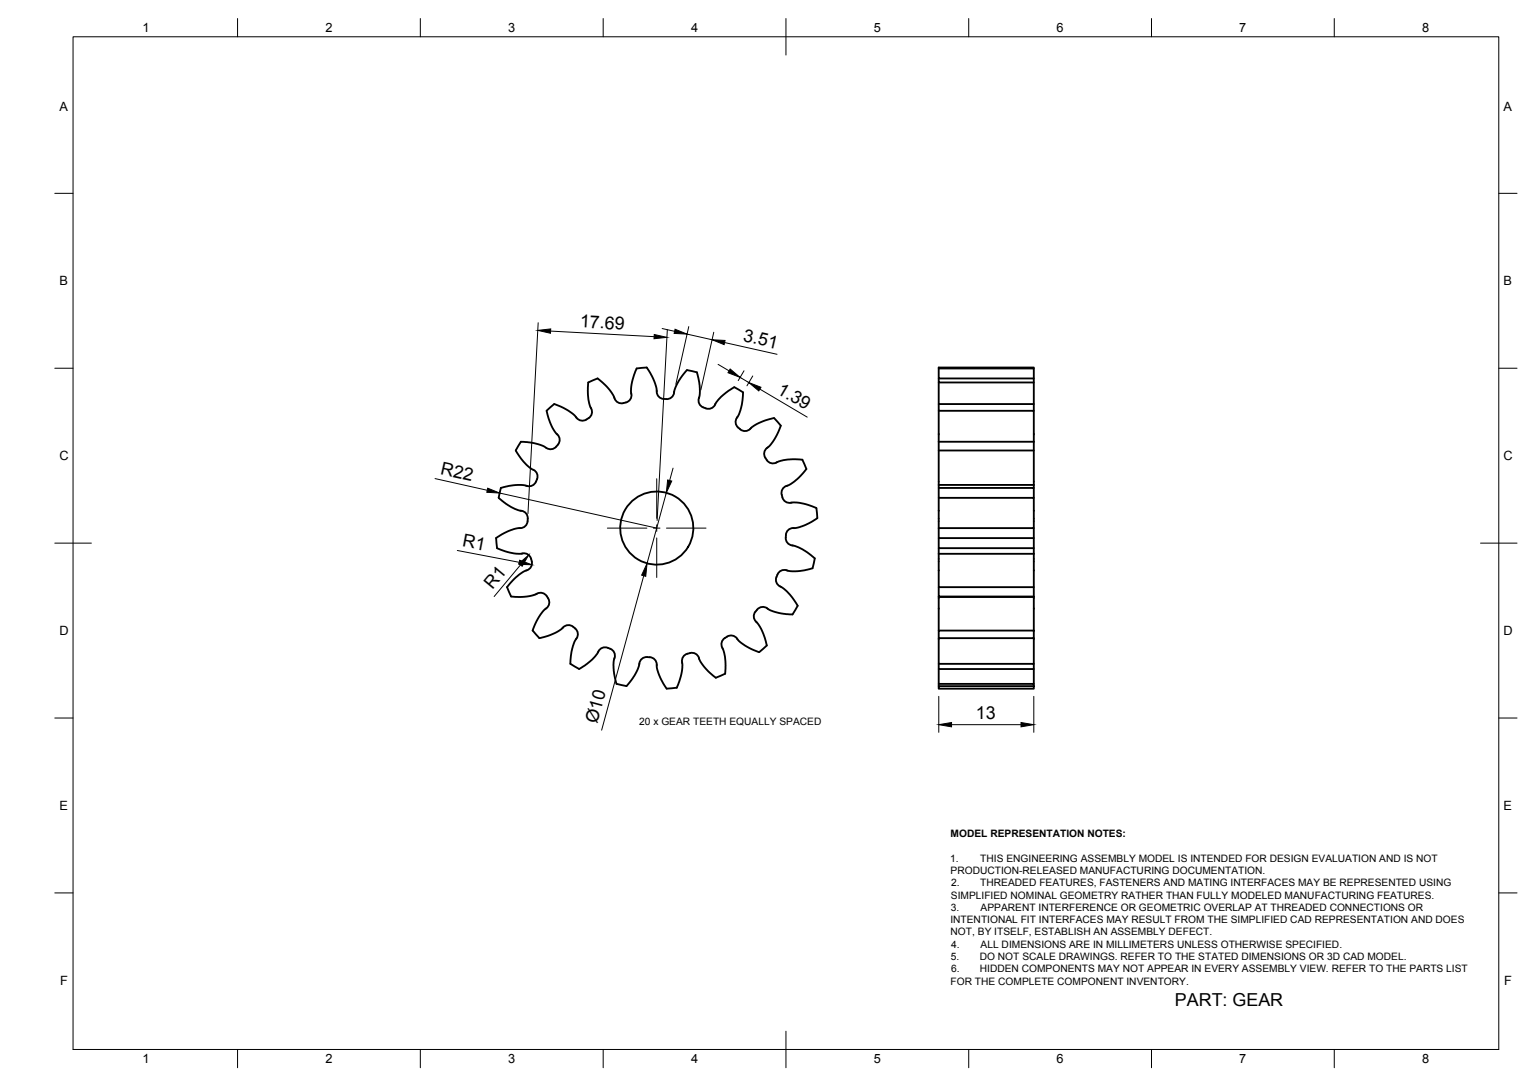
ISO-10303-21;
HEADER;
/* Generated by software containing ST-Developer
 * from STEP Tools, Inc. (www.steptools.com) 
 */

FILE_DESCRIPTION(
/* description */ (''),
/* implementation_level */ '2;1');

FILE_NAME(
/* name */ 'Gear.step',
/* time_stamp */ '2026-10-04T22:47:03-07:00',
/* author */ (''),
/* organization */ (''),
/* preprocessor_version */ 'ST-DEVELOPER v20.2',
/* originating_system */ 'Autodesk Translation Framework v15.15.0.0',
/* authorisation */ '');

FILE_SCHEMA (('AUTOMOTIVE_DESIGN { 1 0 10303 214 3 1 1 }'));
ENDSEC;

DATA;
#10=MECHANICAL_DESIGN_GEOMETRIC_PRESENTATION_REPRESENTATION('',(#77),#19878);
#63=SHAPE_REPRESENTATION_RELATIONSHIP('SRR','None',#19907,#70);
#70=ADVANCED_BREP_SHAPE_REPRESENTATION('',(#84),#19871);
#77=STYLED_ITEM('',(#19951),#84);
#84=MANIFOLD_SOLID_BREP('Body1',#4825);
#91=FACE_BOUND('',#736,.T.);
#92=FACE_BOUND('',#738,.T.);
#111=B_SPLINE_CURVE_WITH_KNOTS('',5,(#7546,#7547,#7548,#7549,#7550,#7551,
#7552,#7553,#7554,#7555,#7556,#7557,#7558,#7559,#7560,#7561,#7562,#7563,
#7564,#7565,#7566,#7567,#7568,#7569,#7570,#7571,#7572,#7573,#7574,#7575,
#7576,#7577,#7578,#7579,#7580,#7581,#7582,#7583,#7584,#7585,#7586,#7587,
#7588,#7589,#7590,#7591,#7592,#7593,#7594,#7595,#7596,#7597,#7598,#7599,
#7600,#7601,#7602,#7603,#7604,#7605,#7606,#7607,#7608,#7609,#7610,#7611,
#7612,#7613,#7614,#7615,#7616,#7617,#7618,#7619),.UNSPECIFIED.,.F.,.F.,
(6,1,1,1,1,1,1,1,1,1,1,1,1,1,1,1,1,1,1,1,1,1,1,1,1,1,1,1,1,1,1,1,1,1,1,
1,1,1,1,1,1,1,1,1,1,1,1,1,1,1,1,1,1,1,1,1,1,1,1,1,1,1,1,1,1,1,1,1,1,6),
(0.,0.0142857142857143,0.0285714285714286,0.0428571428571429,0.0571428571428571,
0.0714285714285714,0.0857142857142857,0.1,0.114285714285714,0.128571428571429,
0.142857142857143,0.157142857142857,0.171428571428571,0.185714285714286,
0.2,0.214285714285714,0.228571428571429,0.242857142857143,0.257142857142857,
0.271428571428571,0.285714285714286,0.3,0.314285714285714,0.328571428571429,
0.342857142857143,0.357142857142857,0.371428571428571,0.385714285714286,
0.4,0.414285714285714,0.428571428571429,0.442857142857143,0.457142857142857,
0.471428571428572,0.485714285714286,0.5,0.514285714285714,0.528571428571429,
0.542857142857143,0.557142857142857,0.571428571428571,0.585714285714286,
0.6,0.614285714285714,0.628571428571428,0.642857142857142,0.657142857142857,
0.671428571428571,0.685714285714285,0.699999999999999,0.714285714285714,
0.728571428571428,0.742857142857142,0.757142857142856,0.771428571428571,
0.785714285714285,0.799999999999999,0.814285714285713,0.828571428571428,
0.842857142857142,0.857142857142856,0.87142857142857,0.885714285714284,
0.899999999999999,0.914285714285713,0.928571428571427,0.942857142857141,
0.957142857142856,0.97142857142857,1.),.UNSPECIFIED.);
#112=B_SPLINE_CURVE_WITH_KNOTS('',3,(#7621,#7622,#7623,#7624,#7625,#7626,
#7627,#7628,#7629,#7630,#7631,#7632,#7633,#7634,#7635,#7636,#7637,#7638,
#7639,#7640,#7641,#7642,#7643,#7644,#7645,#7646,#7647,#7648,#7649,#7650,
#7651,#7652,#7653,#7654,#7655,#7656,#7657,#7658,#7659,#7660,#7661,#7662,
#7663,#7664,#7665,#7666,#7667,#7668,#7669,#7670,#7671,#7672,#7673,#7674,
#7675,#7676,#7677,#7678,#7679,#7680,#7681,#7682,#7683,#7684,#7685,#7686,
#7687),.UNSPECIFIED.,.F.,.F.,(4,3,3,3,3,3,3,3,3,3,3,3,3,3,3,3,3,3,3,3,3,
3,4),(-0.0308474254321917,-0.0282443140955979,-0.0239308458396743,-0.020615261220034,
-0.0170461143578005,-0.0150701375986627,-0.0131660090560162,-0.0115202579240142,
-0.0103391768048034,-0.00917732809651329,-0.00816993701567056,-0.00725747184422916,
-0.00648885937671962,-0.00537659348714137,-0.0047045193012487,-0.00408467783345363,
-0.00323202309358667,-0.00269108370723003,-0.00220561578671065,-0.00169529231611998,
-0.000847646158059989,-0.000380223899959456,0.),.UNSPECIFIED.);
#113=B_SPLINE_CURVE_WITH_KNOTS('',5,(#7845,#7846,#7847,#7848,#7849,#7850,
#7851,#7852,#7853,#7854,#7855,#7856,#7857,#7858,#7859,#7860,#7861,#7862,
#7863,#7864,#7865,#7866,#7867,#7868,#7869,#7870,#7871,#7872,#7873,#7874,
#7875,#7876,#7877,#7878,#7879,#7880,#7881,#7882,#7883,#7884,#7885,#7886,
#7887,#7888,#7889,#7890,#7891,#7892,#7893,#7894,#7895,#7896,#7897,#7898,
#7899,#7900,#7901,#7902,#7903,#7904,#7905,#7906,#7907,#7908,#7909,#7910,
#7911,#7912,#7913,#7914,#7915,#7916,#7917,#7918),.UNSPECIFIED.,.F.,.F.,
(6,1,1,1,1,1,1,1,1,1,1,1,1,1,1,1,1,1,1,1,1,1,1,1,1,1,1,1,1,1,1,1,1,1,1,
1,1,1,1,1,1,1,1,1,1,1,1,1,1,1,1,1,1,1,1,1,1,1,1,1,1,1,1,1,1,1,1,1,1,6),
(0.,0.0142857142857143,0.0285714285714286,0.0428571428571429,0.0571428571428571,
0.0714285714285714,0.0857142857142857,0.1,0.114285714285714,0.128571428571429,
0.142857142857143,0.157142857142857,0.171428571428571,0.185714285714286,
0.2,0.214285714285714,0.228571428571429,0.242857142857143,0.257142857142857,
0.271428571428571,0.285714285714286,0.3,0.314285714285714,0.328571428571429,
0.342857142857143,0.357142857142857,0.371428571428571,0.385714285714286,
0.4,0.414285714285714,0.428571428571429,0.442857142857143,0.457142857142857,
0.471428571428572,0.485714285714286,0.5,0.514285714285714,0.528571428571429,
0.542857142857143,0.557142857142857,0.571428571428571,0.585714285714286,
0.6,0.614285714285714,0.628571428571428,0.642857142857142,0.657142857142857,
0.671428571428571,0.685714285714285,0.699999999999999,0.714285714285714,
0.728571428571428,0.742857142857142,0.757142857142856,0.771428571428571,
0.785714285714285,0.799999999999999,0.814285714285713,0.828571428571428,
0.842857142857142,0.857142857142856,0.87142857142857,0.885714285714284,
0.899999999999999,0.914285714285713,0.928571428571427,0.942857142857141,
0.957142857142856,0.97142857142857,1.),.UNSPECIFIED.);
#114=B_SPLINE_CURVE_WITH_KNOTS('',3,(#7919,#7920,#7921,#7922,#7923,#7924,
#7925,#7926,#7927,#7928,#7929,#7930,#7931,#7932,#7933,#7934,#7935,#7936,
#7937,#7938,#7939,#7940,#7941,#7942,#7943,#7944,#7945,#7946,#7947,#7948,
#7949,#7950,#7951,#7952,#7953,#7954,#7955,#7956,#7957,#7958,#7959,#7960,
#7961,#7962,#7963,#7964,#7965,#7966,#7967,#7968,#7969,#7970,#7971,#7972,
#7973,#7974,#7975,#7976,#7977,#7978,#7979,#7980,#7981,#7982,#7983,#7984,
#7985,#7986,#7987,#7988),.UNSPECIFIED.,.F.,.F.,(4,3,3,3,3,3,3,3,3,3,3,3,
3,3,3,3,3,3,3,3,3,3,3,4),(-0.41144900970185,-0.405504895343942,-0.398537948713814,
-0.388735121356617,-0.382214695160452,-0.375350877738258,-0.367728232762158,
-0.356236725488341,-0.34788839668605,-0.33768327957583,-0.326660059396151,
-0.316483474305328,-0.302658060948649,-0.289316835657715,-0.271192407308052,
-0.255261428784221,-0.231775298718215,-0.202135573387617,-0.16198628027827,
-0.126192134079699,-0.0754619858625935,-0.0360560120089752,-0.00196686783518586,
0.),.UNSPECIFIED.);
#115=B_SPLINE_CURVE_WITH_KNOTS('',5,(#8140,#8141,#8142,#8143,#8144,#8145,
#8146,#8147,#8148,#8149,#8150,#8151,#8152,#8153,#8154,#8155,#8156,#8157,
#8158,#8159,#8160,#8161,#8162,#8163,#8164,#8165,#8166,#8167,#8168,#8169,
#8170,#8171,#8172,#8173,#8174,#8175,#8176,#8177,#8178,#8179,#8180,#8181,
#8182,#8183,#8184,#8185,#8186,#8187,#8188,#8189,#8190,#8191,#8192,#8193,
#8194,#8195,#8196,#8197,#8198,#8199,#8200,#8201,#8202,#8203,#8204,#8205,
#8206,#8207,#8208,#8209,#8210,#8211,#8212,#8213),.UNSPECIFIED.,.F.,.F.,
(6,1,1,1,1,1,1,1,1,1,1,1,1,1,1,1,1,1,1,1,1,1,1,1,1,1,1,1,1,1,1,1,1,1,1,
1,1,1,1,1,1,1,1,1,1,1,1,1,1,1,1,1,1,1,1,1,1,1,1,1,1,1,1,1,1,1,1,1,1,6),
(0.,0.0142857142857143,0.0285714285714286,0.0428571428571429,0.0571428571428571,
0.0714285714285714,0.0857142857142857,0.1,0.114285714285714,0.128571428571429,
0.142857142857143,0.157142857142857,0.171428571428571,0.185714285714286,
0.2,0.214285714285714,0.228571428571429,0.242857142857143,0.257142857142857,
0.271428571428571,0.285714285714286,0.3,0.314285714285714,0.328571428571429,
0.342857142857143,0.357142857142857,0.371428571428571,0.385714285714286,
0.4,0.414285714285714,0.428571428571429,0.442857142857143,0.457142857142857,
0.471428571428572,0.485714285714286,0.5,0.514285714285714,0.528571428571429,
0.542857142857143,0.557142857142857,0.571428571428571,0.585714285714286,
0.6,0.614285714285714,0.628571428571428,0.642857142857142,0.657142857142857,
0.671428571428571,0.685714285714285,0.699999999999999,0.714285714285714,
0.728571428571428,0.742857142857142,0.757142857142856,0.771428571428571,
0.785714285714285,0.799999999999999,0.814285714285713,0.828571428571428,
0.842857142857142,0.857142857142856,0.87142857142857,0.885714285714284,
0.899999999999999,0.914285714285713,0.928571428571427,0.942857142857141,
0.957142857142856,0.97142857142857,1.),.UNSPECIFIED.);
#116=B_SPLINE_CURVE_WITH_KNOTS('',3,(#8215,#8216,#8217,#8218,#8219,#8220,
#8221,#8222,#8223,#8224,#8225,#8226,#8227,#8228,#8229,#8230,#8231,#8232,
#8233,#8234,#8235,#8236,#8237,#8238,#8239,#8240,#8241,#8242,#8243,#8244,
#8245,#8246,#8247,#8248,#8249,#8250,#8251,#8252,#8253,#8254,#8255,#8256,
#8257,#8258,#8259,#8260,#8261,#8262,#8263,#8264,#8265,#8266,#8267,#8268,
#8269,#8270,#8271,#8272,#8273,#8274,#8275,#8276,#8277,#8278,#8279,#8280,
#8281),.UNSPECIFIED.,.F.,.F.,(4,3,3,3,3,3,3,3,3,3,3,3,3,3,3,3,3,3,3,3,3,
3,4),(-0.0308474253927552,-0.0282443143977923,-0.0239308462347147,-0.0206152615976367,
-0.017046114438784,-0.0150701378006816,-0.0131660089382207,-0.0115202578209431,
-0.0103391766998121,-0.00917732804029983,-0.00816993698852514,-0.00725747180050917,
-0.00648885933763945,-0.00537659350788907,-0.00470451931940294,-0.00408467785449232,
-0.00323202307997564,-0.00269108369563703,-0.00220561577615339,-0.00169529230461842,
-0.000847646152309211,-0.000380223895211713,0.),.UNSPECIFIED.);
#117=B_SPLINE_CURVE_WITH_KNOTS('',5,(#8439,#8440,#8441,#8442,#8443,#8444,
#8445,#8446,#8447,#8448,#8449,#8450,#8451,#8452,#8453,#8454,#8455,#8456,
#8457,#8458,#8459,#8460,#8461,#8462,#8463,#8464,#8465,#8466,#8467,#8468,
#8469,#8470,#8471,#8472,#8473,#8474,#8475,#8476,#8477,#8478,#8479,#8480,
#8481,#8482,#8483,#8484,#8485,#8486,#8487,#8488,#8489,#8490,#8491,#8492,
#8493,#8494,#8495,#8496,#8497,#8498,#8499,#8500,#8501,#8502,#8503,#8504,
#8505,#8506,#8507,#8508,#8509,#8510,#8511,#8512),.UNSPECIFIED.,.F.,.F.,
(6,1,1,1,1,1,1,1,1,1,1,1,1,1,1,1,1,1,1,1,1,1,1,1,1,1,1,1,1,1,1,1,1,1,1,
1,1,1,1,1,1,1,1,1,1,1,1,1,1,1,1,1,1,1,1,1,1,1,1,1,1,1,1,1,1,1,1,1,1,6),
(0.,0.0142857142857143,0.0285714285714286,0.0428571428571429,0.0571428571428571,
0.0714285714285714,0.0857142857142857,0.1,0.114285714285714,0.128571428571429,
0.142857142857143,0.157142857142857,0.171428571428571,0.185714285714286,
0.2,0.214285714285714,0.228571428571429,0.242857142857143,0.257142857142857,
0.271428571428571,0.285714285714286,0.3,0.314285714285714,0.328571428571429,
0.342857142857143,0.357142857142857,0.371428571428571,0.385714285714286,
0.4,0.414285714285714,0.428571428571429,0.442857142857143,0.457142857142857,
0.471428571428572,0.485714285714286,0.5,0.514285714285714,0.528571428571429,
0.542857142857143,0.557142857142857,0.571428571428571,0.585714285714286,
0.6,0.614285714285714,0.628571428571428,0.642857142857142,0.657142857142857,
0.671428571428571,0.685714285714285,0.699999999999999,0.714285714285714,
0.728571428571428,0.742857142857142,0.757142857142856,0.771428571428571,
0.785714285714285,0.799999999999999,0.814285714285713,0.828571428571428,
0.842857142857142,0.857142857142856,0.87142857142857,0.885714285714284,
0.899999999999999,0.914285714285713,0.928571428571427,0.942857142857141,
0.957142857142856,0.97142857142857,1.),.UNSPECIFIED.);
#118=B_SPLINE_CURVE_WITH_KNOTS('',3,(#8513,#8514,#8515,#8516,#8517,#8518,
#8519,#8520,#8521,#8522,#8523,#8524,#8525,#8526,#8527,#8528,#8529,#8530,
#8531,#8532,#8533,#8534,#8535,#8536,#8537,#8538,#8539,#8540,#8541,#8542,
#8543,#8544,#8545,#8546,#8547,#8548,#8549,#8550,#8551,#8552,#8553,#8554,
#8555,#8556,#8557,#8558,#8559,#8560,#8561,#8562,#8563,#8564,#8565,#8566,
#8567,#8568,#8569,#8570,#8571,#8572,#8573,#8574,#8575,#8576,#8577,#8578,
#8579,#8580,#8581,#8582,#8583,#8584,#8585,#8586,#8587,#8588),
 .UNSPECIFIED.,.F.,.F.,(4,3,3,3,3,3,3,3,3,3,3,3,3,3,3,3,3,3,3,3,3,3,3,3,
3,4),(-0.411449009835962,-0.403601796399829,-0.395573025581345,-0.386876504715203,
-0.375226575568619,-0.367043560841026,-0.358155681265519,-0.345047445919287,
-0.335636642409539,-0.325415895835815,-0.30690198526545,-0.293588015170367,
-0.286320302426775,-0.284969138437181,-0.283753083910261,-0.264146344834336,
-0.2466687814383,-0.228881898831898,-0.20935255979658,-0.188662818643314,
-0.1773046112729,-0.142988917240362,-0.110440538152722,-0.0644976592576526,
-0.0288887144369996,0.),.UNSPECIFIED.);
#119=B_SPLINE_CURVE_WITH_KNOTS('',5,(#8740,#8741,#8742,#8743,#8744,#8745,
#8746,#8747,#8748,#8749,#8750,#8751,#8752,#8753,#8754,#8755,#8756,#8757,
#8758,#8759,#8760,#8761,#8762,#8763,#8764,#8765,#8766,#8767,#8768,#8769,
#8770,#8771,#8772,#8773,#8774,#8775,#8776,#8777,#8778,#8779,#8780,#8781,
#8782,#8783,#8784,#8785,#8786,#8787,#8788,#8789,#8790,#8791,#8792,#8793,
#8794,#8795,#8796,#8797,#8798,#8799,#8800,#8801,#8802,#8803,#8804,#8805,
#8806,#8807,#8808,#8809,#8810,#8811,#8812,#8813),.UNSPECIFIED.,.F.,.F.,
(6,1,1,1,1,1,1,1,1,1,1,1,1,1,1,1,1,1,1,1,1,1,1,1,1,1,1,1,1,1,1,1,1,1,1,
1,1,1,1,1,1,1,1,1,1,1,1,1,1,1,1,1,1,1,1,1,1,1,1,1,1,1,1,1,1,1,1,1,1,6),
(0.,0.0142857142857143,0.0285714285714286,0.0428571428571429,0.0571428571428571,
0.0714285714285714,0.0857142857142857,0.1,0.114285714285714,0.128571428571429,
0.142857142857143,0.157142857142857,0.171428571428571,0.185714285714286,
0.2,0.214285714285714,0.228571428571429,0.242857142857143,0.257142857142857,
0.271428571428571,0.285714285714286,0.3,0.314285714285714,0.328571428571429,
0.342857142857143,0.357142857142857,0.371428571428571,0.385714285714286,
0.4,0.414285714285714,0.428571428571429,0.442857142857143,0.457142857142857,
0.471428571428572,0.485714285714286,0.5,0.514285714285714,0.528571428571429,
0.542857142857143,0.557142857142857,0.571428571428571,0.585714285714286,
0.6,0.614285714285714,0.628571428571428,0.642857142857142,0.657142857142857,
0.671428571428571,0.685714285714285,0.699999999999999,0.714285714285714,
0.728571428571428,0.742857142857142,0.757142857142856,0.771428571428571,
0.785714285714285,0.799999999999999,0.814285714285713,0.828571428571428,
0.842857142857142,0.857142857142856,0.87142857142857,0.885714285714284,
0.899999999999999,0.914285714285713,0.928571428571427,0.942857142857141,
0.957142857142856,0.97142857142857,1.),.UNSPECIFIED.);
#120=B_SPLINE_CURVE_WITH_KNOTS('',3,(#8815,#8816,#8817,#8818,#8819,#8820,
#8821,#8822,#8823,#8824,#8825,#8826,#8827,#8828,#8829,#8830,#8831,#8832,
#8833,#8834,#8835,#8836,#8837,#8838,#8839,#8840,#8841,#8842,#8843,#8844,
#8845,#8846,#8847,#8848,#8849,#8850,#8851,#8852,#8853,#8854,#8855,#8856,
#8857,#8858,#8859,#8860,#8861,#8862,#8863,#8864,#8865,#8866,#8867,#8868,
#8869,#8870,#8871,#8872,#8873,#8874,#8875,#8876,#8877,#8878,#8879,#8880,
#8881),.UNSPECIFIED.,.F.,.F.,(4,3,3,3,3,3,3,3,3,3,3,3,3,3,3,3,3,3,3,3,3,
3,4),(-0.0308474254458724,-0.0282443139325418,-0.0239308456237518,-0.0206152609798776,
-0.0170461143209945,-0.0150701375196663,-0.0131660090920878,-0.0115202579555768,
-0.0103391768402169,-0.00917732811491881,-0.00816993702510001,-0.00725747186261159,
-0.0064888593923997,-0.00537659347817632,-0.00470451929340428,-0.00408467782457058,
-0.0032320230991173,-0.00269108371201768,-0.00220561579110508,-0.00169529232104257,
-0.000847646160521286,-0.000380223902305551,0.),.UNSPECIFIED.);
#121=B_SPLINE_CURVE_WITH_KNOTS('',5,(#9039,#9040,#9041,#9042,#9043,#9044,
#9045,#9046,#9047,#9048,#9049,#9050,#9051,#9052,#9053,#9054,#9055,#9056,
#9057,#9058,#9059,#9060,#9061,#9062,#9063,#9064,#9065,#9066,#9067,#9068,
#9069,#9070,#9071,#9072,#9073,#9074,#9075,#9076,#9077,#9078,#9079,#9080,
#9081,#9082,#9083,#9084,#9085,#9086,#9087,#9088,#9089,#9090,#9091,#9092,
#9093,#9094,#9095,#9096,#9097,#9098,#9099,#9100,#9101,#9102,#9103,#9104,
#9105,#9106,#9107,#9108,#9109,#9110,#9111,#9112),.UNSPECIFIED.,.F.,.F.,
(6,1,1,1,1,1,1,1,1,1,1,1,1,1,1,1,1,1,1,1,1,1,1,1,1,1,1,1,1,1,1,1,1,1,1,
1,1,1,1,1,1,1,1,1,1,1,1,1,1,1,1,1,1,1,1,1,1,1,1,1,1,1,1,1,1,1,1,1,1,6),
(0.,0.0142857142857143,0.0285714285714286,0.0428571428571429,0.0571428571428571,
0.0714285714285714,0.0857142857142857,0.1,0.114285714285714,0.128571428571429,
0.142857142857143,0.157142857142857,0.171428571428571,0.185714285714286,
0.2,0.214285714285714,0.228571428571429,0.242857142857143,0.257142857142857,
0.271428571428571,0.285714285714286,0.3,0.314285714285714,0.328571428571429,
0.342857142857143,0.357142857142857,0.371428571428571,0.385714285714286,
0.4,0.414285714285714,0.428571428571429,0.442857142857143,0.457142857142857,
0.471428571428572,0.485714285714286,0.5,0.514285714285714,0.528571428571429,
0.542857142857143,0.557142857142857,0.571428571428571,0.585714285714286,
0.6,0.614285714285714,0.628571428571428,0.642857142857142,0.657142857142857,
0.671428571428571,0.685714285714285,0.699999999999999,0.714285714285714,
0.728571428571428,0.742857142857142,0.757142857142856,0.771428571428571,
0.785714285714285,0.799999999999999,0.814285714285713,0.828571428571428,
0.842857142857142,0.857142857142856,0.87142857142857,0.885714285714284,
0.899999999999999,0.914285714285713,0.928571428571427,0.942857142857141,
0.957142857142856,0.97142857142857,1.),.UNSPECIFIED.);
#122=B_SPLINE_CURVE_WITH_KNOTS('',3,(#9113,#9114,#9115,#9116,#9117,#9118,
#9119,#9120,#9121,#9122,#9123,#9124,#9125,#9126,#9127,#9128,#9129,#9130,
#9131,#9132,#9133,#9134,#9135,#9136,#9137,#9138,#9139,#9140,#9141,#9142,
#9143,#9144,#9145,#9146,#9147,#9148,#9149,#9150,#9151,#9152,#9153,#9154,
#9155,#9156,#9157,#9158,#9159,#9160,#9161,#9162,#9163,#9164,#9165,#9166,
#9167,#9168,#9169,#9170,#9171,#9172,#9173,#9174,#9175,#9176,#9177,#9178,
#9179,#9180,#9181,#9182),.UNSPECIFIED.,.F.,.F.,(4,3,3,3,3,3,3,3,3,3,3,3,
3,3,3,3,3,3,3,3,3,3,3,4),(-0.411449010058416,-0.405504895678982,-0.398537949040723,
-0.388735121700349,-0.382214695498563,-0.375350878070222,-0.367728233088589,
-0.356236725804571,-0.347888396993553,-0.337683279874044,-0.326660059681915,
-0.316483474587148,-0.302658061236691,-0.289316835946338,-0.271192407689148,
-0.25526142925369,-0.231775299041798,-0.202135573687089,-0.161986280481546,
-0.126192134078593,-0.075461985765785,-0.0360560137735561,-0.00196687385551187,
0.),.UNSPECIFIED.);
#123=B_SPLINE_CURVE_WITH_KNOTS('',5,(#9334,#9335,#9336,#9337,#9338,#9339,
#9340,#9341,#9342,#9343,#9344,#9345,#9346,#9347,#9348,#9349,#9350,#9351,
#9352,#9353,#9354,#9355,#9356,#9357,#9358,#9359,#9360,#9361,#9362,#9363,
#9364,#9365,#9366,#9367,#9368,#9369,#9370,#9371,#9372,#9373,#9374,#9375,
#9376,#9377,#9378,#9379,#9380,#9381,#9382,#9383,#9384,#9385,#9386,#9387,
#9388,#9389,#9390,#9391,#9392,#9393,#9394,#9395,#9396,#9397,#9398,#9399,
#9400,#9401,#9402,#9403,#9404,#9405,#9406,#9407),.UNSPECIFIED.,.F.,.F.,
(6,1,1,1,1,1,1,1,1,1,1,1,1,1,1,1,1,1,1,1,1,1,1,1,1,1,1,1,1,1,1,1,1,1,1,
1,1,1,1,1,1,1,1,1,1,1,1,1,1,1,1,1,1,1,1,1,1,1,1,1,1,1,1,1,1,1,1,1,1,6),
(0.,0.0142857142857143,0.0285714285714286,0.0428571428571429,0.0571428571428571,
0.0714285714285714,0.0857142857142857,0.1,0.114285714285714,0.128571428571429,
0.142857142857143,0.157142857142857,0.171428571428571,0.185714285714286,
0.2,0.214285714285714,0.228571428571429,0.242857142857143,0.257142857142857,
0.271428571428571,0.285714285714286,0.3,0.314285714285714,0.328571428571429,
0.342857142857143,0.357142857142857,0.371428571428571,0.385714285714286,
0.4,0.414285714285714,0.428571428571429,0.442857142857143,0.457142857142857,
0.471428571428572,0.485714285714286,0.5,0.514285714285714,0.528571428571429,
0.542857142857143,0.557142857142857,0.571428571428571,0.585714285714286,
0.6,0.614285714285714,0.628571428571428,0.642857142857142,0.657142857142857,
0.671428571428571,0.685714285714285,0.699999999999999,0.714285714285714,
0.728571428571428,0.742857142857142,0.757142857142856,0.771428571428571,
0.785714285714285,0.799999999999999,0.814285714285713,0.828571428571428,
0.842857142857142,0.857142857142856,0.87142857142857,0.885714285714284,
0.899999999999999,0.914285714285713,0.928571428571427,0.942857142857141,
0.957142857142856,0.97142857142857,1.),.UNSPECIFIED.);
#124=B_SPLINE_CURVE_WITH_KNOTS('',3,(#9409,#9410,#9411,#9412,#9413,#9414,
#9415,#9416,#9417,#9418,#9419,#9420,#9421,#9422,#9423,#9424,#9425,#9426,
#9427,#9428,#9429,#9430,#9431,#9432,#9433,#9434,#9435,#9436,#9437,#9438,
#9439,#9440,#9441,#9442,#9443,#9444,#9445,#9446,#9447,#9448,#9449,#9450,
#9451,#9452,#9453,#9454,#9455,#9456,#9457,#9458,#9459,#9460,#9461,#9462,
#9463,#9464,#9465,#9466,#9467,#9468,#9469,#9470,#9471,#9472,#9473,#9474,
#9475),.UNSPECIFIED.,.F.,.F.,(4,3,3,3,3,3,3,3,3,3,3,3,3,3,3,3,3,3,3,3,3,
3,4),(-0.0308474254450083,-0.0282443143076938,-0.0239308461003898,-0.0206152614713912,
-0.0170461144298779,-0.0150701377273182,-0.0131660090093565,-0.0115202578831869,
-0.0103391767614099,-0.00917732807782989,-0.00816993701064961,-0.00725747183277268,
-0.00648885936633748,-0.00537659350089532,-0.00470451931328341,-0.00408467784616126,
-0.00323202309082144,-0.00269108370483176,-0.00220561578430491,-0.0016952923129278,
-0.000847646156463901,-0.000380223898998028,0.),.UNSPECIFIED.);
#125=B_SPLINE_CURVE_WITH_KNOTS('',5,(#9633,#9634,#9635,#9636,#9637,#9638,
#9639,#9640,#9641,#9642,#9643,#9644,#9645,#9646,#9647,#9648,#9649,#9650,
#9651,#9652,#9653,#9654,#9655,#9656,#9657,#9658,#9659,#9660,#9661,#9662,
#9663,#9664,#9665,#9666,#9667,#9668,#9669,#9670,#9671,#9672,#9673,#9674,
#9675,#9676,#9677,#9678,#9679,#9680,#9681,#9682,#9683,#9684,#9685,#9686,
#9687,#9688,#9689,#9690,#9691,#9692,#9693,#9694,#9695,#9696,#9697,#9698,
#9699,#9700,#9701,#9702,#9703,#9704,#9705,#9706),.UNSPECIFIED.,.F.,.F.,
(6,1,1,1,1,1,1,1,1,1,1,1,1,1,1,1,1,1,1,1,1,1,1,1,1,1,1,1,1,1,1,1,1,1,1,
1,1,1,1,1,1,1,1,1,1,1,1,1,1,1,1,1,1,1,1,1,1,1,1,1,1,1,1,1,1,1,1,1,1,6),
(0.,0.0142857142857143,0.0285714285714286,0.0428571428571429,0.0571428571428571,
0.0714285714285714,0.0857142857142857,0.1,0.114285714285714,0.128571428571429,
0.142857142857143,0.157142857142857,0.171428571428571,0.185714285714286,
0.2,0.214285714285714,0.228571428571429,0.242857142857143,0.257142857142857,
0.271428571428571,0.285714285714286,0.3,0.314285714285714,0.328571428571429,
0.342857142857143,0.357142857142857,0.371428571428571,0.385714285714286,
0.4,0.414285714285714,0.428571428571429,0.442857142857143,0.457142857142857,
0.471428571428572,0.485714285714286,0.5,0.514285714285714,0.528571428571429,
0.542857142857143,0.557142857142857,0.571428571428571,0.585714285714286,
0.6,0.614285714285714,0.628571428571428,0.642857142857142,0.657142857142857,
0.671428571428571,0.685714285714285,0.699999999999999,0.714285714285714,
0.728571428571428,0.742857142857142,0.757142857142856,0.771428571428571,
0.785714285714285,0.799999999999999,0.814285714285713,0.828571428571428,
0.842857142857142,0.857142857142856,0.87142857142857,0.885714285714284,
0.899999999999999,0.914285714285713,0.928571428571427,0.942857142857141,
0.957142857142856,0.97142857142857,1.),.UNSPECIFIED.);
#126=B_SPLINE_CURVE_WITH_KNOTS('',3,(#9707,#9708,#9709,#9710,#9711,#9712,
#9713,#9714,#9715,#9716,#9717,#9718,#9719,#9720,#9721,#9722,#9723,#9724,
#9725,#9726,#9727,#9728,#9729,#9730,#9731,#9732,#9733,#9734,#9735,#9736,
#9737,#9738,#9739,#9740,#9741,#9742,#9743,#9744,#9745,#9746,#9747,#9748,
#9749,#9750,#9751,#9752,#9753,#9754,#9755,#9756,#9757,#9758,#9759,#9760,
#9761,#9762,#9763,#9764,#9765,#9766,#9767,#9768,#9769,#9770,#9771,#9772,
#9773,#9774,#9775,#9776),.UNSPECIFIED.,.F.,.F.,(4,3,3,3,3,3,3,3,3,3,3,3,
3,3,3,3,3,3,3,3,3,3,3,4),(-0.411449009990747,-0.405504895608626,-0.398537948969837,
-0.388735121635006,-0.38221469543425,-0.375350878008265,-0.367728233026823,
-0.356236725744735,-0.347888396935362,-0.337683279819759,-0.326660059629232,
-0.31648347453161,-0.302658061144547,-0.289316835829758,-0.271192407431711,
-0.255261428895363,-0.2317752988163,-0.202135573454307,-0.16198628027259,
-0.126192133914446,-0.0754619856962401,-0.0360560096209726,-0.00196686147092064,
0.),.UNSPECIFIED.);
#127=B_SPLINE_CURVE_WITH_KNOTS('',5,(#9928,#9929,#9930,#9931,#9932,#9933,
#9934,#9935,#9936,#9937,#9938,#9939,#9940,#9941,#9942,#9943,#9944,#9945,
#9946,#9947,#9948,#9949,#9950,#9951,#9952,#9953,#9954,#9955,#9956,#9957,
#9958,#9959,#9960,#9961,#9962,#9963,#9964,#9965,#9966,#9967,#9968,#9969,
#9970,#9971,#9972,#9973,#9974,#9975,#9976,#9977,#9978,#9979,#9980,#9981,
#9982,#9983,#9984,#9985,#9986,#9987,#9988,#9989,#9990,#9991,#9992,#9993,
#9994,#9995,#9996,#9997,#9998,#9999,#10000,#10001),.UNSPECIFIED.,.F.,.F.,
(6,1,1,1,1,1,1,1,1,1,1,1,1,1,1,1,1,1,1,1,1,1,1,1,1,1,1,1,1,1,1,1,1,1,1,
1,1,1,1,1,1,1,1,1,1,1,1,1,1,1,1,1,1,1,1,1,1,1,1,1,1,1,1,1,1,1,1,1,1,6),
(0.,0.0142857142857143,0.0285714285714286,0.0428571428571429,0.0571428571428571,
0.0714285714285714,0.0857142857142857,0.1,0.114285714285714,0.128571428571429,
0.142857142857143,0.157142857142857,0.171428571428571,0.185714285714286,
0.2,0.214285714285714,0.228571428571429,0.242857142857143,0.257142857142857,
0.271428571428571,0.285714285714286,0.3,0.314285714285714,0.328571428571429,
0.342857142857143,0.357142857142857,0.371428571428571,0.385714285714286,
0.4,0.414285714285714,0.428571428571429,0.442857142857143,0.457142857142857,
0.471428571428572,0.485714285714286,0.5,0.514285714285714,0.528571428571429,
0.542857142857143,0.557142857142857,0.571428571428571,0.585714285714286,
0.6,0.614285714285714,0.628571428571428,0.642857142857142,0.657142857142857,
0.671428571428571,0.685714285714285,0.699999999999999,0.714285714285714,
0.728571428571428,0.742857142857142,0.757142857142856,0.771428571428571,
0.785714285714285,0.799999999999999,0.814285714285713,0.828571428571428,
0.842857142857142,0.857142857142856,0.87142857142857,0.885714285714284,
0.899999999999999,0.914285714285713,0.928571428571427,0.942857142857141,
0.957142857142856,0.97142857142857,1.),.UNSPECIFIED.);
#128=B_SPLINE_CURVE_WITH_KNOTS('',3,(#10003,#10004,#10005,#10006,#10007,
#10008,#10009,#10010,#10011,#10012,#10013,#10014,#10015,#10016,#10017,#10018,
#10019,#10020,#10021,#10022,#10023,#10024,#10025,#10026,#10027,#10028,#10029,
#10030,#10031,#10032,#10033,#10034,#10035,#10036,#10037,#10038,#10039,#10040,
#10041,#10042,#10043,#10044,#10045,#10046,#10047,#10048,#10049,#10050,#10051,
#10052,#10053,#10054,#10055,#10056,#10057,#10058,#10059,#10060,#10061,#10062,
#10063,#10064,#10065,#10066,#10067,#10068,#10069),.UNSPECIFIED.,.F.,.F.,
(4,3,3,3,3,3,3,3,3,3,3,3,3,3,3,3,3,3,3,3,3,3,4),(-0.0308474254187031,-0.028244314224116,
-0.0239308459820195,-0.020615261356278,-0.0170461143857998,-0.0150701376654228,
-0.0131660090191134,-0.0115202578917242,-0.0103391767722299,-0.00917732807803008,
-0.00816993700645051,-0.00725747183186186,-0.00648885936554755,-0.00537659349257577,
-0.0047045193060038,-0.00408467783901597,-0.00323202308941783,-0.00269108370365142,
-0.00220561578349396,-0.00169529231275093,-0.000847646156375465,-0.000380223898800284,
0.),.UNSPECIFIED.);
#129=B_SPLINE_CURVE_WITH_KNOTS('',5,(#10227,#10228,#10229,#10230,#10231,
#10232,#10233,#10234,#10235,#10236,#10237,#10238,#10239,#10240,#10241,#10242,
#10243,#10244,#10245,#10246,#10247,#10248,#10249,#10250,#10251,#10252,#10253,
#10254,#10255,#10256,#10257,#10258,#10259,#10260,#10261,#10262,#10263,#10264,
#10265,#10266,#10267,#10268,#10269,#10270,#10271,#10272,#10273,#10274,#10275,
#10276,#10277,#10278,#10279,#10280,#10281,#10282,#10283,#10284,#10285,#10286,
#10287,#10288,#10289,#10290,#10291,#10292,#10293,#10294,#10295,#10296,#10297,
#10298,#10299,#10300),.UNSPECIFIED.,.F.,.F.,(6,1,1,1,1,1,1,1,1,1,1,1,1,
1,1,1,1,1,1,1,1,1,1,1,1,1,1,1,1,1,1,1,1,1,1,1,1,1,1,1,1,1,1,1,1,1,1,1,1,
1,1,1,1,1,1,1,1,1,1,1,1,1,1,1,1,1,1,1,1,6),(0.,0.0142857142857143,0.0285714285714286,
0.0428571428571429,0.0571428571428571,0.0714285714285714,0.0857142857142857,
0.1,0.114285714285714,0.128571428571429,0.142857142857143,0.157142857142857,
0.171428571428571,0.185714285714286,0.2,0.214285714285714,0.228571428571429,
0.242857142857143,0.257142857142857,0.271428571428571,0.285714285714286,
0.3,0.314285714285714,0.328571428571429,0.342857142857143,0.357142857142857,
0.371428571428571,0.385714285714286,0.4,0.414285714285714,0.428571428571429,
0.442857142857143,0.457142857142857,0.471428571428572,0.485714285714286,
0.5,0.514285714285714,0.528571428571429,0.542857142857143,0.557142857142857,
0.571428571428571,0.585714285714286,0.6,0.614285714285714,0.628571428571428,
0.642857142857142,0.657142857142857,0.671428571428571,0.685714285714285,
0.699999999999999,0.714285714285714,0.728571428571428,0.742857142857142,
0.757142857142856,0.771428571428571,0.785714285714285,0.799999999999999,
0.814285714285713,0.828571428571428,0.842857142857142,0.857142857142856,
0.87142857142857,0.885714285714284,0.899999999999999,0.914285714285713,
0.928571428571427,0.942857142857141,0.957142857142856,0.97142857142857,
1.),.UNSPECIFIED.);
#130=B_SPLINE_CURVE_WITH_KNOTS('',3,(#10301,#10302,#10303,#10304,#10305,
#10306,#10307,#10308,#10309,#10310,#10311,#10312,#10313,#10314,#10315,#10316,
#10317,#10318,#10319,#10320,#10321,#10322,#10323,#10324,#10325,#10326,#10327,
#10328,#10329,#10330,#10331,#10332,#10333,#10334,#10335,#10336,#10337,#10338,
#10339,#10340,#10341,#10342,#10343,#10344,#10345,#10346,#10347,#10348,#10349,
#10350,#10351,#10352,#10353,#10354,#10355,#10356,#10357,#10358,#10359,#10360,
#10361,#10362,#10363,#10364,#10365,#10366,#10367,#10368,#10369,#10370),
 .UNSPECIFIED.,.F.,.F.,(4,3,3,3,3,3,3,3,3,3,3,3,3,3,3,3,3,3,3,3,3,3,3,4),
(-0.411449009784292,-0.405504895410621,-0.398537948775868,-0.388735121437593,
-0.382214695240303,-0.375350877816651,-0.367728232839072,-0.356236725562851,
-0.347888396756906,-0.33768327964519,-0.326660059462181,-0.31648347436891,
-0.302658061000279,-0.289316835703338,-0.271192407317085,-0.255261428783421,
-0.231775298711656,-0.20213557335682,-0.161986280248108,-0.126192134001441,
-0.0754619855590316,-0.036056011065119,-0.00196686534552455,0.),
 .UNSPECIFIED.);
#131=B_SPLINE_CURVE_WITH_KNOTS('',5,(#10522,#10523,#10524,#10525,#10526,
#10527,#10528,#10529,#10530,#10531,#10532,#10533,#10534,#10535,#10536,#10537,
#10538,#10539,#10540,#10541,#10542,#10543,#10544,#10545,#10546,#10547,#10548,
#10549,#10550,#10551,#10552,#10553,#10554,#10555,#10556,#10557,#10558,#10559,
#10560,#10561,#10562,#10563,#10564,#10565,#10566,#10567,#10568,#10569,#10570,
#10571,#10572,#10573,#10574,#10575,#10576,#10577,#10578,#10579,#10580,#10581,
#10582,#10583,#10584,#10585,#10586,#10587,#10588,#10589,#10590,#10591,#10592,
#10593,#10594,#10595),.UNSPECIFIED.,.F.,.F.,(6,1,1,1,1,1,1,1,1,1,1,1,1,
1,1,1,1,1,1,1,1,1,1,1,1,1,1,1,1,1,1,1,1,1,1,1,1,1,1,1,1,1,1,1,1,1,1,1,1,
1,1,1,1,1,1,1,1,1,1,1,1,1,1,1,1,1,1,1,1,6),(0.,0.0142857142857143,0.0285714285714286,
0.0428571428571429,0.0571428571428571,0.0714285714285714,0.0857142857142857,
0.1,0.114285714285714,0.128571428571429,0.142857142857143,0.157142857142857,
0.171428571428571,0.185714285714286,0.2,0.214285714285714,0.228571428571429,
0.242857142857143,0.257142857142857,0.271428571428571,0.285714285714286,
0.3,0.314285714285714,0.328571428571429,0.342857142857143,0.357142857142857,
0.371428571428571,0.385714285714286,0.4,0.414285714285714,0.428571428571429,
0.442857142857143,0.457142857142857,0.471428571428572,0.485714285714286,
0.5,0.514285714285714,0.528571428571429,0.542857142857143,0.557142857142857,
0.571428571428571,0.585714285714286,0.6,0.614285714285714,0.628571428571428,
0.642857142857142,0.657142857142857,0.671428571428571,0.685714285714285,
0.699999999999999,0.714285714285714,0.728571428571428,0.742857142857142,
0.757142857142856,0.771428571428571,0.785714285714285,0.799999999999999,
0.814285714285713,0.828571428571428,0.842857142857142,0.857142857142856,
0.87142857142857,0.885714285714284,0.899999999999999,0.914285714285713,
0.928571428571427,0.942857142857141,0.957142857142856,0.97142857142857,
1.),.UNSPECIFIED.);
#132=B_SPLINE_CURVE_WITH_KNOTS('',3,(#10597,#10598,#10599,#10600,#10601,
#10602,#10603,#10604,#10605,#10606,#10607,#10608,#10609,#10610,#10611,#10612,
#10613,#10614,#10615,#10616,#10617,#10618,#10619,#10620,#10621,#10622,#10623,
#10624,#10625,#10626,#10627,#10628,#10629,#10630,#10631,#10632,#10633,#10634,
#10635,#10636,#10637,#10638,#10639,#10640,#10641,#10642,#10643,#10644,#10645,
#10646,#10647,#10648,#10649,#10650,#10651,#10652,#10653,#10654,#10655,#10656,
#10657,#10658,#10659,#10660,#10661,#10662,#10663),.UNSPECIFIED.,.F.,.F.,
(4,3,3,3,3,3,3,3,3,3,3,3,3,3,3,3,3,3,3,3,3,3,4),(-0.0308474254321917,-0.0282443140955979,
-0.0239308458396743,-0.020615261220034,-0.0170461143578005,-0.0150701375986627,
-0.0131660090560162,-0.0115202579240142,-0.0103391768048034,-0.00917732809651329,
-0.00816993701567056,-0.00725747184422916,-0.00648885937671962,-0.00537659348714137,
-0.0047045193012487,-0.00408467783345363,-0.00323202309358667,-0.00269108370723003,
-0.00220561578671065,-0.00169529231611998,-0.000847646158059989,-0.000380223899959456,
0.),.UNSPECIFIED.);
#133=B_SPLINE_CURVE_WITH_KNOTS('',5,(#10821,#10822,#10823,#10824,#10825,
#10826,#10827,#10828,#10829,#10830,#10831,#10832,#10833,#10834,#10835,#10836,
#10837,#10838,#10839,#10840,#10841,#10842,#10843,#10844,#10845,#10846,#10847,
#10848,#10849,#10850,#10851,#10852,#10853,#10854,#10855,#10856,#10857,#10858,
#10859,#10860,#10861,#10862,#10863,#10864,#10865,#10866,#10867,#10868,#10869,
#10870,#10871,#10872,#10873,#10874,#10875,#10876,#10877,#10878,#10879,#10880,
#10881,#10882,#10883,#10884,#10885,#10886,#10887,#10888,#10889,#10890,#10891,
#10892,#10893,#10894),.UNSPECIFIED.,.F.,.F.,(6,1,1,1,1,1,1,1,1,1,1,1,1,
1,1,1,1,1,1,1,1,1,1,1,1,1,1,1,1,1,1,1,1,1,1,1,1,1,1,1,1,1,1,1,1,1,1,1,1,
1,1,1,1,1,1,1,1,1,1,1,1,1,1,1,1,1,1,1,1,6),(0.,0.0142857142857143,0.0285714285714286,
0.0428571428571429,0.0571428571428571,0.0714285714285714,0.0857142857142857,
0.1,0.114285714285714,0.128571428571429,0.142857142857143,0.157142857142857,
0.171428571428571,0.185714285714286,0.2,0.214285714285714,0.228571428571429,
0.242857142857143,0.257142857142857,0.271428571428571,0.285714285714286,
0.3,0.314285714285714,0.328571428571429,0.342857142857143,0.357142857142857,
0.371428571428571,0.385714285714286,0.4,0.414285714285714,0.428571428571429,
0.442857142857143,0.457142857142857,0.471428571428572,0.485714285714286,
0.5,0.514285714285714,0.528571428571429,0.542857142857143,0.557142857142857,
0.571428571428571,0.585714285714286,0.6,0.614285714285714,0.628571428571428,
0.642857142857142,0.657142857142857,0.671428571428571,0.685714285714285,
0.699999999999999,0.714285714285714,0.728571428571428,0.742857142857142,
0.757142857142856,0.771428571428571,0.785714285714285,0.799999999999999,
0.814285714285713,0.828571428571428,0.842857142857142,0.857142857142856,
0.87142857142857,0.885714285714284,0.899999999999999,0.914285714285713,
0.928571428571427,0.942857142857141,0.957142857142856,0.97142857142857,
1.),.UNSPECIFIED.);
#134=B_SPLINE_CURVE_WITH_KNOTS('',3,(#10895,#10896,#10897,#10898,#10899,
#10900,#10901,#10902,#10903,#10904,#10905,#10906,#10907,#10908,#10909,#10910,
#10911,#10912,#10913,#10914,#10915,#10916,#10917,#10918,#10919,#10920,#10921,
#10922,#10923,#10924,#10925,#10926,#10927,#10928,#10929,#10930,#10931,#10932,
#10933,#10934,#10935,#10936,#10937,#10938,#10939,#10940,#10941,#10942,#10943,
#10944,#10945,#10946,#10947,#10948,#10949,#10950,#10951,#10952,#10953,#10954,
#10955,#10956,#10957,#10958,#10959,#10960,#10961,#10962,#10963,#10964),
 .UNSPECIFIED.,.F.,.F.,(4,3,3,3,3,3,3,3,3,3,3,3,3,3,3,3,3,3,3,3,3,3,3,4),
(-0.41144900970185,-0.405504895343942,-0.398537948713814,-0.388735121356617,
-0.382214695160452,-0.375350877738258,-0.367728232762158,-0.356236725488341,
-0.34788839668605,-0.33768327957583,-0.326660059396151,-0.316483474305328,
-0.302658060948649,-0.289316835657715,-0.271192407308052,-0.255261428784221,
-0.231775298718215,-0.202135573387617,-0.16198628027827,-0.126192134079699,
-0.0754619858625935,-0.0360560120089752,-0.00196686783518586,0.),
 .UNSPECIFIED.);
#135=B_SPLINE_CURVE_WITH_KNOTS('',5,(#11116,#11117,#11118,#11119,#11120,
#11121,#11122,#11123,#11124,#11125,#11126,#11127,#11128,#11129,#11130,#11131,
#11132,#11133,#11134,#11135,#11136,#11137,#11138,#11139,#11140,#11141,#11142,
#11143,#11144,#11145,#11146,#11147,#11148,#11149,#11150,#11151,#11152,#11153,
#11154,#11155,#11156,#11157,#11158,#11159,#11160,#11161,#11162,#11163,#11164,
#11165,#11166,#11167,#11168,#11169,#11170,#11171,#11172,#11173,#11174,#11175,
#11176,#11177,#11178,#11179,#11180,#11181,#11182,#11183,#11184,#11185,#11186,
#11187,#11188,#11189),.UNSPECIFIED.,.F.,.F.,(6,1,1,1,1,1,1,1,1,1,1,1,1,
1,1,1,1,1,1,1,1,1,1,1,1,1,1,1,1,1,1,1,1,1,1,1,1,1,1,1,1,1,1,1,1,1,1,1,1,
1,1,1,1,1,1,1,1,1,1,1,1,1,1,1,1,1,1,1,1,6),(0.,0.0142857142857143,0.0285714285714286,
0.0428571428571429,0.0571428571428571,0.0714285714285714,0.0857142857142857,
0.1,0.114285714285714,0.128571428571429,0.142857142857143,0.157142857142857,
0.171428571428571,0.185714285714286,0.2,0.214285714285714,0.228571428571429,
0.242857142857143,0.257142857142857,0.271428571428571,0.285714285714286,
0.3,0.314285714285714,0.328571428571429,0.342857142857143,0.357142857142857,
0.371428571428571,0.385714285714286,0.4,0.414285714285714,0.428571428571429,
0.442857142857143,0.457142857142857,0.471428571428572,0.485714285714286,
0.5,0.514285714285714,0.528571428571429,0.542857142857143,0.557142857142857,
0.571428571428571,0.585714285714286,0.6,0.614285714285714,0.628571428571428,
0.642857142857142,0.657142857142857,0.671428571428571,0.685714285714285,
0.699999999999999,0.714285714285714,0.728571428571428,0.742857142857142,
0.757142857142856,0.771428571428571,0.785714285714285,0.799999999999999,
0.814285714285713,0.828571428571428,0.842857142857142,0.857142857142856,
0.87142857142857,0.885714285714284,0.899999999999999,0.914285714285713,
0.928571428571427,0.942857142857141,0.957142857142856,0.97142857142857,
1.),.UNSPECIFIED.);
#136=B_SPLINE_CURVE_WITH_KNOTS('',3,(#11191,#11192,#11193,#11194,#11195,
#11196,#11197,#11198,#11199,#11200,#11201,#11202,#11203,#11204,#11205,#11206,
#11207,#11208,#11209,#11210,#11211,#11212,#11213,#11214,#11215,#11216,#11217,
#11218,#11219,#11220,#11221,#11222,#11223,#11224,#11225,#11226,#11227,#11228,
#11229,#11230,#11231,#11232,#11233,#11234,#11235,#11236,#11237,#11238,#11239,
#11240,#11241,#11242,#11243,#11244,#11245,#11246,#11247,#11248,#11249,#11250,
#11251,#11252,#11253,#11254,#11255,#11256,#11257),.UNSPECIFIED.,.F.,.F.,
(4,3,3,3,3,3,3,3,3,3,3,3,3,3,3,3,3,3,3,3,3,3,4),(-0.0308474254313729,-0.0282443144331512,
-0.0239308462436385,-0.0206152616062002,-0.017046114491142,-0.0150701378789916,
-0.0131660089309141,-0.0115202578145499,-0.0103391766904584,-0.0091773280428693,
-0.00816993699591886,-0.00725747180427489,-0.00648885934148822,-0.00537659351838039,
-0.00470451932858284,-0.00408467786302119,-0.00323202308259216,-0.00269108369773592,
-0.00220561577775678,-0.00169529230541892,-0.00084764615270946,-0.000380223895080282,
0.),.UNSPECIFIED.);
#137=B_SPLINE_CURVE_WITH_KNOTS('',5,(#11415,#11416,#11417,#11418,#11419,
#11420,#11421,#11422,#11423,#11424,#11425,#11426,#11427,#11428,#11429,#11430,
#11431,#11432,#11433,#11434,#11435,#11436,#11437,#11438,#11439,#11440,#11441,
#11442,#11443,#11444,#11445,#11446,#11447,#11448,#11449,#11450,#11451,#11452,
#11453,#11454,#11455,#11456,#11457,#11458,#11459,#11460,#11461,#11462,#11463,
#11464,#11465,#11466,#11467,#11468,#11469,#11470,#11471,#11472,#11473,#11474,
#11475,#11476,#11477,#11478,#11479,#11480,#11481,#11482,#11483,#11484,#11485,
#11486,#11487,#11488),.UNSPECIFIED.,.F.,.F.,(6,1,1,1,1,1,1,1,1,1,1,1,1,
1,1,1,1,1,1,1,1,1,1,1,1,1,1,1,1,1,1,1,1,1,1,1,1,1,1,1,1,1,1,1,1,1,1,1,1,
1,1,1,1,1,1,1,1,1,1,1,1,1,1,1,1,1,1,1,1,6),(0.,0.0142857142857143,0.0285714285714286,
0.0428571428571429,0.0571428571428571,0.0714285714285714,0.0857142857142857,
0.1,0.114285714285714,0.128571428571429,0.142857142857143,0.157142857142857,
0.171428571428571,0.185714285714286,0.2,0.214285714285714,0.228571428571429,
0.242857142857143,0.257142857142857,0.271428571428571,0.285714285714286,
0.3,0.314285714285714,0.328571428571429,0.342857142857143,0.357142857142857,
0.371428571428571,0.385714285714286,0.4,0.414285714285714,0.428571428571429,
0.442857142857143,0.457142857142857,0.471428571428572,0.485714285714286,
0.5,0.514285714285714,0.528571428571429,0.542857142857143,0.557142857142857,
0.571428571428571,0.585714285714286,0.6,0.614285714285714,0.628571428571428,
0.642857142857142,0.657142857142857,0.671428571428571,0.685714285714285,
0.699999999999999,0.714285714285714,0.728571428571428,0.742857142857142,
0.757142857142856,0.771428571428571,0.785714285714285,0.799999999999999,
0.814285714285713,0.828571428571428,0.842857142857142,0.857142857142856,
0.87142857142857,0.885714285714284,0.899999999999999,0.914285714285713,
0.928571428571427,0.942857142857141,0.957142857142856,0.97142857142857,
1.),.UNSPECIFIED.);
#138=B_SPLINE_CURVE_WITH_KNOTS('',3,(#11489,#11490,#11491,#11492,#11493,
#11494,#11495,#11496,#11497,#11498,#11499,#11500,#11501,#11502,#11503,#11504,
#11505,#11506,#11507,#11508,#11509,#11510,#11511,#11512,#11513,#11514,#11515,
#11516,#11517,#11518,#11519,#11520,#11521,#11522,#11523,#11524,#11525,#11526,
#11527,#11528,#11529,#11530,#11531,#11532,#11533,#11534,#11535,#11536,#11537,
#11538,#11539,#11540,#11541,#11542,#11543,#11544,#11545,#11546,#11547,#11548,
#11549,#11550,#11551,#11552,#11553,#11554,#11555,#11556,#11557,#11558),
 .UNSPECIFIED.,.F.,.F.,(4,3,3,3,3,3,3,3,3,3,3,3,3,3,3,3,3,3,3,3,3,3,3,4),
(-0.411449009745582,-0.405504895379435,-0.398537948745384,-0.388735121403136,
-0.382214695205601,-0.375350877782795,-0.367728232806823,-0.35623672553161,
-0.347888396726707,-0.337683279620391,-0.326660059439279,-0.316483474349347,
-0.302658060997721,-0.289316835702375,-0.271192407460765,-0.255261428951979,
-0.231775298732412,-0.202135573328733,-0.161986280135987,-0.12619213402364,
-0.0754619855322879,-0.0360560073833462,-0.00196685495466459,0.),
 .UNSPECIFIED.);
#139=B_SPLINE_CURVE_WITH_KNOTS('',5,(#11710,#11711,#11712,#11713,#11714,
#11715,#11716,#11717,#11718,#11719,#11720,#11721,#11722,#11723,#11724,#11725,
#11726,#11727,#11728,#11729,#11730,#11731,#11732,#11733,#11734,#11735,#11736,
#11737,#11738,#11739,#11740,#11741,#11742,#11743,#11744,#11745,#11746,#11747,
#11748,#11749,#11750,#11751,#11752,#11753,#11754,#11755,#11756,#11757,#11758,
#11759,#11760,#11761,#11762,#11763,#11764,#11765,#11766,#11767,#11768,#11769,
#11770,#11771,#11772,#11773,#11774,#11775,#11776,#11777,#11778,#11779,#11780,
#11781,#11782,#11783),.UNSPECIFIED.,.F.,.F.,(6,1,1,1,1,1,1,1,1,1,1,1,1,
1,1,1,1,1,1,1,1,1,1,1,1,1,1,1,1,1,1,1,1,1,1,1,1,1,1,1,1,1,1,1,1,1,1,1,1,
1,1,1,1,1,1,1,1,1,1,1,1,1,1,1,1,1,1,1,1,6),(0.,0.0142857142857143,0.0285714285714286,
0.0428571428571429,0.0571428571428571,0.0714285714285714,0.0857142857142857,
0.1,0.114285714285714,0.128571428571429,0.142857142857143,0.157142857142857,
0.171428571428571,0.185714285714286,0.2,0.214285714285714,0.228571428571429,
0.242857142857143,0.257142857142857,0.271428571428571,0.285714285714286,
0.3,0.314285714285714,0.328571428571429,0.342857142857143,0.357142857142857,
0.371428571428571,0.385714285714286,0.4,0.414285714285714,0.428571428571429,
0.442857142857143,0.457142857142857,0.471428571428572,0.485714285714286,
0.5,0.514285714285714,0.528571428571429,0.542857142857143,0.557142857142857,
0.571428571428571,0.585714285714286,0.6,0.614285714285714,0.628571428571428,
0.642857142857142,0.657142857142857,0.671428571428571,0.685714285714285,
0.699999999999999,0.714285714285714,0.728571428571428,0.742857142857142,
0.757142857142856,0.771428571428571,0.785714285714285,0.799999999999999,
0.814285714285713,0.828571428571428,0.842857142857142,0.857142857142856,
0.87142857142857,0.885714285714284,0.899999999999999,0.914285714285713,
0.928571428571427,0.942857142857141,0.957142857142856,0.97142857142857,
1.),.UNSPECIFIED.);
#140=B_SPLINE_CURVE_WITH_KNOTS('',3,(#11785,#11786,#11787,#11788,#11789,
#11790,#11791,#11792,#11793,#11794,#11795,#11796,#11797,#11798,#11799,#11800,
#11801,#11802,#11803,#11804,#11805,#11806,#11807,#11808,#11809,#11810,#11811,
#11812,#11813,#11814,#11815,#11816,#11817,#11818,#11819,#11820,#11821,#11822,
#11823,#11824,#11825,#11826,#11827,#11828,#11829,#11830,#11831,#11832,#11833,
#11834,#11835,#11836,#11837,#11838,#11839,#11840,#11841,#11842,#11843,#11844,
#11845,#11846,#11847,#11848,#11849,#11850,#11851),.UNSPECIFIED.,.F.,.F.,
(4,3,3,3,3,3,3,3,3,3,3,3,3,3,3,3,3,3,3,3,3,3,4),(-0.0308474254096501,-0.028244313899376,
-0.0239308455956517,-0.020615260955671,-0.0170461143005811,-0.0150701375011353,
-0.0131660090769615,-0.0115202579423413,-0.0103391768283886,-0.00917732810453088,
-0.0081699370150875,-0.00725747185097503,-0.0064888593825484,-0.00537659347407927,
-0.00470451928981936,-0.00408467782188743,-0.00323202309462087,-0.00269108370824936,
-0.00220561578794048,-0.00169529231835461,-0.000847646159177307,-0.000380223901533956,
0.),.UNSPECIFIED.);
#141=B_SPLINE_CURVE_WITH_KNOTS('',5,(#12009,#12010,#12011,#12012,#12013,
#12014,#12015,#12016,#12017,#12018,#12019,#12020,#12021,#12022,#12023,#12024,
#12025,#12026,#12027,#12028,#12029,#12030,#12031,#12032,#12033,#12034,#12035,
#12036,#12037,#12038,#12039,#12040,#12041,#12042,#12043,#12044,#12045,#12046,
#12047,#12048,#12049,#12050,#12051,#12052,#12053,#12054,#12055,#12056,#12057,
#12058,#12059,#12060,#12061,#12062,#12063,#12064,#12065,#12066,#12067,#12068,
#12069,#12070,#12071,#12072,#12073,#12074,#12075,#12076,#12077,#12078,#12079,
#12080,#12081,#12082),.UNSPECIFIED.,.F.,.F.,(6,1,1,1,1,1,1,1,1,1,1,1,1,
1,1,1,1,1,1,1,1,1,1,1,1,1,1,1,1,1,1,1,1,1,1,1,1,1,1,1,1,1,1,1,1,1,1,1,1,
1,1,1,1,1,1,1,1,1,1,1,1,1,1,1,1,1,1,1,1,6),(0.,0.0142857142857143,0.0285714285714286,
0.0428571428571429,0.0571428571428571,0.0714285714285714,0.0857142857142857,
0.1,0.114285714285714,0.128571428571429,0.142857142857143,0.157142857142857,
0.171428571428571,0.185714285714286,0.2,0.214285714285714,0.228571428571429,
0.242857142857143,0.257142857142857,0.271428571428571,0.285714285714286,
0.3,0.314285714285714,0.328571428571429,0.342857142857143,0.357142857142857,
0.371428571428571,0.385714285714286,0.4,0.414285714285714,0.428571428571429,
0.442857142857143,0.457142857142857,0.471428571428572,0.485714285714286,
0.5,0.514285714285714,0.528571428571429,0.542857142857143,0.557142857142857,
0.571428571428571,0.585714285714286,0.6,0.614285714285714,0.628571428571428,
0.642857142857142,0.657142857142857,0.671428571428571,0.685714285714285,
0.699999999999999,0.714285714285714,0.728571428571428,0.742857142857142,
0.757142857142856,0.771428571428571,0.785714285714285,0.799999999999999,
0.814285714285713,0.828571428571428,0.842857142857142,0.857142857142856,
0.87142857142857,0.885714285714284,0.899999999999999,0.914285714285713,
0.928571428571427,0.942857142857141,0.957142857142856,0.97142857142857,
1.),.UNSPECIFIED.);
#142=B_SPLINE_CURVE_WITH_KNOTS('',3,(#12083,#12084,#12085,#12086,#12087,
#12088,#12089,#12090,#12091,#12092,#12093,#12094,#12095,#12096,#12097,#12098,
#12099,#12100,#12101,#12102,#12103,#12104,#12105,#12106,#12107,#12108,#12109,
#12110,#12111,#12112,#12113,#12114,#12115,#12116,#12117,#12118,#12119,#12120,
#12121,#12122,#12123,#12124,#12125,#12126,#12127,#12128,#12129,#12130,#12131,
#12132,#12133,#12134,#12135,#12136,#12137,#12138,#12139,#12140,#12141,#12142,
#12143,#12144,#12145,#12146,#12147,#12148,#12149,#12150,#12151,#12152),
 .UNSPECIFIED.,.F.,.F.,(4,3,3,3,3,3,3,3,3,3,3,3,3,3,3,3,3,3,3,3,3,3,3,4),
(-0.411449009865562,-0.4055048954869,-0.398537948850747,-0.388735121518256,
-0.382214695319647,-0.375350877895016,-0.3677282329171,-0.35623672563844,
-0.347888396831227,-0.337683279715536,-0.326660059528631,-0.316483474438613,
-0.302658061094389,-0.28931683580642,-0.271192407552387,-0.255261429122638,
-0.231775298922887,-0.202135573548005,-0.161986280573123,-0.126192134261937,
-0.0754619859222758,-0.0360560139042322,-0.00196687400591684,0.),
 .UNSPECIFIED.);
#143=B_SPLINE_CURVE_WITH_KNOTS('',5,(#12304,#12305,#12306,#12307,#12308,
#12309,#12310,#12311,#12312,#12313,#12314,#12315,#12316,#12317,#12318,#12319,
#12320,#12321,#12322,#12323,#12324,#12325,#12326,#12327,#12328,#12329,#12330,
#12331,#12332,#12333,#12334,#12335,#12336,#12337,#12338,#12339,#12340,#12341,
#12342,#12343,#12344,#12345,#12346,#12347,#12348,#12349,#12350,#12351,#12352,
#12353,#12354,#12355,#12356,#12357,#12358,#12359,#12360,#12361,#12362,#12363,
#12364,#12365,#12366,#12367,#12368,#12369,#12370,#12371,#12372,#12373,#12374,
#12375,#12376,#12377),.UNSPECIFIED.,.F.,.F.,(6,1,1,1,1,1,1,1,1,1,1,1,1,
1,1,1,1,1,1,1,1,1,1,1,1,1,1,1,1,1,1,1,1,1,1,1,1,1,1,1,1,1,1,1,1,1,1,1,1,
1,1,1,1,1,1,1,1,1,1,1,1,1,1,1,1,1,1,1,1,6),(0.,0.0142857142857143,0.0285714285714286,
0.0428571428571429,0.0571428571428571,0.0714285714285714,0.0857142857142857,
0.1,0.114285714285714,0.128571428571429,0.142857142857143,0.157142857142857,
0.171428571428571,0.185714285714286,0.2,0.214285714285714,0.228571428571429,
0.242857142857143,0.257142857142857,0.271428571428571,0.285714285714286,
0.3,0.314285714285714,0.328571428571429,0.342857142857143,0.357142857142857,
0.371428571428571,0.385714285714286,0.4,0.414285714285714,0.428571428571429,
0.442857142857143,0.457142857142857,0.471428571428572,0.485714285714286,
0.5,0.514285714285714,0.528571428571429,0.542857142857143,0.557142857142857,
0.571428571428571,0.585714285714286,0.6,0.614285714285714,0.628571428571428,
0.642857142857142,0.657142857142857,0.671428571428571,0.685714285714285,
0.699999999999999,0.714285714285714,0.728571428571428,0.742857142857142,
0.757142857142856,0.771428571428571,0.785714285714285,0.799999999999999,
0.814285714285713,0.828571428571428,0.842857142857142,0.857142857142856,
0.87142857142857,0.885714285714284,0.899999999999999,0.914285714285713,
0.928571428571427,0.942857142857141,0.957142857142856,0.97142857142857,
1.),.UNSPECIFIED.);
#144=B_SPLINE_CURVE_WITH_KNOTS('',3,(#12379,#12380,#12381,#12382,#12383,
#12384,#12385,#12386,#12387,#12388,#12389,#12390,#12391,#12392,#12393,#12394,
#12395,#12396,#12397,#12398,#12399,#12400,#12401,#12402,#12403,#12404,#12405,
#12406,#12407,#12408,#12409,#12410,#12411,#12412,#12413,#12414,#12415,#12416,
#12417,#12418,#12419,#12420,#12421,#12422,#12423,#12424,#12425,#12426,#12427,
#12428,#12429,#12430,#12431,#12432,#12433,#12434,#12435,#12436,#12437,#12438,
#12439,#12440,#12441,#12442,#12443,#12444,#12445),.UNSPECIFIED.,.F.,.F.,
(4,3,3,3,3,3,3,3,3,3,3,3,3,3,3,3,3,3,3,3,3,3,4),(-0.0308474254198399,-0.0282443142846492,
-0.0239308460906392,-0.0206152614646765,-0.0170461144159942,-0.0150701377147652,
-0.0131660089970923,-0.0115202578724558,-0.0103391767515509,-0.00917732806988761,
-0.00816993700370822,-0.00725747182636578,-0.00648885936066672,-0.00537659349685568,
-0.00470451930974872,-0.00408467784315956,-0.00323202308807464,-0.00269108370254087,
-0.00220561578241539,-0.00169529231143548,-0.000847646155717738,-0.000380223898423687,
0.),.UNSPECIFIED.);
#145=B_SPLINE_CURVE_WITH_KNOTS('',5,(#12603,#12604,#12605,#12606,#12607,
#12608,#12609,#12610,#12611,#12612,#12613,#12614,#12615,#12616,#12617,#12618,
#12619,#12620,#12621,#12622,#12623,#12624,#12625,#12626,#12627,#12628,#12629,
#12630,#12631,#12632,#12633,#12634,#12635,#12636,#12637,#12638,#12639,#12640,
#12641,#12642,#12643,#12644,#12645,#12646,#12647,#12648,#12649,#12650,#12651,
#12652,#12653,#12654,#12655,#12656,#12657,#12658,#12659,#12660,#12661,#12662,
#12663,#12664,#12665,#12666,#12667,#12668,#12669,#12670,#12671,#12672,#12673,
#12674,#12675,#12676),.UNSPECIFIED.,.F.,.F.,(6,1,1,1,1,1,1,1,1,1,1,1,1,
1,1,1,1,1,1,1,1,1,1,1,1,1,1,1,1,1,1,1,1,1,1,1,1,1,1,1,1,1,1,1,1,1,1,1,1,
1,1,1,1,1,1,1,1,1,1,1,1,1,1,1,1,1,1,1,1,6),(0.,0.0142857142857143,0.0285714285714286,
0.0428571428571429,0.0571428571428571,0.0714285714285714,0.0857142857142857,
0.1,0.114285714285714,0.128571428571429,0.142857142857143,0.157142857142857,
0.171428571428571,0.185714285714286,0.2,0.214285714285714,0.228571428571429,
0.242857142857143,0.257142857142857,0.271428571428571,0.285714285714286,
0.3,0.314285714285714,0.328571428571429,0.342857142857143,0.357142857142857,
0.371428571428571,0.385714285714286,0.4,0.414285714285714,0.428571428571429,
0.442857142857143,0.457142857142857,0.471428571428572,0.485714285714286,
0.5,0.514285714285714,0.528571428571429,0.542857142857143,0.557142857142857,
0.571428571428571,0.585714285714286,0.6,0.614285714285714,0.628571428571428,
0.642857142857142,0.657142857142857,0.671428571428571,0.685714285714285,
0.699999999999999,0.714285714285714,0.728571428571428,0.742857142857142,
0.757142857142856,0.771428571428571,0.785714285714285,0.799999999999999,
0.814285714285713,0.828571428571428,0.842857142857142,0.857142857142856,
0.87142857142857,0.885714285714284,0.899999999999999,0.914285714285713,
0.928571428571427,0.942857142857141,0.957142857142856,0.97142857142857,
1.),.UNSPECIFIED.);
#146=B_SPLINE_CURVE_WITH_KNOTS('',3,(#12677,#12678,#12679,#12680,#12681,
#12682,#12683,#12684,#12685,#12686,#12687,#12688,#12689,#12690,#12691,#12692,
#12693,#12694,#12695,#12696,#12697,#12698,#12699,#12700,#12701,#12702,#12703,
#12704,#12705,#12706,#12707,#12708,#12709,#12710,#12711,#12712,#12713,#12714,
#12715,#12716,#12717,#12718,#12719,#12720,#12721,#12722,#12723,#12724,#12725,
#12726,#12727,#12728,#12729,#12730,#12731,#12732,#12733,#12734,#12735,#12736,
#12737,#12738,#12739,#12740,#12741,#12742,#12743,#12744,#12745,#12746),
 .UNSPECIFIED.,.F.,.F.,(4,3,3,3,3,3,3,3,3,3,3,3,3,3,3,3,3,3,3,3,3,3,3,4),
(-0.411449010137647,-0.405504895753404,-0.398537949112127,-0.388735121773796,
-0.382214695570712,-0.375350878142277,-0.367728233158118,-0.356236725871927,
-0.347888397059155,-0.337683279939957,-0.326660059745585,-0.316483474644296,
-0.302658061251899,-0.289316835931869,-0.271192407516363,-0.255261428973649,
-0.231775298903159,-0.202135573529554,-0.161986280339301,-0.126192134013684,
-0.0754619855442812,-0.0360560094852106,-0.00196686131918792,0.),
 .UNSPECIFIED.);
#147=B_SPLINE_CURVE_WITH_KNOTS('',5,(#12898,#12899,#12900,#12901,#12902,
#12903,#12904,#12905,#12906,#12907,#12908,#12909,#12910,#12911,#12912,#12913,
#12914,#12915,#12916,#12917,#12918,#12919,#12920,#12921,#12922,#12923,#12924,
#12925,#12926,#12927,#12928,#12929,#12930,#12931,#12932,#12933,#12934,#12935,
#12936,#12937,#12938,#12939,#12940,#12941,#12942,#12943,#12944,#12945,#12946,
#12947,#12948,#12949,#12950,#12951,#12952,#12953,#12954,#12955,#12956,#12957,
#12958,#12959,#12960,#12961,#12962,#12963,#12964,#12965,#12966,#12967,#12968,
#12969,#12970,#12971),.UNSPECIFIED.,.F.,.F.,(6,1,1,1,1,1,1,1,1,1,1,1,1,
1,1,1,1,1,1,1,1,1,1,1,1,1,1,1,1,1,1,1,1,1,1,1,1,1,1,1,1,1,1,1,1,1,1,1,1,
1,1,1,1,1,1,1,1,1,1,1,1,1,1,1,1,1,1,1,1,6),(0.,0.0142857142857143,0.0285714285714286,
0.0428571428571429,0.0571428571428571,0.0714285714285714,0.0857142857142857,
0.1,0.114285714285714,0.128571428571429,0.142857142857143,0.157142857142857,
0.171428571428571,0.185714285714286,0.2,0.214285714285714,0.228571428571429,
0.242857142857143,0.257142857142857,0.271428571428571,0.285714285714286,
0.3,0.314285714285714,0.328571428571429,0.342857142857143,0.357142857142857,
0.371428571428571,0.385714285714286,0.4,0.414285714285714,0.428571428571429,
0.442857142857143,0.457142857142857,0.471428571428572,0.485714285714286,
0.5,0.514285714285714,0.528571428571429,0.542857142857143,0.557142857142857,
0.571428571428571,0.585714285714286,0.6,0.614285714285714,0.628571428571428,
0.642857142857142,0.657142857142857,0.671428571428571,0.685714285714285,
0.699999999999999,0.714285714285714,0.728571428571428,0.742857142857142,
0.757142857142856,0.771428571428571,0.785714285714285,0.799999999999999,
0.814285714285713,0.828571428571428,0.842857142857142,0.857142857142856,
0.87142857142857,0.885714285714284,0.899999999999999,0.914285714285713,
0.928571428571427,0.942857142857141,0.957142857142856,0.97142857142857,
1.),.UNSPECIFIED.);
#148=B_SPLINE_CURVE_WITH_KNOTS('',3,(#12973,#12974,#12975,#12976,#12977,
#12978,#12979,#12980,#12981,#12982,#12983,#12984,#12985,#12986,#12987,#12988,
#12989,#12990,#12991,#12992,#12993,#12994,#12995,#12996,#12997,#12998,#12999,
#13000,#13001,#13002,#13003,#13004,#13005,#13006,#13007,#13008,#13009,#13010,
#13011,#13012,#13013,#13014,#13015,#13016,#13017,#13018,#13019,#13020,#13021,
#13022,#13023,#13024,#13025,#13026,#13027,#13028,#13029,#13030,#13031,#13032,
#13033,#13034,#13035,#13036,#13037,#13038,#13039),.UNSPECIFIED.,.F.,.F.,
(4,3,3,3,3,3,3,3,3,3,3,3,3,3,3,3,3,3,3,3,3,3,4),(-0.0308474254388288,-0.0282443142460501,
-0.0239308460091484,-0.0206152613794386,-0.0170461144143175,-0.0150701377107825,
-0.0131660090144569,-0.0115202578876498,-0.0103391767664952,-0.00917732807839727,
-0.00816993700961439,-0.0072574718319948,-0.00648885936575202,-0.00537659349968903,
-0.00470451931222791,-0.00408467784513401,-0.00323202309051337,-0.00269108370452265,
-0.00220561578410232,-0.00169529231285346,-0.00084764615642673,-0.000380223898580438,
0.),.UNSPECIFIED.);
#149=B_SPLINE_CURVE_WITH_KNOTS('',5,(#13197,#13198,#13199,#13200,#13201,
#13202,#13203,#13204,#13205,#13206,#13207,#13208,#13209,#13210,#13211,#13212,
#13213,#13214,#13215,#13216,#13217,#13218,#13219,#13220,#13221,#13222,#13223,
#13224,#13225,#13226,#13227,#13228,#13229,#13230,#13231,#13232,#13233,#13234,
#13235,#13236,#13237,#13238,#13239,#13240,#13241,#13242,#13243,#13244,#13245,
#13246,#13247,#13248,#13249,#13250,#13251,#13252,#13253,#13254,#13255,#13256,
#13257,#13258,#13259,#13260,#13261,#13262,#13263,#13264,#13265,#13266,#13267,
#13268,#13269,#13270),.UNSPECIFIED.,.F.,.F.,(6,1,1,1,1,1,1,1,1,1,1,1,1,
1,1,1,1,1,1,1,1,1,1,1,1,1,1,1,1,1,1,1,1,1,1,1,1,1,1,1,1,1,1,1,1,1,1,1,1,
1,1,1,1,1,1,1,1,1,1,1,1,1,1,1,1,1,1,1,1,6),(0.,0.0142857142857143,0.0285714285714286,
0.0428571428571429,0.0571428571428571,0.0714285714285714,0.0857142857142857,
0.1,0.114285714285714,0.128571428571429,0.142857142857143,0.157142857142857,
0.171428571428571,0.185714285714286,0.2,0.214285714285714,0.228571428571429,
0.242857142857143,0.257142857142857,0.271428571428571,0.285714285714286,
0.3,0.314285714285714,0.328571428571429,0.342857142857143,0.357142857142857,
0.371428571428571,0.385714285714286,0.4,0.414285714285714,0.428571428571429,
0.442857142857143,0.457142857142857,0.471428571428572,0.485714285714286,
0.5,0.514285714285714,0.528571428571429,0.542857142857143,0.557142857142857,
0.571428571428571,0.585714285714286,0.6,0.614285714285714,0.628571428571428,
0.642857142857142,0.657142857142857,0.671428571428571,0.685714285714285,
0.699999999999999,0.714285714285714,0.728571428571428,0.742857142857142,
0.757142857142856,0.771428571428571,0.785714285714285,0.799999999999999,
0.814285714285713,0.828571428571428,0.842857142857142,0.857142857142856,
0.87142857142857,0.885714285714284,0.899999999999999,0.914285714285713,
0.928571428571427,0.942857142857141,0.957142857142856,0.97142857142857,
1.),.UNSPECIFIED.);
#150=B_SPLINE_CURVE_WITH_KNOTS('',3,(#13271,#13272,#13273,#13274,#13275,
#13276,#13277,#13278,#13279,#13280,#13281,#13282,#13283,#13284,#13285,#13286,
#13287,#13288,#13289,#13290,#13291,#13292,#13293,#13294,#13295,#13296,#13297,
#13298,#13299,#13300,#13301,#13302,#13303,#13304,#13305,#13306,#13307,#13308,
#13309,#13310,#13311,#13312,#13313,#13314,#13315,#13316,#13317,#13318,#13319,
#13320,#13321,#13322,#13323,#13324,#13325,#13326,#13327,#13328,#13329,#13330,
#13331,#13332,#13333,#13334,#13335,#13336,#13337,#13338,#13339,#13340),
 .UNSPECIFIED.,.F.,.F.,(4,3,3,3,3,3,3,3,3,3,3,3,3,3,3,3,3,3,3,3,3,3,3,4),
(-0.41144900992668,-0.405504895550952,-0.398537948913654,-0.388735121571637,
-0.382214695372107,-0.37535087794608,-0.367728232965685,-0.356236725685507,
-0.347888396876633,-0.33768327976105,-0.326660059574477,-0.316483474477592,
-0.302658061103083,-0.289316835800213,-0.271192407406943,-0.255261428869757,
-0.231775298804757,-0.202135573441996,-0.161986280303818,-0.126192134093902,
-0.0754619856550688,-0.0360560111222661,-0.00196686536757399,0.),
 .UNSPECIFIED.);
#151=B_SPLINE_CURVE_WITH_KNOTS('',5,(#13492,#13493,#13494,#13495,#13496,
#13497,#13498,#13499,#13500,#13501,#13502,#13503,#13504,#13505,#13506,#13507,
#13508,#13509,#13510,#13511,#13512,#13513,#13514,#13515,#13516,#13517,#13518,
#13519,#13520,#13521,#13522,#13523,#13524,#13525,#13526,#13527,#13528,#13529,
#13530,#13531,#13532,#13533,#13534,#13535,#13536,#13537,#13538,#13539,#13540,
#13541,#13542,#13543,#13544,#13545,#13546,#13547,#13548,#13549,#13550,#13551,
#13552,#13553,#13554,#13555,#13556,#13557,#13558,#13559,#13560,#13561,#13562,
#13563,#13564,#13565),.UNSPECIFIED.,.F.,.F.,(6,1,1,1,1,1,1,1,1,1,1,1,1,
1,1,1,1,1,1,1,1,1,1,1,1,1,1,1,1,1,1,1,1,1,1,1,1,1,1,1,1,1,1,1,1,1,1,1,1,
1,1,1,1,1,1,1,1,1,1,1,1,1,1,1,1,1,1,1,1,6),(0.,0.0142857142857143,0.0285714285714286,
0.0428571428571429,0.0571428571428571,0.0714285714285714,0.0857142857142857,
0.1,0.114285714285714,0.128571428571429,0.142857142857143,0.157142857142857,
0.171428571428571,0.185714285714286,0.2,0.214285714285714,0.228571428571429,
0.242857142857143,0.257142857142857,0.271428571428571,0.285714285714286,
0.3,0.314285714285714,0.328571428571429,0.342857142857143,0.357142857142857,
0.371428571428571,0.385714285714286,0.4,0.414285714285714,0.428571428571429,
0.442857142857143,0.457142857142857,0.471428571428572,0.485714285714286,
0.5,0.514285714285714,0.528571428571429,0.542857142857143,0.557142857142857,
0.571428571428571,0.585714285714286,0.6,0.614285714285714,0.628571428571428,
0.642857142857142,0.657142857142857,0.671428571428571,0.685714285714285,
0.699999999999999,0.714285714285714,0.728571428571428,0.742857142857142,
0.757142857142856,0.771428571428571,0.785714285714285,0.799999999999999,
0.814285714285713,0.828571428571428,0.842857142857142,0.857142857142856,
0.87142857142857,0.885714285714284,0.899999999999999,0.914285714285713,
0.928571428571427,0.942857142857141,0.957142857142856,0.97142857142857,
1.),.UNSPECIFIED.);
#152=B_SPLINE_CURVE_WITH_KNOTS('',3,(#13567,#13568,#13569,#13570,#13571,
#13572,#13573,#13574,#13575,#13576,#13577,#13578,#13579,#13580,#13581,#13582,
#13583,#13584,#13585,#13586,#13587,#13588,#13589,#13590,#13591,#13592,#13593,
#13594,#13595,#13596,#13597,#13598,#13599,#13600,#13601,#13602,#13603,#13604,
#13605,#13606,#13607,#13608,#13609,#13610,#13611,#13612,#13613,#13614,#13615,
#13616,#13617,#13618,#13619,#13620,#13621,#13622,#13623,#13624,#13625,#13626,
#13627,#13628,#13629,#13630,#13631,#13632,#13633),.UNSPECIFIED.,.F.,.F.,
(4,3,3,3,3,3,3,3,3,3,3,3,3,3,3,3,3,3,3,3,3,3,4),(-0.0308474254052201,-0.0282443140946725,
-0.0239308458458541,-0.0206152612254046,-0.0170461143478486,-0.015070137591752,
-0.0131660090404763,-0.0115202579104168,-0.0103391767922971,-0.00917732808736861,
-0.0081699370073885,-0.00725747183607438,-0.00648885936953476,-0.00537659348374253,
-0.00470451929827472,-0.00408467783114113,-0.00323202309011053,-0.00269108370432218,
-0.00220561578425795,-0.00169529231400166,-0.000847646157000828,-0.000380223899135919,
0.),.UNSPECIFIED.);
#153=B_SPLINE_CURVE_WITH_KNOTS('',5,(#13791,#13792,#13793,#13794,#13795,
#13796,#13797,#13798,#13799,#13800,#13801,#13802,#13803,#13804,#13805,#13806,
#13807,#13808,#13809,#13810,#13811,#13812,#13813,#13814,#13815,#13816,#13817,
#13818,#13819,#13820,#13821,#13822,#13823,#13824,#13825,#13826,#13827,#13828,
#13829,#13830,#13831,#13832,#13833,#13834,#13835,#13836,#13837,#13838,#13839,
#13840,#13841,#13842,#13843,#13844,#13845,#13846,#13847,#13848,#13849,#13850,
#13851,#13852,#13853,#13854,#13855,#13856,#13857,#13858,#13859,#13860,#13861,
#13862,#13863,#13864),.UNSPECIFIED.,.F.,.F.,(6,1,1,1,1,1,1,1,1,1,1,1,1,
1,1,1,1,1,1,1,1,1,1,1,1,1,1,1,1,1,1,1,1,1,1,1,1,1,1,1,1,1,1,1,1,1,1,1,1,
1,1,1,1,1,1,1,1,1,1,1,1,1,1,1,1,1,1,1,1,6),(0.,0.0142857142857143,0.0285714285714286,
0.0428571428571429,0.0571428571428571,0.0714285714285714,0.0857142857142857,
0.1,0.114285714285714,0.128571428571429,0.142857142857143,0.157142857142857,
0.171428571428571,0.185714285714286,0.2,0.214285714285714,0.228571428571429,
0.242857142857143,0.257142857142857,0.271428571428571,0.285714285714286,
0.3,0.314285714285714,0.328571428571429,0.342857142857143,0.357142857142857,
0.371428571428571,0.385714285714286,0.4,0.414285714285714,0.428571428571429,
0.442857142857143,0.457142857142857,0.471428571428572,0.485714285714286,
0.5,0.514285714285714,0.528571428571429,0.542857142857143,0.557142857142857,
0.571428571428571,0.585714285714286,0.6,0.614285714285714,0.628571428571428,
0.642857142857142,0.657142857142857,0.671428571428571,0.685714285714285,
0.699999999999999,0.714285714285714,0.728571428571428,0.742857142857142,
0.757142857142856,0.771428571428571,0.785714285714285,0.799999999999999,
0.814285714285713,0.828571428571428,0.842857142857142,0.857142857142856,
0.87142857142857,0.885714285714284,0.899999999999999,0.914285714285713,
0.928571428571427,0.942857142857141,0.957142857142856,0.97142857142857,
1.),.UNSPECIFIED.);
#154=B_SPLINE_CURVE_WITH_KNOTS('',3,(#13865,#13866,#13867,#13868,#13869,
#13870,#13871,#13872,#13873,#13874,#13875,#13876,#13877,#13878,#13879,#13880,
#13881,#13882,#13883,#13884,#13885,#13886,#13887,#13888,#13889,#13890,#13891,
#13892,#13893,#13894,#13895,#13896,#13897,#13898,#13899,#13900,#13901,#13902,
#13903,#13904,#13905,#13906,#13907,#13908,#13909,#13910,#13911,#13912,#13913,
#13914,#13915,#13916,#13917,#13918,#13919,#13920,#13921,#13922,#13923,#13924,
#13925,#13926,#13927,#13928,#13929,#13930,#13931,#13932,#13933,#13934),
 .UNSPECIFIED.,.F.,.F.,(4,3,3,3,3,3,3,3,3,3,3,3,3,3,3,3,3,3,3,3,3,3,3,4),
(-0.411449009805915,-0.405504895443787,-0.398537948811133,-0.388735121455847,
-0.382214695257969,-0.375350877833497,-0.367728232855643,-0.356236725578904,
-0.347888396774101,-0.337683279662952,-0.326660059480431,-0.316483474386569,
-0.302658061019101,-0.289316835720957,-0.271192407372165,-0.25526142885209,
-0.231775298779651,-0.202135573443613,-0.161986280308302,-0.126192134070803,
-0.0754619857048084,-0.0360560114441301,-0.00196686623016366,0.),
 .UNSPECIFIED.);
#155=B_SPLINE_CURVE_WITH_KNOTS('',5,(#14086,#14087,#14088,#14089,#14090,
#14091,#14092,#14093,#14094,#14095,#14096,#14097,#14098,#14099,#14100,#14101,
#14102,#14103,#14104,#14105,#14106,#14107,#14108,#14109,#14110,#14111,#14112,
#14113,#14114,#14115,#14116,#14117,#14118,#14119,#14120,#14121,#14122,#14123,
#14124,#14125,#14126,#14127,#14128,#14129,#14130,#14131,#14132,#14133,#14134,
#14135,#14136,#14137,#14138,#14139,#14140,#14141,#14142,#14143,#14144,#14145,
#14146,#14147,#14148,#14149,#14150,#14151,#14152,#14153,#14154,#14155,#14156,
#14157,#14158,#14159),.UNSPECIFIED.,.F.,.F.,(6,1,1,1,1,1,1,1,1,1,1,1,1,
1,1,1,1,1,1,1,1,1,1,1,1,1,1,1,1,1,1,1,1,1,1,1,1,1,1,1,1,1,1,1,1,1,1,1,1,
1,1,1,1,1,1,1,1,1,1,1,1,1,1,1,1,1,1,1,1,6),(0.,0.0142857142857143,0.0285714285714286,
0.0428571428571429,0.0571428571428571,0.0714285714285714,0.0857142857142857,
0.1,0.114285714285714,0.128571428571429,0.142857142857143,0.157142857142857,
0.171428571428571,0.185714285714286,0.2,0.214285714285714,0.228571428571429,
0.242857142857143,0.257142857142857,0.271428571428571,0.285714285714286,
0.3,0.314285714285714,0.328571428571429,0.342857142857143,0.357142857142857,
0.371428571428571,0.385714285714286,0.4,0.414285714285714,0.428571428571429,
0.442857142857143,0.457142857142857,0.471428571428572,0.485714285714286,
0.5,0.514285714285714,0.528571428571429,0.542857142857143,0.557142857142857,
0.571428571428571,0.585714285714286,0.6,0.614285714285714,0.628571428571428,
0.642857142857142,0.657142857142857,0.671428571428571,0.685714285714285,
0.699999999999999,0.714285714285714,0.728571428571428,0.742857142857142,
0.757142857142856,0.771428571428571,0.785714285714285,0.799999999999999,
0.814285714285713,0.828571428571428,0.842857142857142,0.857142857142856,
0.87142857142857,0.885714285714284,0.899999999999999,0.914285714285713,
0.928571428571427,0.942857142857141,0.957142857142856,0.97142857142857,
1.),.UNSPECIFIED.);
#156=B_SPLINE_CURVE_WITH_KNOTS('',3,(#14161,#14162,#14163,#14164,#14165,
#14166,#14167,#14168,#14169,#14170,#14171,#14172,#14173,#14174,#14175,#14176,
#14177,#14178,#14179,#14180,#14181,#14182,#14183,#14184,#14185,#14186,#14187,
#14188,#14189,#14190,#14191,#14192,#14193,#14194,#14195,#14196,#14197,#14198,
#14199,#14200,#14201,#14202,#14203,#14204,#14205,#14206,#14207,#14208,#14209,
#14210,#14211,#14212,#14213,#14214,#14215,#14216,#14217,#14218,#14219,#14220,
#14221,#14222,#14223,#14224,#14225,#14226,#14227),.UNSPECIFIED.,.F.,.F.,
(4,3,3,3,3,3,3,3,3,3,3,3,3,3,3,3,3,3,3,3,3,3,4),(-0.0308474254313729,-0.0282443144331512,
-0.0239308462436385,-0.0206152616062002,-0.017046114491142,-0.0150701378789916,
-0.0131660089309141,-0.0115202578145499,-0.0103391766904584,-0.0091773280428693,
-0.00816993699591886,-0.00725747180427489,-0.00648885934148822,-0.00537659351838039,
-0.00470451932858284,-0.00408467786302119,-0.00323202308259216,-0.00269108369773592,
-0.00220561577775678,-0.00169529230541892,-0.00084764615270946,-0.000380223895080282,
0.),.UNSPECIFIED.);
#157=B_SPLINE_CURVE_WITH_KNOTS('',5,(#14385,#14386,#14387,#14388,#14389,
#14390,#14391,#14392,#14393,#14394,#14395,#14396,#14397,#14398,#14399,#14400,
#14401,#14402,#14403,#14404,#14405,#14406,#14407,#14408,#14409,#14410,#14411,
#14412,#14413,#14414,#14415,#14416,#14417,#14418,#14419,#14420,#14421,#14422,
#14423,#14424,#14425,#14426,#14427,#14428,#14429,#14430,#14431,#14432,#14433,
#14434,#14435,#14436,#14437,#14438,#14439,#14440,#14441,#14442,#14443,#14444,
#14445,#14446,#14447,#14448,#14449,#14450,#14451,#14452,#14453,#14454,#14455,
#14456,#14457,#14458),.UNSPECIFIED.,.F.,.F.,(6,1,1,1,1,1,1,1,1,1,1,1,1,
1,1,1,1,1,1,1,1,1,1,1,1,1,1,1,1,1,1,1,1,1,1,1,1,1,1,1,1,1,1,1,1,1,1,1,1,
1,1,1,1,1,1,1,1,1,1,1,1,1,1,1,1,1,1,1,1,6),(0.,0.0142857142857143,0.0285714285714286,
0.0428571428571429,0.0571428571428571,0.0714285714285714,0.0857142857142857,
0.1,0.114285714285714,0.128571428571429,0.142857142857143,0.157142857142857,
0.171428571428571,0.185714285714286,0.2,0.214285714285714,0.228571428571429,
0.242857142857143,0.257142857142857,0.271428571428571,0.285714285714286,
0.3,0.314285714285714,0.328571428571429,0.342857142857143,0.357142857142857,
0.371428571428571,0.385714285714286,0.4,0.414285714285714,0.428571428571429,
0.442857142857143,0.457142857142857,0.471428571428572,0.485714285714286,
0.5,0.514285714285714,0.528571428571429,0.542857142857143,0.557142857142857,
0.571428571428571,0.585714285714286,0.6,0.614285714285714,0.628571428571428,
0.642857142857142,0.657142857142857,0.671428571428571,0.685714285714285,
0.699999999999999,0.714285714285714,0.728571428571428,0.742857142857142,
0.757142857142856,0.771428571428571,0.785714285714285,0.799999999999999,
0.814285714285713,0.828571428571428,0.842857142857142,0.857142857142856,
0.87142857142857,0.885714285714284,0.899999999999999,0.914285714285713,
0.928571428571427,0.942857142857141,0.957142857142856,0.97142857142857,
1.),.UNSPECIFIED.);
#158=B_SPLINE_CURVE_WITH_KNOTS('',3,(#14459,#14460,#14461,#14462,#14463,
#14464,#14465,#14466,#14467,#14468,#14469,#14470,#14471,#14472,#14473,#14474,
#14475,#14476,#14477,#14478,#14479,#14480,#14481,#14482,#14483,#14484,#14485,
#14486,#14487,#14488,#14489,#14490,#14491,#14492,#14493,#14494,#14495,#14496,
#14497,#14498,#14499,#14500,#14501,#14502,#14503,#14504,#14505,#14506,#14507,
#14508,#14509,#14510,#14511,#14512,#14513,#14514,#14515,#14516,#14517,#14518,
#14519,#14520,#14521,#14522,#14523,#14524,#14525,#14526,#14527,#14528),
 .UNSPECIFIED.,.F.,.F.,(4,3,3,3,3,3,3,3,3,3,3,3,3,3,3,3,3,3,3,3,3,3,3,4),
(-0.411449009745582,-0.405504895379435,-0.398537948745384,-0.388735121403136,
-0.382214695205601,-0.375350877782795,-0.367728232806823,-0.35623672553161,
-0.347888396726707,-0.337683279620391,-0.326660059439279,-0.316483474349347,
-0.302658060997721,-0.289316835702375,-0.271192407460765,-0.255261428951979,
-0.231775298732412,-0.202135573328733,-0.161986280135987,-0.12619213402364,
-0.0754619855322879,-0.0360560073833462,-0.00196685495466459,0.),
 .UNSPECIFIED.);
#159=B_SPLINE_CURVE_WITH_KNOTS('',5,(#14680,#14681,#14682,#14683,#14684,
#14685,#14686,#14687,#14688,#14689,#14690,#14691,#14692,#14693,#14694,#14695,
#14696,#14697,#14698,#14699,#14700,#14701,#14702,#14703,#14704,#14705,#14706,
#14707,#14708,#14709,#14710,#14711,#14712,#14713,#14714,#14715,#14716,#14717,
#14718,#14719,#14720,#14721,#14722,#14723,#14724,#14725,#14726,#14727,#14728,
#14729,#14730,#14731,#14732,#14733,#14734,#14735,#14736,#14737,#14738,#14739,
#14740,#14741,#14742,#14743,#14744,#14745,#14746,#14747,#14748,#14749,#14750,
#14751,#14752,#14753),.UNSPECIFIED.,.F.,.F.,(6,1,1,1,1,1,1,1,1,1,1,1,1,
1,1,1,1,1,1,1,1,1,1,1,1,1,1,1,1,1,1,1,1,1,1,1,1,1,1,1,1,1,1,1,1,1,1,1,1,
1,1,1,1,1,1,1,1,1,1,1,1,1,1,1,1,1,1,1,1,6),(0.,0.0142857142857143,0.0285714285714286,
0.0428571428571429,0.0571428571428571,0.0714285714285714,0.0857142857142857,
0.1,0.114285714285714,0.128571428571429,0.142857142857143,0.157142857142857,
0.171428571428571,0.185714285714286,0.2,0.214285714285714,0.228571428571429,
0.242857142857143,0.257142857142857,0.271428571428571,0.285714285714286,
0.3,0.314285714285714,0.328571428571429,0.342857142857143,0.357142857142857,
0.371428571428571,0.385714285714286,0.4,0.414285714285714,0.428571428571429,
0.442857142857143,0.457142857142857,0.471428571428572,0.485714285714286,
0.5,0.514285714285714,0.528571428571429,0.542857142857143,0.557142857142857,
0.571428571428571,0.585714285714286,0.6,0.614285714285714,0.628571428571428,
0.642857142857142,0.657142857142857,0.671428571428571,0.685714285714285,
0.699999999999999,0.714285714285714,0.728571428571428,0.742857142857142,
0.757142857142856,0.771428571428571,0.785714285714285,0.799999999999999,
0.814285714285713,0.828571428571428,0.842857142857142,0.857142857142856,
0.87142857142857,0.885714285714284,0.899999999999999,0.914285714285713,
0.928571428571427,0.942857142857141,0.957142857142856,0.97142857142857,
1.),.UNSPECIFIED.);
#160=B_SPLINE_CURVE_WITH_KNOTS('',3,(#14755,#14756,#14757,#14758,#14759,
#14760,#14761,#14762,#14763,#14764,#14765,#14766,#14767,#14768,#14769,#14770,
#14771,#14772,#14773,#14774,#14775,#14776,#14777,#14778,#14779,#14780,#14781,
#14782,#14783,#14784,#14785,#14786,#14787,#14788,#14789,#14790,#14791,#14792,
#14793,#14794,#14795,#14796,#14797,#14798,#14799,#14800,#14801,#14802,#14803,
#14804,#14805,#14806,#14807,#14808,#14809,#14810,#14811,#14812,#14813,#14814,
#14815,#14816,#14817,#14818,#14819,#14820,#14821),.UNSPECIFIED.,.F.,.F.,
(4,3,3,3,3,3,3,3,3,3,3,3,3,3,3,3,3,3,3,3,3,3,4),(-0.0308474254096501,-0.028244313899376,
-0.0239308455956517,-0.020615260955671,-0.0170461143005811,-0.0150701375011353,
-0.0131660090769615,-0.0115202579423413,-0.0103391768283886,-0.00917732810453088,
-0.0081699370150875,-0.00725747185097503,-0.0064888593825484,-0.00537659347407927,
-0.00470451928981936,-0.00408467782188743,-0.00323202309462087,-0.00269108370824936,
-0.00220561578794048,-0.00169529231835461,-0.000847646159177307,-0.000380223901533956,
0.),.UNSPECIFIED.);
#161=B_SPLINE_CURVE_WITH_KNOTS('',5,(#14979,#14980,#14981,#14982,#14983,
#14984,#14985,#14986,#14987,#14988,#14989,#14990,#14991,#14992,#14993,#14994,
#14995,#14996,#14997,#14998,#14999,#15000,#15001,#15002,#15003,#15004,#15005,
#15006,#15007,#15008,#15009,#15010,#15011,#15012,#15013,#15014,#15015,#15016,
#15017,#15018,#15019,#15020,#15021,#15022,#15023,#15024,#15025,#15026,#15027,
#15028,#15029,#15030,#15031,#15032,#15033,#15034,#15035,#15036,#15037,#15038,
#15039,#15040,#15041,#15042,#15043,#15044,#15045,#15046,#15047,#15048,#15049,
#15050,#15051,#15052),.UNSPECIFIED.,.F.,.F.,(6,1,1,1,1,1,1,1,1,1,1,1,1,
1,1,1,1,1,1,1,1,1,1,1,1,1,1,1,1,1,1,1,1,1,1,1,1,1,1,1,1,1,1,1,1,1,1,1,1,
1,1,1,1,1,1,1,1,1,1,1,1,1,1,1,1,1,1,1,1,6),(0.,0.0142857142857143,0.0285714285714286,
0.0428571428571429,0.0571428571428571,0.0714285714285714,0.0857142857142857,
0.1,0.114285714285714,0.128571428571429,0.142857142857143,0.157142857142857,
0.171428571428571,0.185714285714286,0.2,0.214285714285714,0.228571428571429,
0.242857142857143,0.257142857142857,0.271428571428571,0.285714285714286,
0.3,0.314285714285714,0.328571428571429,0.342857142857143,0.357142857142857,
0.371428571428571,0.385714285714286,0.4,0.414285714285714,0.428571428571429,
0.442857142857143,0.457142857142857,0.471428571428572,0.485714285714286,
0.5,0.514285714285714,0.528571428571429,0.542857142857143,0.557142857142857,
0.571428571428571,0.585714285714286,0.6,0.614285714285714,0.628571428571428,
0.642857142857142,0.657142857142857,0.671428571428571,0.685714285714285,
0.699999999999999,0.714285714285714,0.728571428571428,0.742857142857142,
0.757142857142856,0.771428571428571,0.785714285714285,0.799999999999999,
0.814285714285713,0.828571428571428,0.842857142857142,0.857142857142856,
0.87142857142857,0.885714285714284,0.899999999999999,0.914285714285713,
0.928571428571427,0.942857142857141,0.957142857142856,0.97142857142857,
1.),.UNSPECIFIED.);
#162=B_SPLINE_CURVE_WITH_KNOTS('',3,(#15053,#15054,#15055,#15056,#15057,
#15058,#15059,#15060,#15061,#15062,#15063,#15064,#15065,#15066,#15067,#15068,
#15069,#15070,#15071,#15072,#15073,#15074,#15075,#15076,#15077,#15078,#15079,
#15080,#15081,#15082,#15083,#15084,#15085,#15086,#15087,#15088,#15089,#15090,
#15091,#15092,#15093,#15094,#15095,#15096,#15097,#15098,#15099,#15100,#15101,
#15102,#15103,#15104,#15105,#15106,#15107,#15108,#15109,#15110,#15111,#15112,
#15113,#15114,#15115,#15116,#15117,#15118,#15119,#15120,#15121,#15122),
 .UNSPECIFIED.,.F.,.F.,(4,3,3,3,3,3,3,3,3,3,3,3,3,3,3,3,3,3,3,3,3,3,3,4),
(-0.411449009865562,-0.4055048954869,-0.398537948850747,-0.388735121518256,
-0.382214695319647,-0.375350877895016,-0.3677282329171,-0.35623672563844,
-0.347888396831227,-0.337683279715536,-0.326660059528631,-0.316483474438613,
-0.302658061094389,-0.28931683580642,-0.271192407552387,-0.255261429122638,
-0.231775298922887,-0.202135573548005,-0.161986280573123,-0.126192134261937,
-0.0754619859222758,-0.0360560139042322,-0.00196687400591684,0.),
 .UNSPECIFIED.);
#163=B_SPLINE_CURVE_WITH_KNOTS('',5,(#15274,#15275,#15276,#15277,#15278,
#15279,#15280,#15281,#15282,#15283,#15284,#15285,#15286,#15287,#15288,#15289,
#15290,#15291,#15292,#15293,#15294,#15295,#15296,#15297,#15298,#15299,#15300,
#15301,#15302,#15303,#15304,#15305,#15306,#15307,#15308,#15309,#15310,#15311,
#15312,#15313,#15314,#15315,#15316,#15317,#15318,#15319,#15320,#15321,#15322,
#15323,#15324,#15325,#15326,#15327,#15328,#15329,#15330,#15331,#15332,#15333,
#15334,#15335,#15336,#15337,#15338,#15339,#15340,#15341,#15342,#15343,#15344,
#15345,#15346,#15347),.UNSPECIFIED.,.F.,.F.,(6,1,1,1,1,1,1,1,1,1,1,1,1,
1,1,1,1,1,1,1,1,1,1,1,1,1,1,1,1,1,1,1,1,1,1,1,1,1,1,1,1,1,1,1,1,1,1,1,1,
1,1,1,1,1,1,1,1,1,1,1,1,1,1,1,1,1,1,1,1,6),(0.,0.0142857142857143,0.0285714285714286,
0.0428571428571429,0.0571428571428571,0.0714285714285714,0.0857142857142857,
0.1,0.114285714285714,0.128571428571429,0.142857142857143,0.157142857142857,
0.171428571428571,0.185714285714286,0.2,0.214285714285714,0.228571428571429,
0.242857142857143,0.257142857142857,0.271428571428571,0.285714285714286,
0.3,0.314285714285714,0.328571428571429,0.342857142857143,0.357142857142857,
0.371428571428571,0.385714285714286,0.4,0.414285714285714,0.428571428571429,
0.442857142857143,0.457142857142857,0.471428571428572,0.485714285714286,
0.5,0.514285714285714,0.528571428571429,0.542857142857143,0.557142857142857,
0.571428571428571,0.585714285714286,0.6,0.614285714285714,0.628571428571428,
0.642857142857142,0.657142857142857,0.671428571428571,0.685714285714285,
0.699999999999999,0.714285714285714,0.728571428571428,0.742857142857142,
0.757142857142856,0.771428571428571,0.785714285714285,0.799999999999999,
0.814285714285713,0.828571428571428,0.842857142857142,0.857142857142856,
0.87142857142857,0.885714285714284,0.899999999999999,0.914285714285713,
0.928571428571427,0.942857142857141,0.957142857142856,0.97142857142857,
1.),.UNSPECIFIED.);
#164=B_SPLINE_CURVE_WITH_KNOTS('',3,(#15349,#15350,#15351,#15352,#15353,
#15354,#15355,#15356,#15357,#15358,#15359,#15360,#15361,#15362,#15363,#15364,
#15365,#15366,#15367,#15368,#15369,#15370,#15371,#15372,#15373,#15374,#15375,
#15376,#15377,#15378,#15379,#15380,#15381,#15382,#15383,#15384,#15385,#15386,
#15387,#15388,#15389,#15390,#15391,#15392,#15393,#15394,#15395,#15396,#15397,
#15398,#15399,#15400,#15401,#15402,#15403,#15404,#15405,#15406,#15407,#15408,
#15409,#15410,#15411,#15412,#15413,#15414,#15415),.UNSPECIFIED.,.F.,.F.,
(4,3,3,3,3,3,3,3,3,3,3,3,3,3,3,3,3,3,3,3,3,3,4),(-0.0308474254361046,-0.0282443142716837,
-0.0239308460693387,-0.0206152614403016,-0.0170461144189006,-0.0150701377175538,
-0.0131660090058279,-0.0115202578800994,-0.0103391767587464,-0.00917732807603053,
-0.0081699370085221,-0.00725747183125426,-0.00648885936500699,-0.00537659349888438,
-0.00470451931152384,-0.00408467784453854,-0.00323202309003581,-0.00269108370418276,
-0.00220561578378896,-0.00169529231258491,-0.000847646156292456,-0.00038022389874333,
0.),.UNSPECIFIED.);
#165=B_SPLINE_CURVE_WITH_KNOTS('',5,(#15573,#15574,#15575,#15576,#15577,
#15578,#15579,#15580,#15581,#15582,#15583,#15584,#15585,#15586,#15587,#15588,
#15589,#15590,#15591,#15592,#15593,#15594,#15595,#15596,#15597,#15598,#15599,
#15600,#15601,#15602,#15603,#15604,#15605,#15606,#15607,#15608,#15609,#15610,
#15611,#15612,#15613,#15614,#15615,#15616,#15617,#15618,#15619,#15620,#15621,
#15622,#15623,#15624,#15625,#15626,#15627,#15628,#15629,#15630,#15631,#15632,
#15633,#15634,#15635,#15636,#15637,#15638,#15639,#15640,#15641,#15642,#15643,
#15644,#15645,#15646),.UNSPECIFIED.,.F.,.F.,(6,1,1,1,1,1,1,1,1,1,1,1,1,
1,1,1,1,1,1,1,1,1,1,1,1,1,1,1,1,1,1,1,1,1,1,1,1,1,1,1,1,1,1,1,1,1,1,1,1,
1,1,1,1,1,1,1,1,1,1,1,1,1,1,1,1,1,1,1,1,6),(0.,0.0142857142857143,0.0285714285714286,
0.0428571428571429,0.0571428571428571,0.0714285714285714,0.0857142857142857,
0.1,0.114285714285714,0.128571428571429,0.142857142857143,0.157142857142857,
0.171428571428571,0.185714285714286,0.2,0.214285714285714,0.228571428571429,
0.242857142857143,0.257142857142857,0.271428571428571,0.285714285714286,
0.3,0.314285714285714,0.328571428571429,0.342857142857143,0.357142857142857,
0.371428571428571,0.385714285714286,0.4,0.414285714285714,0.428571428571429,
0.442857142857143,0.457142857142857,0.471428571428572,0.485714285714286,
0.5,0.514285714285714,0.528571428571429,0.542857142857143,0.557142857142857,
0.571428571428571,0.585714285714286,0.6,0.614285714285714,0.628571428571428,
0.642857142857142,0.657142857142857,0.671428571428571,0.685714285714285,
0.699999999999999,0.714285714285714,0.728571428571428,0.742857142857142,
0.757142857142856,0.771428571428571,0.785714285714285,0.799999999999999,
0.814285714285713,0.828571428571428,0.842857142857142,0.857142857142856,
0.87142857142857,0.885714285714284,0.899999999999999,0.914285714285713,
0.928571428571427,0.942857142857141,0.957142857142856,0.97142857142857,
1.),.UNSPECIFIED.);
#166=B_SPLINE_CURVE_WITH_KNOTS('',3,(#15647,#15648,#15649,#15650,#15651,
#15652,#15653,#15654,#15655,#15656,#15657,#15658,#15659,#15660,#15661,#15662,
#15663,#15664,#15665,#15666,#15667,#15668,#15669,#15670,#15671,#15672,#15673,
#15674,#15675,#15676,#15677,#15678,#15679,#15680,#15681,#15682,#15683,#15684,
#15685,#15686,#15687,#15688,#15689,#15690,#15691,#15692,#15693,#15694,#15695,
#15696,#15697,#15698,#15699,#15700,#15701,#15702,#15703,#15704,#15705,#15706,
#15707,#15708,#15709,#15710,#15711,#15712,#15713,#15714,#15715,#15716),
 .UNSPECIFIED.,.F.,.F.,(4,3,3,3,3,3,3,3,3,3,3,3,3,3,3,3,3,3,3,3,3,3,3,4),
(-0.411449009993053,-0.405504895610899,-0.398537948972071,-0.388735121637185,
-0.382214695436393,-0.37535087801037,-0.36772823302889,-0.356236725746737,
-0.347888396936899,-0.337683279821287,-0.326660059631445,-0.316483474534432,
-0.3026580611645,-0.28931683586772,-0.271192407496477,-0.255261428976351,
-0.231775298863032,-0.202135573489481,-0.161986280301393,-0.126192134011822,
-0.0754619855028801,-0.0360560096614338,-0.00196686194487841,0.),
 .UNSPECIFIED.);
#167=B_SPLINE_CURVE_WITH_KNOTS('',5,(#15868,#15869,#15870,#15871,#15872,
#15873,#15874,#15875,#15876,#15877,#15878,#15879,#15880,#15881,#15882,#15883,
#15884,#15885,#15886,#15887,#15888,#15889,#15890,#15891,#15892,#15893,#15894,
#15895,#15896,#15897,#15898,#15899,#15900,#15901,#15902,#15903,#15904,#15905,
#15906,#15907,#15908,#15909,#15910,#15911,#15912,#15913,#15914,#15915,#15916,
#15917,#15918,#15919,#15920,#15921,#15922,#15923,#15924,#15925,#15926,#15927,
#15928,#15929,#15930,#15931,#15932,#15933,#15934,#15935,#15936,#15937,#15938,
#15939,#15940,#15941),.UNSPECIFIED.,.F.,.F.,(6,1,1,1,1,1,1,1,1,1,1,1,1,
1,1,1,1,1,1,1,1,1,1,1,1,1,1,1,1,1,1,1,1,1,1,1,1,1,1,1,1,1,1,1,1,1,1,1,1,
1,1,1,1,1,1,1,1,1,1,1,1,1,1,1,1,1,1,1,1,6),(0.,0.0142857142857143,0.0285714285714286,
0.0428571428571429,0.0571428571428571,0.0714285714285714,0.0857142857142857,
0.1,0.114285714285714,0.128571428571429,0.142857142857143,0.157142857142857,
0.171428571428571,0.185714285714286,0.2,0.214285714285714,0.228571428571429,
0.242857142857143,0.257142857142857,0.271428571428571,0.285714285714286,
0.3,0.314285714285714,0.328571428571429,0.342857142857143,0.357142857142857,
0.371428571428571,0.385714285714286,0.4,0.414285714285714,0.428571428571429,
0.442857142857143,0.457142857142857,0.471428571428572,0.485714285714286,
0.5,0.514285714285714,0.528571428571429,0.542857142857143,0.557142857142857,
0.571428571428571,0.585714285714286,0.6,0.614285714285714,0.628571428571428,
0.642857142857142,0.657142857142857,0.671428571428571,0.685714285714285,
0.699999999999999,0.714285714285714,0.728571428571428,0.742857142857142,
0.757142857142856,0.771428571428571,0.785714285714285,0.799999999999999,
0.814285714285713,0.828571428571428,0.842857142857142,0.857142857142856,
0.87142857142857,0.885714285714284,0.899999999999999,0.914285714285713,
0.928571428571427,0.942857142857141,0.957142857142856,0.97142857142857,
1.),.UNSPECIFIED.);
#168=B_SPLINE_CURVE_WITH_KNOTS('',3,(#15943,#15944,#15945,#15946,#15947,
#15948,#15949,#15950,#15951,#15952,#15953,#15954,#15955,#15956,#15957,#15958,
#15959,#15960,#15961,#15962,#15963,#15964,#15965,#15966,#15967,#15968,#15969,
#15970,#15971,#15972,#15973,#15974,#15975,#15976,#15977,#15978,#15979,#15980,
#15981,#15982,#15983,#15984,#15985,#15986,#15987,#15988,#15989,#15990,#15991,
#15992,#15993,#15994,#15995,#15996,#15997,#15998,#15999,#16000,#16001,#16002,
#16003,#16004,#16005,#16006,#16007,#16008,#16009),.UNSPECIFIED.,.F.,.F.,
(4,3,3,3,3,3,3,3,3,3,3,3,3,3,3,3,3,3,3,3,3,3,4),(-0.0308474254372875,-0.0282443142425791,
-0.0239308460054441,-0.0206152613763472,-0.0170461144127407,-0.0150701377079118,
-0.0131660090146465,-0.0115202578878157,-0.0103391767667528,-0.00917732807920022,
-0.00816993700966646,-0.00725747183268602,-0.00648885936638244,-0.00537659349841556,
-0.00470451931111362,-0.00408467784397183,-0.00323202309066985,-0.00269108370466403,
-0.00220561578425269,-0.00169529231308492,-0.00084764615654246,-0.000380223898520597,
0.),.UNSPECIFIED.);
#169=B_SPLINE_CURVE_WITH_KNOTS('',5,(#16167,#16168,#16169,#16170,#16171,
#16172,#16173,#16174,#16175,#16176,#16177,#16178,#16179,#16180,#16181,#16182,
#16183,#16184,#16185,#16186,#16187,#16188,#16189,#16190,#16191,#16192,#16193,
#16194,#16195,#16196,#16197,#16198,#16199,#16200,#16201,#16202,#16203,#16204,
#16205,#16206,#16207,#16208,#16209,#16210,#16211,#16212,#16213,#16214,#16215,
#16216,#16217,#16218,#16219,#16220,#16221,#16222,#16223,#16224,#16225,#16226,
#16227,#16228,#16229,#16230,#16231,#16232,#16233,#16234,#16235,#16236,#16237,
#16238,#16239,#16240),.UNSPECIFIED.,.F.,.F.,(6,1,1,1,1,1,1,1,1,1,1,1,1,
1,1,1,1,1,1,1,1,1,1,1,1,1,1,1,1,1,1,1,1,1,1,1,1,1,1,1,1,1,1,1,1,1,1,1,1,
1,1,1,1,1,1,1,1,1,1,1,1,1,1,1,1,1,1,1,1,6),(0.,0.0142857142857143,0.0285714285714286,
0.0428571428571429,0.0571428571428571,0.0714285714285714,0.0857142857142857,
0.1,0.114285714285714,0.128571428571429,0.142857142857143,0.157142857142857,
0.171428571428571,0.185714285714286,0.2,0.214285714285714,0.228571428571429,
0.242857142857143,0.257142857142857,0.271428571428571,0.285714285714286,
0.3,0.314285714285714,0.328571428571429,0.342857142857143,0.357142857142857,
0.371428571428571,0.385714285714286,0.4,0.414285714285714,0.428571428571429,
0.442857142857143,0.457142857142857,0.471428571428572,0.485714285714286,
0.5,0.514285714285714,0.528571428571429,0.542857142857143,0.557142857142857,
0.571428571428571,0.585714285714286,0.6,0.614285714285714,0.628571428571428,
0.642857142857142,0.657142857142857,0.671428571428571,0.685714285714285,
0.699999999999999,0.714285714285714,0.728571428571428,0.742857142857142,
0.757142857142856,0.771428571428571,0.785714285714285,0.799999999999999,
0.814285714285713,0.828571428571428,0.842857142857142,0.857142857142856,
0.87142857142857,0.885714285714284,0.899999999999999,0.914285714285713,
0.928571428571427,0.942857142857141,0.957142857142856,0.97142857142857,
1.),.UNSPECIFIED.);
#170=B_SPLINE_CURVE_WITH_KNOTS('',3,(#16241,#16242,#16243,#16244,#16245,
#16246,#16247,#16248,#16249,#16250,#16251,#16252,#16253,#16254,#16255,#16256,
#16257,#16258,#16259,#16260,#16261,#16262,#16263,#16264,#16265,#16266,#16267,
#16268,#16269,#16270,#16271,#16272,#16273,#16274,#16275,#16276,#16277,#16278,
#16279,#16280,#16281,#16282,#16283,#16284,#16285,#16286,#16287,#16288,#16289,
#16290,#16291,#16292,#16293,#16294,#16295,#16296,#16297,#16298,#16299,#16300,
#16301,#16302,#16303,#16304,#16305,#16306,#16307,#16308,#16309,#16310),
 .UNSPECIFIED.,.F.,.F.,(4,3,3,3,3,3,3,3,3,3,3,3,3,3,3,3,3,3,3,3,3,3,3,4),
(-0.411449009936769,-0.405504895560803,-0.398537948923531,-0.388735121582206,
-0.382214695382425,-0.375350877956282,-0.36772823297609,-0.356236725695587,
-0.347888396886988,-0.337683279771699,-0.326660059584262,-0.316483474487346,
-0.302658061115119,-0.289316835813513,-0.271192407420841,-0.2552614288874,
-0.231775298819437,-0.20213557344945,-0.161986280299213,-0.126192134097661,
-0.075461985664044,-0.0360560111596636,-0.00196686546694207,0.),
 .UNSPECIFIED.);
#171=B_SPLINE_CURVE_WITH_KNOTS('',5,(#16462,#16463,#16464,#16465,#16466,
#16467,#16468,#16469,#16470,#16471,#16472,#16473,#16474,#16475,#16476,#16477,
#16478,#16479,#16480,#16481,#16482,#16483,#16484,#16485,#16486,#16487,#16488,
#16489,#16490,#16491,#16492,#16493,#16494,#16495,#16496,#16497,#16498,#16499,
#16500,#16501,#16502,#16503,#16504,#16505,#16506,#16507,#16508,#16509,#16510,
#16511,#16512,#16513,#16514,#16515,#16516,#16517,#16518,#16519,#16520,#16521,
#16522,#16523,#16524,#16525,#16526,#16527,#16528,#16529,#16530,#16531,#16532,
#16533,#16534,#16535),.UNSPECIFIED.,.F.,.F.,(6,1,1,1,1,1,1,1,1,1,1,1,1,
1,1,1,1,1,1,1,1,1,1,1,1,1,1,1,1,1,1,1,1,1,1,1,1,1,1,1,1,1,1,1,1,1,1,1,1,
1,1,1,1,1,1,1,1,1,1,1,1,1,1,1,1,1,1,1,1,6),(0.,0.0142857142857143,0.0285714285714286,
0.0428571428571429,0.0571428571428571,0.0714285714285714,0.0857142857142857,
0.1,0.114285714285714,0.128571428571429,0.142857142857143,0.157142857142857,
0.171428571428571,0.185714285714286,0.2,0.214285714285714,0.228571428571429,
0.242857142857143,0.257142857142857,0.271428571428571,0.285714285714286,
0.3,0.314285714285714,0.328571428571429,0.342857142857143,0.357142857142857,
0.371428571428571,0.385714285714286,0.4,0.414285714285714,0.428571428571429,
0.442857142857143,0.457142857142857,0.471428571428572,0.485714285714286,
0.5,0.514285714285714,0.528571428571429,0.542857142857143,0.557142857142857,
0.571428571428571,0.585714285714286,0.6,0.614285714285714,0.628571428571428,
0.642857142857142,0.657142857142857,0.671428571428571,0.685714285714285,
0.699999999999999,0.714285714285714,0.728571428571428,0.742857142857142,
0.757142857142856,0.771428571428571,0.785714285714285,0.799999999999999,
0.814285714285713,0.828571428571428,0.842857142857142,0.857142857142856,
0.87142857142857,0.885714285714284,0.899999999999999,0.914285714285713,
0.928571428571427,0.942857142857141,0.957142857142856,0.97142857142857,
1.),.UNSPECIFIED.);
#172=B_SPLINE_CURVE_WITH_KNOTS('',3,(#16537,#16538,#16539,#16540,#16541,
#16542,#16543,#16544,#16545,#16546,#16547,#16548,#16549,#16550,#16551,#16552,
#16553,#16554,#16555,#16556,#16557,#16558,#16559,#16560,#16561,#16562,#16563,
#16564,#16565,#16566,#16567,#16568,#16569,#16570,#16571,#16572,#16573,#16574,
#16575,#16576,#16577,#16578,#16579,#16580,#16581,#16582,#16583,#16584,#16585,
#16586,#16587,#16588,#16589,#16590,#16591,#16592,#16593,#16594,#16595,#16596,
#16597,#16598,#16599,#16600,#16601,#16602,#16603),.UNSPECIFIED.,.F.,.F.,
(4,3,3,3,3,3,3,3,3,3,3,3,3,3,3,3,3,3,3,3,3,3,4),(-0.0308474254273919,-0.0282443140912033,
-0.023930845835951,-0.0206152612175604,-0.017046114348032,-0.0150701375777768,
-0.0131660090603802,-0.0115202579278327,-0.0103391768090652,-0.00917732809722278,
-0.00816993701457461,-0.00725747184403407,-0.00648885937658713,-0.00537659348549602,
-0.00470451929980902,-0.00408467783206431,-0.00323202309310146,-0.0026910837068358,
-0.00220561578639057,-0.00169529231588426,-0.00084764615794213,-0.000380223899718856,
0.),.UNSPECIFIED.);
#173=B_SPLINE_CURVE_WITH_KNOTS('',5,(#16761,#16762,#16763,#16764,#16765,
#16766,#16767,#16768,#16769,#16770,#16771,#16772,#16773,#16774,#16775,#16776,
#16777,#16778,#16779,#16780,#16781,#16782,#16783,#16784,#16785,#16786,#16787,
#16788,#16789,#16790,#16791,#16792,#16793,#16794,#16795,#16796,#16797,#16798,
#16799,#16800,#16801,#16802,#16803,#16804,#16805,#16806,#16807,#16808,#16809,
#16810,#16811,#16812,#16813,#16814,#16815,#16816,#16817,#16818,#16819,#16820,
#16821,#16822,#16823,#16824,#16825,#16826,#16827,#16828,#16829,#16830,#16831,
#16832,#16833,#16834),.UNSPECIFIED.,.F.,.F.,(6,1,1,1,1,1,1,1,1,1,1,1,1,
1,1,1,1,1,1,1,1,1,1,1,1,1,1,1,1,1,1,1,1,1,1,1,1,1,1,1,1,1,1,1,1,1,1,1,1,
1,1,1,1,1,1,1,1,1,1,1,1,1,1,1,1,1,1,1,1,6),(0.,0.0142857142857143,0.0285714285714286,
0.0428571428571429,0.0571428571428571,0.0714285714285714,0.0857142857142857,
0.1,0.114285714285714,0.128571428571429,0.142857142857143,0.157142857142857,
0.171428571428571,0.185714285714286,0.2,0.214285714285714,0.228571428571429,
0.242857142857143,0.257142857142857,0.271428571428571,0.285714285714286,
0.3,0.314285714285714,0.328571428571429,0.342857142857143,0.357142857142857,
0.371428571428571,0.385714285714286,0.4,0.414285714285714,0.428571428571429,
0.442857142857143,0.457142857142857,0.471428571428572,0.485714285714286,
0.5,0.514285714285714,0.528571428571429,0.542857142857143,0.557142857142857,
0.571428571428571,0.585714285714286,0.6,0.614285714285714,0.628571428571428,
0.642857142857142,0.657142857142857,0.671428571428571,0.685714285714285,
0.699999999999999,0.714285714285714,0.728571428571428,0.742857142857142,
0.757142857142856,0.771428571428571,0.785714285714285,0.799999999999999,
0.814285714285713,0.828571428571428,0.842857142857142,0.857142857142856,
0.87142857142857,0.885714285714284,0.899999999999999,0.914285714285713,
0.928571428571427,0.942857142857141,0.957142857142856,0.97142857142857,
1.),.UNSPECIFIED.);
#174=B_SPLINE_CURVE_WITH_KNOTS('',3,(#16835,#16836,#16837,#16838,#16839,
#16840,#16841,#16842,#16843,#16844,#16845,#16846,#16847,#16848,#16849,#16850,
#16851,#16852,#16853,#16854,#16855,#16856,#16857,#16858,#16859,#16860,#16861,
#16862,#16863,#16864,#16865,#16866,#16867,#16868,#16869,#16870,#16871,#16872,
#16873,#16874,#16875,#16876,#16877,#16878,#16879,#16880,#16881,#16882,#16883,
#16884,#16885,#16886,#16887,#16888,#16889,#16890,#16891,#16892,#16893,#16894,
#16895,#16896,#16897,#16898,#16899,#16900,#16901,#16902,#16903,#16904),
 .UNSPECIFIED.,.F.,.F.,(4,3,3,3,3,3,3,3,3,3,3,3,3,3,3,3,3,3,3,3,3,3,3,4),
(-0.411449009732374,-0.405504895374025,-0.398537948743379,-0.388735121385456,
-0.382214695188797,-0.375350877765784,-0.367728232789201,-0.356236725514539,
-0.347888396711252,-0.337683279600152,-0.326660059420458,-0.316483474327811,
-0.302658060968815,-0.289316835675101,-0.271192407321049,-0.25526142880334,
-0.231775298738104,-0.202135573394745,-0.161986280278011,-0.12619213408638,
-0.075461986045109,-0.0360560119938936,-0.00196686781714211,0.),
 .UNSPECIFIED.);
#175=B_SPLINE_CURVE_WITH_KNOTS('',5,(#17056,#17057,#17058,#17059,#17060,
#17061,#17062,#17063,#17064,#17065,#17066,#17067,#17068,#17069,#17070,#17071,
#17072,#17073,#17074,#17075,#17076,#17077,#17078,#17079,#17080,#17081,#17082,
#17083,#17084,#17085,#17086,#17087,#17088,#17089,#17090,#17091,#17092,#17093,
#17094,#17095,#17096,#17097,#17098,#17099,#17100,#17101,#17102,#17103,#17104,
#17105,#17106,#17107,#17108,#17109,#17110,#17111,#17112,#17113,#17114,#17115,
#17116,#17117,#17118,#17119,#17120,#17121,#17122,#17123,#17124,#17125,#17126,
#17127,#17128,#17129),.UNSPECIFIED.,.F.,.F.,(6,1,1,1,1,1,1,1,1,1,1,1,1,
1,1,1,1,1,1,1,1,1,1,1,1,1,1,1,1,1,1,1,1,1,1,1,1,1,1,1,1,1,1,1,1,1,1,1,1,
1,1,1,1,1,1,1,1,1,1,1,1,1,1,1,1,1,1,1,1,6),(0.,0.0142857142857143,0.0285714285714286,
0.0428571428571429,0.0571428571428571,0.0714285714285714,0.0857142857142857,
0.1,0.114285714285714,0.128571428571429,0.142857142857143,0.157142857142857,
0.171428571428571,0.185714285714286,0.2,0.214285714285714,0.228571428571429,
0.242857142857143,0.257142857142857,0.271428571428571,0.285714285714286,
0.3,0.314285714285714,0.328571428571429,0.342857142857143,0.357142857142857,
0.371428571428571,0.385714285714286,0.4,0.414285714285714,0.428571428571429,
0.442857142857143,0.457142857142857,0.471428571428572,0.485714285714286,
0.5,0.514285714285714,0.528571428571429,0.542857142857143,0.557142857142857,
0.571428571428571,0.585714285714286,0.6,0.614285714285714,0.628571428571428,
0.642857142857142,0.657142857142857,0.671428571428571,0.685714285714285,
0.699999999999999,0.714285714285714,0.728571428571428,0.742857142857142,
0.757142857142856,0.771428571428571,0.785714285714285,0.799999999999999,
0.814285714285713,0.828571428571428,0.842857142857142,0.857142857142856,
0.87142857142857,0.885714285714284,0.899999999999999,0.914285714285713,
0.928571428571427,0.942857142857141,0.957142857142856,0.97142857142857,
1.),.UNSPECIFIED.);
#176=B_SPLINE_CURVE_WITH_KNOTS('',3,(#17131,#17132,#17133,#17134,#17135,
#17136,#17137,#17138,#17139,#17140,#17141,#17142,#17143,#17144,#17145,#17146,
#17147,#17148,#17149,#17150,#17151,#17152,#17153,#17154,#17155,#17156,#17157,
#17158,#17159,#17160,#17161,#17162,#17163,#17164,#17165,#17166,#17167,#17168,
#17169,#17170,#17171,#17172,#17173,#17174,#17175,#17176,#17177,#17178,#17179,
#17180,#17181,#17182,#17183,#17184,#17185,#17186,#17187,#17188,#17189,#17190,
#17191,#17192,#17193,#17194,#17195,#17196,#17197,#17198,#17199,#17200,#17201,
#17202,#17203,#17204,#17205,#17206,#17207,#17208,#17209,#17210,#17211,#17212),
 .UNSPECIFIED.,.F.,.F.,(4,3,3,3,3,3,3,3,3,3,3,3,3,3,3,3,3,3,3,3,3,3,3,3,
3,3,3,4),(-0.0308474254798612,-0.029574376059012,-0.0279034614454273,-0.0261594951050881,
-0.0245245266610201,-0.0244638420994598,-0.0235024106936745,-0.0226524167819541,
-0.0218081022887322,-0.0210633233132742,-0.0203818283699597,-0.0196859172472405,
-0.0190140811746369,-0.0183610672845718,-0.0175680780754909,-0.0168470831907521,
-0.0157941404913301,-0.0150253842943035,-0.0145558410351065,-0.0144056441754732,
-0.0143445590752705,-0.0129617214128992,-0.0112953999186002,-0.00949202192895945,
-0.00761828414789307,-0.00419987046129966,-0.00201831189392491,0.),
 .UNSPECIFIED.);
#177=B_SPLINE_CURVE_WITH_KNOTS('',5,(#17370,#17371,#17372,#17373,#17374,
#17375,#17376,#17377,#17378,#17379,#17380,#17381,#17382,#17383,#17384,#17385,
#17386,#17387,#17388,#17389,#17390,#17391,#17392,#17393,#17394,#17395,#17396,
#17397,#17398,#17399,#17400,#17401,#17402,#17403,#17404,#17405,#17406,#17407,
#17408,#17409,#17410,#17411,#17412,#17413,#17414,#17415,#17416,#17417,#17418,
#17419,#17420,#17421,#17422,#17423,#17424,#17425,#17426,#17427,#17428,#17429,
#17430,#17431,#17432,#17433,#17434,#17435,#17436,#17437,#17438,#17439,#17440,
#17441,#17442,#17443),.UNSPECIFIED.,.F.,.F.,(6,1,1,1,1,1,1,1,1,1,1,1,1,
1,1,1,1,1,1,1,1,1,1,1,1,1,1,1,1,1,1,1,1,1,1,1,1,1,1,1,1,1,1,1,1,1,1,1,1,
1,1,1,1,1,1,1,1,1,1,1,1,1,1,1,1,1,1,1,1,6),(0.,0.0142857142857143,0.0285714285714286,
0.0428571428571429,0.0571428571428571,0.0714285714285714,0.0857142857142857,
0.1,0.114285714285714,0.128571428571429,0.142857142857143,0.157142857142857,
0.171428571428571,0.185714285714286,0.2,0.214285714285714,0.228571428571429,
0.242857142857143,0.257142857142857,0.271428571428571,0.285714285714286,
0.3,0.314285714285714,0.328571428571429,0.342857142857143,0.357142857142857,
0.371428571428571,0.385714285714286,0.4,0.414285714285714,0.428571428571429,
0.442857142857143,0.457142857142857,0.471428571428572,0.485714285714286,
0.5,0.514285714285714,0.528571428571429,0.542857142857143,0.557142857142857,
0.571428571428571,0.585714285714286,0.6,0.614285714285714,0.628571428571428,
0.642857142857142,0.657142857142857,0.671428571428571,0.685714285714285,
0.699999999999999,0.714285714285714,0.728571428571428,0.742857142857142,
0.757142857142856,0.771428571428571,0.785714285714285,0.799999999999999,
0.814285714285713,0.828571428571428,0.842857142857142,0.857142857142856,
0.87142857142857,0.885714285714284,0.899999999999999,0.914285714285713,
0.928571428571427,0.942857142857141,0.957142857142856,0.97142857142857,
1.),.UNSPECIFIED.);
#178=B_SPLINE_CURVE_WITH_KNOTS('',3,(#17444,#17445,#17446,#17447,#17448,
#17449,#17450,#17451,#17452,#17453,#17454,#17455,#17456,#17457,#17458,#17459,
#17460,#17461,#17462,#17463,#17464,#17465,#17466,#17467,#17468,#17469,#17470,
#17471,#17472,#17473,#17474,#17475,#17476,#17477,#17478,#17479,#17480,#17481,
#17482,#17483,#17484,#17485,#17486,#17487,#17488,#17489,#17490,#17491,#17492,
#17493,#17494,#17495,#17496,#17497,#17498,#17499,#17500,#17501,#17502,#17503,
#17504,#17505,#17506,#17507,#17508,#17509,#17510,#17511,#17512,#17513),
 .UNSPECIFIED.,.F.,.F.,(4,3,3,3,3,3,3,3,3,3,3,3,3,3,3,3,3,3,3,3,3,3,3,4),
(-0.411449009780156,-0.40550489541351,-0.398537948778872,-0.388735121435802,
-0.382214695237718,-0.375350877814336,-0.367728232837723,-0.356236725561544,
-0.347888396755939,-0.337683279648765,-0.326660059466727,-0.316483474375939,
-0.302658061023146,-0.289316835726674,-0.271192407480734,-0.255261428970096,
-0.231775298750333,-0.202135573344553,-0.161986280154224,-0.126192133975022,
-0.0754619861897902,-0.0360560078842204,-0.00196685499849691,0.),
 .UNSPECIFIED.);
#179=B_SPLINE_CURVE_WITH_KNOTS('',5,(#17665,#17666,#17667,#17668,#17669,
#17670,#17671,#17672,#17673,#17674,#17675,#17676,#17677,#17678,#17679,#17680,
#17681,#17682,#17683,#17684,#17685,#17686,#17687,#17688,#17689,#17690,#17691,
#17692,#17693,#17694,#17695,#17696,#17697,#17698,#17699,#17700,#17701,#17702,
#17703,#17704,#17705,#17706,#17707,#17708,#17709,#17710,#17711,#17712,#17713,
#17714,#17715,#17716,#17717,#17718,#17719,#17720,#17721,#17722,#17723,#17724,
#17725,#17726,#17727,#17728,#17729,#17730,#17731,#17732,#17733,#17734,#17735,
#17736,#17737,#17738),.UNSPECIFIED.,.F.,.F.,(6,1,1,1,1,1,1,1,1,1,1,1,1,
1,1,1,1,1,1,1,1,1,1,1,1,1,1,1,1,1,1,1,1,1,1,1,1,1,1,1,1,1,1,1,1,1,1,1,1,
1,1,1,1,1,1,1,1,1,1,1,1,1,1,1,1,1,1,1,1,6),(0.,0.0142857142857143,0.0285714285714286,
0.0428571428571429,0.0571428571428571,0.0714285714285714,0.0857142857142857,
0.1,0.114285714285714,0.128571428571429,0.142857142857143,0.157142857142857,
0.171428571428571,0.185714285714286,0.2,0.214285714285714,0.228571428571429,
0.242857142857143,0.257142857142857,0.271428571428571,0.285714285714286,
0.3,0.314285714285714,0.328571428571429,0.342857142857143,0.357142857142857,
0.371428571428571,0.385714285714286,0.4,0.414285714285714,0.428571428571429,
0.442857142857143,0.457142857142857,0.471428571428572,0.485714285714286,
0.5,0.514285714285714,0.528571428571429,0.542857142857143,0.557142857142857,
0.571428571428571,0.585714285714286,0.6,0.614285714285714,0.628571428571428,
0.642857142857142,0.657142857142857,0.671428571428571,0.685714285714285,
0.699999999999999,0.714285714285714,0.728571428571428,0.742857142857142,
0.757142857142856,0.771428571428571,0.785714285714285,0.799999999999999,
0.814285714285713,0.828571428571428,0.842857142857142,0.857142857142856,
0.87142857142857,0.885714285714284,0.899999999999999,0.914285714285713,
0.928571428571427,0.942857142857141,0.957142857142856,0.97142857142857,
1.),.UNSPECIFIED.);
#180=B_SPLINE_CURVE_WITH_KNOTS('',3,(#17740,#17741,#17742,#17743,#17744,
#17745,#17746,#17747,#17748,#17749,#17750,#17751,#17752,#17753,#17754,#17755,
#17756,#17757,#17758,#17759,#17760,#17761,#17762,#17763,#17764,#17765,#17766,
#17767,#17768,#17769,#17770,#17771,#17772,#17773,#17774,#17775,#17776,#17777,
#17778,#17779,#17780,#17781,#17782,#17783,#17784,#17785,#17786,#17787,#17788,
#17789,#17790,#17791,#17792,#17793,#17794,#17795,#17796,#17797,#17798,#17799,
#17800,#17801,#17802,#17803,#17804,#17805,#17806),.UNSPECIFIED.,.F.,.F.,
(4,3,3,3,3,3,3,3,3,3,3,3,3,3,3,3,3,3,3,3,3,3,4),(-0.0308474254356243,-0.0282443139231585,
-0.0239308456686803,-0.0206152610248062,-0.0170461143320954,-0.0150701375499139,
-0.0131660090736057,-0.011520257939405,-0.0103391768235893,-0.00917732810571033,
-0.00816993701950823,-0.00725747185266823,-0.00648885938409023,-0.00537659348121548,
-0.00470451929606354,-0.00408467782751111,-0.00323202309648034,-0.00269108370976756,
-0.0022056157890913,-0.00169529231892506,-0.000847646159462529,-0.000380223901454506,
0.),.UNSPECIFIED.);
#181=B_SPLINE_CURVE_WITH_KNOTS('',5,(#17964,#17965,#17966,#17967,#17968,
#17969,#17970,#17971,#17972,#17973,#17974,#17975,#17976,#17977,#17978,#17979,
#17980,#17981,#17982,#17983,#17984,#17985,#17986,#17987,#17988,#17989,#17990,
#17991,#17992,#17993,#17994,#17995,#17996,#17997,#17998,#17999,#18000,#18001,
#18002,#18003,#18004,#18005,#18006,#18007,#18008,#18009,#18010,#18011,#18012,
#18013,#18014,#18015,#18016,#18017,#18018,#18019,#18020,#18021,#18022,#18023,
#18024,#18025,#18026,#18027,#18028,#18029,#18030,#18031,#18032,#18033,#18034,
#18035,#18036,#18037),.UNSPECIFIED.,.F.,.F.,(6,1,1,1,1,1,1,1,1,1,1,1,1,
1,1,1,1,1,1,1,1,1,1,1,1,1,1,1,1,1,1,1,1,1,1,1,1,1,1,1,1,1,1,1,1,1,1,1,1,
1,1,1,1,1,1,1,1,1,1,1,1,1,1,1,1,1,1,1,1,6),(0.,0.0142857142857143,0.0285714285714286,
0.0428571428571429,0.0571428571428571,0.0714285714285714,0.0857142857142857,
0.1,0.114285714285714,0.128571428571429,0.142857142857143,0.157142857142857,
0.171428571428571,0.185714285714286,0.2,0.214285714285714,0.228571428571429,
0.242857142857143,0.257142857142857,0.271428571428571,0.285714285714286,
0.3,0.314285714285714,0.328571428571429,0.342857142857143,0.357142857142857,
0.371428571428571,0.385714285714286,0.4,0.414285714285714,0.428571428571429,
0.442857142857143,0.457142857142857,0.471428571428572,0.485714285714286,
0.5,0.514285714285714,0.528571428571429,0.542857142857143,0.557142857142857,
0.571428571428571,0.585714285714286,0.6,0.614285714285714,0.628571428571428,
0.642857142857142,0.657142857142857,0.671428571428571,0.685714285714285,
0.699999999999999,0.714285714285714,0.728571428571428,0.742857142857142,
0.757142857142856,0.771428571428571,0.785714285714285,0.799999999999999,
0.814285714285713,0.828571428571428,0.842857142857142,0.857142857142856,
0.87142857142857,0.885714285714284,0.899999999999999,0.914285714285713,
0.928571428571427,0.942857142857141,0.957142857142856,0.97142857142857,
1.),.UNSPECIFIED.);
#182=B_SPLINE_CURVE_WITH_KNOTS('',3,(#18038,#18039,#18040,#18041,#18042,
#18043,#18044,#18045,#18046,#18047,#18048,#18049,#18050,#18051,#18052,#18053,
#18054,#18055,#18056,#18057,#18058,#18059,#18060,#18061,#18062,#18063,#18064,
#18065,#18066,#18067,#18068,#18069,#18070,#18071,#18072,#18073,#18074,#18075,
#18076,#18077,#18078,#18079,#18080,#18081,#18082,#18083,#18084,#18085,#18086,
#18087,#18088,#18089,#18090,#18091,#18092,#18093,#18094,#18095,#18096,#18097,
#18098,#18099,#18100,#18101,#18102,#18103,#18104,#18105,#18106,#18107),
 .UNSPECIFIED.,.F.,.F.,(4,3,3,3,3,3,3,3,3,3,3,3,3,3,3,3,3,3,3,3,3,3,3,4),
(-0.411449009963507,-0.40550489558343,-0.398537948945618,-0.388735121610794,
-0.382214695410633,-0.375350877984368,-0.367728233004637,-0.356236725723242,
-0.347888396914042,-0.337683279795922,-0.326660059606393,-0.316483474513951,
-0.302658061166432,-0.289316835878854,-0.27119240761099,-0.255261429176367,
-0.231775298979734,-0.202135573634019,-0.1619862806212,-0.126192134288906,
-0.0754619859378416,-0.0360560139109727,-0.0019668740044922,0.),
 .UNSPECIFIED.);
#183=B_SPLINE_CURVE_WITH_KNOTS('',5,(#18259,#18260,#18261,#18262,#18263,
#18264,#18265,#18266,#18267,#18268,#18269,#18270,#18271,#18272,#18273,#18274,
#18275,#18276,#18277,#18278,#18279,#18280,#18281,#18282,#18283,#18284,#18285,
#18286,#18287,#18288,#18289,#18290,#18291,#18292,#18293,#18294,#18295,#18296,
#18297,#18298,#18299,#18300,#18301,#18302,#18303,#18304,#18305,#18306,#18307,
#18308,#18309,#18310,#18311,#18312,#18313,#18314,#18315,#18316,#18317,#18318,
#18319,#18320,#18321,#18322,#18323,#18324,#18325,#18326,#18327,#18328,#18329,
#18330,#18331,#18332),.UNSPECIFIED.,.F.,.F.,(6,1,1,1,1,1,1,1,1,1,1,1,1,
1,1,1,1,1,1,1,1,1,1,1,1,1,1,1,1,1,1,1,1,1,1,1,1,1,1,1,1,1,1,1,1,1,1,1,1,
1,1,1,1,1,1,1,1,1,1,1,1,1,1,1,1,1,1,1,1,6),(0.,0.0142857142857143,0.0285714285714286,
0.0428571428571429,0.0571428571428571,0.0714285714285714,0.0857142857142857,
0.1,0.114285714285714,0.128571428571429,0.142857142857143,0.157142857142857,
0.171428571428571,0.185714285714286,0.2,0.214285714285714,0.228571428571429,
0.242857142857143,0.257142857142857,0.271428571428571,0.285714285714286,
0.3,0.314285714285714,0.328571428571429,0.342857142857143,0.357142857142857,
0.371428571428571,0.385714285714286,0.4,0.414285714285714,0.428571428571429,
0.442857142857143,0.457142857142857,0.471428571428572,0.485714285714286,
0.5,0.514285714285714,0.528571428571429,0.542857142857143,0.557142857142857,
0.571428571428571,0.585714285714286,0.6,0.614285714285714,0.628571428571428,
0.642857142857142,0.657142857142857,0.671428571428571,0.685714285714285,
0.699999999999999,0.714285714285714,0.728571428571428,0.742857142857142,
0.757142857142856,0.771428571428571,0.785714285714285,0.799999999999999,
0.814285714285713,0.828571428571428,0.842857142857142,0.857142857142856,
0.87142857142857,0.885714285714284,0.899999999999999,0.914285714285713,
0.928571428571427,0.942857142857141,0.957142857142856,0.97142857142857,
1.),.UNSPECIFIED.);
#184=B_SPLINE_CURVE_WITH_KNOTS('',3,(#18334,#18335,#18336,#18337,#18338,
#18339,#18340,#18341,#18342,#18343,#18344,#18345,#18346,#18347,#18348,#18349,
#18350,#18351,#18352,#18353,#18354,#18355,#18356,#18357,#18358,#18359,#18360,
#18361,#18362,#18363,#18364,#18365,#18366,#18367,#18368,#18369,#18370,#18371,
#18372,#18373,#18374,#18375,#18376,#18377,#18378,#18379,#18380,#18381,#18382,
#18383,#18384,#18385,#18386,#18387,#18388,#18389,#18390,#18391,#18392,#18393,
#18394,#18395,#18396,#18397,#18398,#18399,#18400),.UNSPECIFIED.,.F.,.F.,
(4,3,3,3,3,3,3,3,3,3,3,3,3,3,3,3,3,3,3,3,3,3,4),(-0.030847425423351,-0.0282443142621516,
-0.0239308460522739,-0.0206152614247573,-0.0170461144001592,-0.0150701376854405,
-0.0131660090123514,-0.0115202578858075,-0.0103391767661309,-0.00917732807723113,
-0.00816993700701968,-0.0072574718323543,-0.00648885936596464,-0.00537659349330486,
-0.00470451930664176,-0.00408467783955803,-0.00323202308982742,-0.00269108370404856,
-0.00220561578379538,-0.00169529231302908,-0.000847646156514541,-0.000380223899127519,
0.),.UNSPECIFIED.);
#185=B_SPLINE_CURVE_WITH_KNOTS('',5,(#18558,#18559,#18560,#18561,#18562,
#18563,#18564,#18565,#18566,#18567,#18568,#18569,#18570,#18571,#18572,#18573,
#18574,#18575,#18576,#18577,#18578,#18579,#18580,#18581,#18582,#18583,#18584,
#18585,#18586,#18587,#18588,#18589,#18590,#18591,#18592,#18593,#18594,#18595,
#18596,#18597,#18598,#18599,#18600,#18601,#18602,#18603,#18604,#18605,#18606,
#18607,#18608,#18609,#18610,#18611,#18612,#18613,#18614,#18615,#18616,#18617,
#18618,#18619,#18620,#18621,#18622,#18623,#18624,#18625,#18626,#18627,#18628,
#18629,#18630,#18631),.UNSPECIFIED.,.F.,.F.,(6,1,1,1,1,1,1,1,1,1,1,1,1,
1,1,1,1,1,1,1,1,1,1,1,1,1,1,1,1,1,1,1,1,1,1,1,1,1,1,1,1,1,1,1,1,1,1,1,1,
1,1,1,1,1,1,1,1,1,1,1,1,1,1,1,1,1,1,1,1,6),(0.,0.0142857142857143,0.0285714285714286,
0.0428571428571429,0.0571428571428571,0.0714285714285714,0.0857142857142857,
0.1,0.114285714285714,0.128571428571429,0.142857142857143,0.157142857142857,
0.171428571428571,0.185714285714286,0.2,0.214285714285714,0.228571428571429,
0.242857142857143,0.257142857142857,0.271428571428571,0.285714285714286,
0.3,0.314285714285714,0.328571428571429,0.342857142857143,0.357142857142857,
0.371428571428571,0.385714285714286,0.4,0.414285714285714,0.428571428571429,
0.442857142857143,0.457142857142857,0.471428571428572,0.485714285714286,
0.5,0.514285714285714,0.528571428571429,0.542857142857143,0.557142857142857,
0.571428571428571,0.585714285714286,0.6,0.614285714285714,0.628571428571428,
0.642857142857142,0.657142857142857,0.671428571428571,0.685714285714285,
0.699999999999999,0.714285714285714,0.728571428571428,0.742857142857142,
0.757142857142856,0.771428571428571,0.785714285714285,0.799999999999999,
0.814285714285713,0.828571428571428,0.842857142857142,0.857142857142856,
0.87142857142857,0.885714285714284,0.899999999999999,0.914285714285713,
0.928571428571427,0.942857142857141,0.957142857142856,0.97142857142857,
1.),.UNSPECIFIED.);
#186=B_SPLINE_CURVE_WITH_KNOTS('',3,(#18632,#18633,#18634,#18635,#18636,
#18637,#18638,#18639,#18640,#18641,#18642,#18643,#18644,#18645,#18646,#18647,
#18648,#18649,#18650,#18651,#18652,#18653,#18654,#18655,#18656,#18657,#18658,
#18659,#18660,#18661,#18662,#18663,#18664,#18665,#18666,#18667,#18668,#18669,
#18670,#18671,#18672,#18673,#18674,#18675,#18676,#18677,#18678,#18679,#18680,
#18681,#18682,#18683,#18684,#18685,#18686,#18687,#18688,#18689,#18690,#18691,
#18692,#18693,#18694,#18695,#18696,#18697,#18698,#18699,#18700,#18701),
 .UNSPECIFIED.,.F.,.F.,(4,3,3,3,3,3,3,3,3,3,3,3,3,3,3,3,3,3,3,3,3,3,3,4),
(-0.411449009976945,-0.405504895592072,-0.398537948953833,-0.388735121623208,
-0.382214695422447,-0.375350877996945,-0.367728233016586,-0.356236725734817,
-0.347888396925664,-0.337683279812359,-0.326660059622673,-0.31648347452754,
-0.302658061159068,-0.289316835870757,-0.271192407500547,-0.255261428976667,
-0.231775298862027,-0.202135573483824,-0.16198628029512,-0.126192133881173,
-0.0754619854549211,-0.0360560096240121,-0.00196686195736208,0.),
 .UNSPECIFIED.);
#187=B_SPLINE_CURVE_WITH_KNOTS('',5,(#18727,#18728,#18729,#18730,#18731,
#18732,#18733,#18734,#18735,#18736,#18737,#18738,#18739,#18740,#18741,#18742,
#18743,#18744,#18745,#18746,#18747,#18748,#18749,#18750,#18751,#18752,#18753,
#18754,#18755,#18756,#18757,#18758,#18759,#18760,#18761,#18762,#18763,#18764,
#18765,#18766,#18767,#18768,#18769,#18770,#18771,#18772,#18773,#18774,#18775,
#18776,#18777,#18778,#18779,#18780,#18781,#18782,#18783,#18784,#18785,#18786,
#18787,#18788,#18789,#18790,#18791,#18792,#18793,#18794,#18795,#18796,#18797,
#18798,#18799,#18800),.UNSPECIFIED.,.F.,.F.,(6,1,1,1,1,1,1,1,1,1,1,1,1,
1,1,1,1,1,1,1,1,1,1,1,1,1,1,1,1,1,1,1,1,1,1,1,1,1,1,1,1,1,1,1,1,1,1,1,1,
1,1,1,1,1,1,1,1,1,1,1,1,1,1,1,1,1,1,1,1,6),(0.,0.0142857142857143,0.0285714285714286,
0.0428571428571429,0.0571428571428571,0.0714285714285714,0.0857142857142857,
0.1,0.114285714285714,0.128571428571429,0.142857142857143,0.157142857142857,
0.171428571428571,0.185714285714286,0.2,0.214285714285714,0.228571428571429,
0.242857142857143,0.257142857142857,0.271428571428571,0.285714285714286,
0.3,0.314285714285714,0.328571428571429,0.342857142857143,0.357142857142857,
0.371428571428571,0.385714285714286,0.4,0.414285714285714,0.428571428571429,
0.442857142857143,0.457142857142857,0.471428571428572,0.485714285714286,
0.5,0.514285714285714,0.528571428571429,0.542857142857143,0.557142857142857,
0.571428571428571,0.585714285714286,0.6,0.614285714285714,0.628571428571428,
0.642857142857142,0.657142857142857,0.671428571428571,0.685714285714285,
0.699999999999999,0.714285714285714,0.728571428571428,0.742857142857142,
0.757142857142856,0.771428571428571,0.785714285714285,0.799999999999999,
0.814285714285713,0.828571428571428,0.842857142857142,0.857142857142856,
0.87142857142857,0.885714285714284,0.899999999999999,0.914285714285713,
0.928571428571427,0.942857142857141,0.957142857142856,0.97142857142857,
1.),.UNSPECIFIED.);
#188=B_SPLINE_CURVE_WITH_KNOTS('',5,(#18804,#18805,#18806,#18807,#18808,
#18809,#18810,#18811,#18812,#18813,#18814,#18815,#18816,#18817,#18818,#18819,
#18820,#18821,#18822,#18823,#18824,#18825,#18826,#18827,#18828,#18829,#18830,
#18831,#18832,#18833,#18834,#18835,#18836,#18837,#18838,#18839,#18840,#18841,
#18842,#18843,#18844,#18845,#18846,#18847,#18848,#18849,#18850,#18851,#18852,
#18853,#18854,#18855,#18856,#18857,#18858,#18859,#18860,#18861,#18862,#18863,
#18864,#18865,#18866,#18867,#18868,#18869,#18870,#18871,#18872,#18873,#18874,
#18875,#18876,#18877),.UNSPECIFIED.,.F.,.F.,(6,1,1,1,1,1,1,1,1,1,1,1,1,
1,1,1,1,1,1,1,1,1,1,1,1,1,1,1,1,1,1,1,1,1,1,1,1,1,1,1,1,1,1,1,1,1,1,1,1,
1,1,1,1,1,1,1,1,1,1,1,1,1,1,1,1,1,1,1,1,6),(0.,0.0142857142857143,0.0285714285714286,
0.0428571428571429,0.0571428571428571,0.0714285714285714,0.0857142857142857,
0.1,0.114285714285714,0.128571428571429,0.142857142857143,0.157142857142857,
0.171428571428571,0.185714285714286,0.2,0.214285714285714,0.228571428571429,
0.242857142857143,0.257142857142857,0.271428571428571,0.285714285714286,
0.3,0.314285714285714,0.328571428571429,0.342857142857143,0.357142857142857,
0.371428571428571,0.385714285714286,0.4,0.414285714285714,0.428571428571429,
0.442857142857143,0.457142857142857,0.471428571428572,0.485714285714286,
0.5,0.514285714285714,0.528571428571429,0.542857142857143,0.557142857142857,
0.571428571428571,0.585714285714286,0.6,0.614285714285714,0.628571428571428,
0.642857142857142,0.657142857142857,0.671428571428571,0.685714285714285,
0.699999999999999,0.714285714285714,0.728571428571428,0.742857142857142,
0.757142857142856,0.771428571428571,0.785714285714285,0.799999999999999,
0.814285714285713,0.828571428571428,0.842857142857142,0.857142857142856,
0.87142857142857,0.885714285714284,0.899999999999999,0.914285714285713,
0.928571428571427,0.942857142857141,0.957142857142856,0.97142857142857,
1.),.UNSPECIFIED.);
#189=B_SPLINE_CURVE_WITH_KNOTS('',3,(#18892,#18893,#18894,#18895,#18896,
#18897,#18898,#18899,#18900,#18901,#18902,#18903,#18904,#18905,#18906,#18907,
#18908,#18909,#18910,#18911,#18912,#18913,#18914,#18915,#18916,#18917,#18918,
#18919,#18920,#18921,#18922,#18923,#18924,#18925,#18926,#18927,#18928,#18929,
#18930,#18931,#18932,#18933,#18934,#18935,#18936,#18937,#18938,#18939,#18940,
#18941,#18942,#18943,#18944,#18945,#18946,#18947,#18948,#18949,#18950,#18951,
#18952,#18953,#18954,#18955,#18956,#18957,#18958,#18959,#18960,#18961),
 .UNSPECIFIED.,.F.,.F.,(4,3,3,3,3,3,3,3,3,3,3,3,3,3,3,3,3,3,3,3,3,3,3,4),
(-0.411449009793068,-0.405504895416512,-0.398537948781067,-0.38873512144739,
-0.382214695249858,-0.375350877826228,-0.367728232848294,-0.356236725571785,
-0.347888396766066,-0.33768327965463,-0.326660059470826,-0.316483474377544,
-0.302658061011095,-0.289316835715289,-0.271192407328683,-0.255261428798271,
-0.23177529872749,-0.202135573370612,-0.161986280260425,-0.126192134080337,
-0.075461985655617,-0.0360560111852818,-0.00196686554572469,0.),
 .UNSPECIFIED.);
#190=B_SPLINE_CURVE_WITH_KNOTS('',3,(#18965,#18966,#18967,#18968,#18969,
#18970,#18971,#18972,#18973,#18974,#18975,#18976,#18977,#18978,#18979,#18980,
#18981,#18982,#18983,#18984,#18985,#18986,#18987,#18988,#18989,#18990,#18991,
#18992,#18993,#18994,#18995,#18996,#18997,#18998,#18999,#19000,#19001,#19002,
#19003,#19004,#19005,#19006,#19007,#19008,#19009,#19010,#19011,#19012,#19013,
#19014,#19015,#19016,#19017,#19018,#19019,#19020,#19021,#19022,#19023,#19024,
#19025,#19026,#19027,#19028,#19029,#19030,#19031),.UNSPECIFIED.,.F.,.F.,
(4,3,3,3,3,3,3,3,3,3,3,3,3,3,3,3,3,3,3,3,3,3,4),(-0.03084742543048,-0.0282443142384382,
-0.0239308460027108,-0.0206152613738073,-0.0170461144147563,-0.0150701377170469,
-0.0131660090069468,-0.0115202578810785,-0.0103391767598669,-0.00917732807488943,
-0.00816993700694134,-0.00725747182913227,-0.00648885936321739,-0.00537659349882703,
-0.00470451931147365,-0.00408467784459405,-0.00323202308945096,-0.00269108370363151,
-0.00220561578335159,-0.00169529231220793,-0.000847646156103964,-0.000380223898199378,
0.),.UNSPECIFIED.);
#191=B_SPLINE_SURFACE_WITH_KNOTS('',5,1,((#7395,#7396),(#7397,#7398),(#7399,
#7400),(#7401,#7402),(#7403,#7404),(#7405,#7406),(#7407,#7408),(#7409,#7410),
(#7411,#7412),(#7413,#7414),(#7415,#7416),(#7417,#7418),(#7419,#7420),(#7421,
#7422),(#7423,#7424),(#7425,#7426),(#7427,#7428),(#7429,#7430),(#7431,#7432),
(#7433,#7434),(#7435,#7436),(#7437,#7438),(#7439,#7440),(#7441,#7442),(#7443,
#7444),(#7445,#7446),(#7447,#7448),(#7449,#7450),(#7451,#7452),(#7453,#7454),
(#7455,#7456),(#7457,#7458),(#7459,#7460),(#7461,#7462),(#7463,#7464),(#7465,
#7466),(#7467,#7468),(#7469,#7470),(#7471,#7472),(#7473,#7474),(#7475,#7476),
(#7477,#7478),(#7479,#7480),(#7481,#7482),(#7483,#7484),(#7485,#7486),(#7487,
#7488),(#7489,#7490),(#7491,#7492),(#7493,#7494),(#7495,#7496),(#7497,#7498),
(#7499,#7500),(#7501,#7502),(#7503,#7504),(#7505,#7506),(#7507,#7508),(#7509,
#7510),(#7511,#7512),(#7513,#7514),(#7515,#7516),(#7517,#7518),(#7519,#7520),
(#7521,#7522),(#7523,#7524),(#7525,#7526),(#7527,#7528),(#7529,#7530),(#7531,
#7532),(#7533,#7534),(#7535,#7536),(#7537,#7538),(#7539,#7540),(#7541,#7542),
(#7543,#7544)),.UNSPECIFIED.,.F.,.F.,.F.,(6,1,1,1,1,1,1,1,1,1,1,1,1,1,1,
1,1,1,1,1,1,1,1,1,1,1,1,1,1,1,1,1,1,1,1,1,1,1,1,1,1,1,1,1,1,1,1,1,1,1,1,
1,1,1,1,1,1,1,1,1,1,1,1,1,1,1,1,1,1,1,6),(2,2),(-1.,-0.985714285714284,
-0.97142857142857,-0.957142857142856,-0.942857142857141,-0.928571428571427,
-0.914285714285713,-0.899999999999999,-0.885714285714284,-0.87142857142857,
-0.857142857142856,-0.842857142857142,-0.828571428571428,-0.814285714285713,
-0.799999999999999,-0.785714285714285,-0.771428571428571,-0.757142857142856,
-0.742857142857142,-0.728571428571428,-0.714285714285714,-0.699999999999999,
-0.685714285714285,-0.671428571428571,-0.657142857142857,-0.642857142857142,
-0.628571428571428,-0.614285714285714,-0.6,-0.585714285714286,-0.571428571428571,
-0.557142857142857,-0.542857142857143,-0.528571428571429,-0.514285714285714,
-0.5,-0.485714285714286,-0.471428571428572,-0.457142857142857,-0.442857142857143,
-0.428571428571429,-0.414285714285714,-0.4,-0.385714285714286,-0.371428571428571,
-0.357142857142857,-0.342857142857143,-0.328571428571429,-0.314285714285714,
-0.3,-0.285714285714286,-0.271428571428571,-0.257142857142857,-0.242857142857143,
-0.228571428571429,-0.214285714285714,-0.2,-0.185714285714286,-0.171428571428571,
-0.157142857142857,-0.142857142857143,-0.128571428571429,-0.114285714285714,
-0.1,-0.0857142857142857,-0.0714285714285714,-0.0571428571428571,-0.0428571428571429,
-0.0285714285714286,-0.0142857142857143,0.),(0.,2.1),.UNSPECIFIED.);
#192=B_SPLINE_SURFACE_WITH_KNOTS('',5,1,((#7695,#7696),(#7697,#7698),(#7699,
#7700),(#7701,#7702),(#7703,#7704),(#7705,#7706),(#7707,#7708),(#7709,#7710),
(#7711,#7712),(#7713,#7714),(#7715,#7716),(#7717,#7718),(#7719,#7720),(#7721,
#7722),(#7723,#7724),(#7725,#7726),(#7727,#7728),(#7729,#7730),(#7731,#7732),
(#7733,#7734),(#7735,#7736),(#7737,#7738),(#7739,#7740),(#7741,#7742),(#7743,
#7744),(#7745,#7746),(#7747,#7748),(#7749,#7750),(#7751,#7752),(#7753,#7754),
(#7755,#7756),(#7757,#7758),(#7759,#7760),(#7761,#7762),(#7763,#7764),(#7765,
#7766),(#7767,#7768),(#7769,#7770),(#7771,#7772),(#7773,#7774),(#7775,#7776),
(#7777,#7778),(#7779,#7780),(#7781,#7782),(#7783,#7784),(#7785,#7786),(#7787,
#7788),(#7789,#7790),(#7791,#7792),(#7793,#7794),(#7795,#7796),(#7797,#7798),
(#7799,#7800),(#7801,#7802),(#7803,#7804),(#7805,#7806),(#7807,#7808),(#7809,
#7810),(#7811,#7812),(#7813,#7814),(#7815,#7816),(#7817,#7818),(#7819,#7820),
(#7821,#7822),(#7823,#7824),(#7825,#7826),(#7827,#7828),(#7829,#7830),(#7831,
#7832),(#7833,#7834),(#7835,#7836),(#7837,#7838),(#7839,#7840),(#7841,#7842),
(#7843,#7844)),.UNSPECIFIED.,.F.,.F.,.F.,(6,1,1,1,1,1,1,1,1,1,1,1,1,1,1,
1,1,1,1,1,1,1,1,1,1,1,1,1,1,1,1,1,1,1,1,1,1,1,1,1,1,1,1,1,1,1,1,1,1,1,1,
1,1,1,1,1,1,1,1,1,1,1,1,1,1,1,1,1,1,1,6),(2,2),(0.,0.0142857142857143,0.0285714285714286,
0.0428571428571429,0.0571428571428571,0.0714285714285714,0.0857142857142857,
0.1,0.114285714285714,0.128571428571429,0.142857142857143,0.157142857142857,
0.171428571428571,0.185714285714286,0.2,0.214285714285714,0.228571428571429,
0.242857142857143,0.257142857142857,0.271428571428571,0.285714285714286,
0.3,0.314285714285714,0.328571428571429,0.342857142857143,0.357142857142857,
0.371428571428571,0.385714285714286,0.4,0.414285714285714,0.428571428571429,
0.442857142857143,0.457142857142857,0.471428571428572,0.485714285714286,
0.5,0.514285714285714,0.528571428571429,0.542857142857143,0.557142857142857,
0.571428571428571,0.585714285714286,0.6,0.614285714285714,0.628571428571428,
0.642857142857142,0.657142857142857,0.671428571428571,0.685714285714285,
0.699999999999999,0.714285714285714,0.728571428571428,0.742857142857142,
0.757142857142856,0.771428571428571,0.785714285714285,0.799999999999999,
0.814285714285713,0.828571428571428,0.842857142857142,0.857142857142856,
0.87142857142857,0.885714285714284,0.899999999999999,0.914285714285713,
0.928571428571427,0.942857142857141,0.957142857142856,0.97142857142857,
0.985714285714284,1.),(0.,2.1),.UNSPECIFIED.);
#193=B_SPLINE_SURFACE_WITH_KNOTS('',5,1,((#7989,#7990),(#7991,#7992),(#7993,
#7994),(#7995,#7996),(#7997,#7998),(#7999,#8000),(#8001,#8002),(#8003,#8004),
(#8005,#8006),(#8007,#8008),(#8009,#8010),(#8011,#8012),(#8013,#8014),(#8015,
#8016),(#8017,#8018),(#8019,#8020),(#8021,#8022),(#8023,#8024),(#8025,#8026),
(#8027,#8028),(#8029,#8030),(#8031,#8032),(#8033,#8034),(#8035,#8036),(#8037,
#8038),(#8039,#8040),(#8041,#8042),(#8043,#8044),(#8045,#8046),(#8047,#8048),
(#8049,#8050),(#8051,#8052),(#8053,#8054),(#8055,#8056),(#8057,#8058),(#8059,
#8060),(#8061,#8062),(#8063,#8064),(#8065,#8066),(#8067,#8068),(#8069,#8070),
(#8071,#8072),(#8073,#8074),(#8075,#8076),(#8077,#8078),(#8079,#8080),(#8081,
#8082),(#8083,#8084),(#8085,#8086),(#8087,#8088),(#8089,#8090),(#8091,#8092),
(#8093,#8094),(#8095,#8096),(#8097,#8098),(#8099,#8100),(#8101,#8102),(#8103,
#8104),(#8105,#8106),(#8107,#8108),(#8109,#8110),(#8111,#8112),(#8113,#8114),
(#8115,#8116),(#8117,#8118),(#8119,#8120),(#8121,#8122),(#8123,#8124),(#8125,
#8126),(#8127,#8128),(#8129,#8130),(#8131,#8132),(#8133,#8134),(#8135,#8136),
(#8137,#8138)),.UNSPECIFIED.,.F.,.F.,.F.,(6,1,1,1,1,1,1,1,1,1,1,1,1,1,1,
1,1,1,1,1,1,1,1,1,1,1,1,1,1,1,1,1,1,1,1,1,1,1,1,1,1,1,1,1,1,1,1,1,1,1,1,
1,1,1,1,1,1,1,1,1,1,1,1,1,1,1,1,1,1,1,6),(2,2),(-1.,-0.985714285714284,
-0.97142857142857,-0.957142857142856,-0.942857142857141,-0.928571428571427,
-0.914285714285713,-0.899999999999999,-0.885714285714284,-0.87142857142857,
-0.857142857142856,-0.842857142857142,-0.828571428571428,-0.814285714285713,
-0.799999999999999,-0.785714285714285,-0.771428571428571,-0.757142857142856,
-0.742857142857142,-0.728571428571428,-0.714285714285714,-0.699999999999999,
-0.685714285714285,-0.671428571428571,-0.657142857142857,-0.642857142857142,
-0.628571428571428,-0.614285714285714,-0.6,-0.585714285714286,-0.571428571428571,
-0.557142857142857,-0.542857142857143,-0.528571428571429,-0.514285714285714,
-0.5,-0.485714285714286,-0.471428571428572,-0.457142857142857,-0.442857142857143,
-0.428571428571429,-0.414285714285714,-0.4,-0.385714285714286,-0.371428571428571,
-0.357142857142857,-0.342857142857143,-0.328571428571429,-0.314285714285714,
-0.3,-0.285714285714286,-0.271428571428571,-0.257142857142857,-0.242857142857143,
-0.228571428571429,-0.214285714285714,-0.2,-0.185714285714286,-0.171428571428571,
-0.157142857142857,-0.142857142857143,-0.128571428571429,-0.114285714285714,
-0.1,-0.0857142857142857,-0.0714285714285714,-0.0571428571428571,-0.0428571428571429,
-0.0285714285714286,-0.0142857142857143,0.),(0.,2.1),.UNSPECIFIED.);
#194=B_SPLINE_SURFACE_WITH_KNOTS('',5,1,((#8289,#8290),(#8291,#8292),(#8293,
#8294),(#8295,#8296),(#8297,#8298),(#8299,#8300),(#8301,#8302),(#8303,#8304),
(#8305,#8306),(#8307,#8308),(#8309,#8310),(#8311,#8312),(#8313,#8314),(#8315,
#8316),(#8317,#8318),(#8319,#8320),(#8321,#8322),(#8323,#8324),(#8325,#8326),
(#8327,#8328),(#8329,#8330),(#8331,#8332),(#8333,#8334),(#8335,#8336),(#8337,
#8338),(#8339,#8340),(#8341,#8342),(#8343,#8344),(#8345,#8346),(#8347,#8348),
(#8349,#8350),(#8351,#8352),(#8353,#8354),(#8355,#8356),(#8357,#8358),(#8359,
#8360),(#8361,#8362),(#8363,#8364),(#8365,#8366),(#8367,#8368),(#8369,#8370),
(#8371,#8372),(#8373,#8374),(#8375,#8376),(#8377,#8378),(#8379,#8380),(#8381,
#8382),(#8383,#8384),(#8385,#8386),(#8387,#8388),(#8389,#8390),(#8391,#8392),
(#8393,#8394),(#8395,#8396),(#8397,#8398),(#8399,#8400),(#8401,#8402),(#8403,
#8404),(#8405,#8406),(#8407,#8408),(#8409,#8410),(#8411,#8412),(#8413,#8414),
(#8415,#8416),(#8417,#8418),(#8419,#8420),(#8421,#8422),(#8423,#8424),(#8425,
#8426),(#8427,#8428),(#8429,#8430),(#8431,#8432),(#8433,#8434),(#8435,#8436),
(#8437,#8438)),.UNSPECIFIED.,.F.,.F.,.F.,(6,1,1,1,1,1,1,1,1,1,1,1,1,1,1,
1,1,1,1,1,1,1,1,1,1,1,1,1,1,1,1,1,1,1,1,1,1,1,1,1,1,1,1,1,1,1,1,1,1,1,1,
1,1,1,1,1,1,1,1,1,1,1,1,1,1,1,1,1,1,1,6),(2,2),(0.,0.0142857142857143,0.0285714285714286,
0.0428571428571429,0.0571428571428571,0.0714285714285714,0.0857142857142857,
0.1,0.114285714285714,0.128571428571429,0.142857142857143,0.157142857142857,
0.171428571428571,0.185714285714286,0.2,0.214285714285714,0.228571428571429,
0.242857142857143,0.257142857142857,0.271428571428571,0.285714285714286,
0.3,0.314285714285714,0.328571428571429,0.342857142857143,0.357142857142857,
0.371428571428571,0.385714285714286,0.4,0.414285714285714,0.428571428571429,
0.442857142857143,0.457142857142857,0.471428571428572,0.485714285714286,
0.5,0.514285714285714,0.528571428571429,0.542857142857143,0.557142857142857,
0.571428571428571,0.585714285714286,0.6,0.614285714285714,0.628571428571428,
0.642857142857142,0.657142857142857,0.671428571428571,0.685714285714285,
0.699999999999999,0.714285714285714,0.728571428571428,0.742857142857142,
0.757142857142856,0.771428571428571,0.785714285714285,0.799999999999999,
0.814285714285713,0.828571428571428,0.842857142857142,0.857142857142856,
0.87142857142857,0.885714285714284,0.899999999999999,0.914285714285713,
0.928571428571427,0.942857142857141,0.957142857142856,0.97142857142857,
0.985714285714284,1.),(0.,2.1),.UNSPECIFIED.);
#195=B_SPLINE_SURFACE_WITH_KNOTS('',5,1,((#8589,#8590),(#8591,#8592),(#8593,
#8594),(#8595,#8596),(#8597,#8598),(#8599,#8600),(#8601,#8602),(#8603,#8604),
(#8605,#8606),(#8607,#8608),(#8609,#8610),(#8611,#8612),(#8613,#8614),(#8615,
#8616),(#8617,#8618),(#8619,#8620),(#8621,#8622),(#8623,#8624),(#8625,#8626),
(#8627,#8628),(#8629,#8630),(#8631,#8632),(#8633,#8634),(#8635,#8636),(#8637,
#8638),(#8639,#8640),(#8641,#8642),(#8643,#8644),(#8645,#8646),(#8647,#8648),
(#8649,#8650),(#8651,#8652),(#8653,#8654),(#8655,#8656),(#8657,#8658),(#8659,
#8660),(#8661,#8662),(#8663,#8664),(#8665,#8666),(#8667,#8668),(#8669,#8670),
(#8671,#8672),(#8673,#8674),(#8675,#8676),(#8677,#8678),(#8679,#8680),(#8681,
#8682),(#8683,#8684),(#8685,#8686),(#8687,#8688),(#8689,#8690),(#8691,#8692),
(#8693,#8694),(#8695,#8696),(#8697,#8698),(#8699,#8700),(#8701,#8702),(#8703,
#8704),(#8705,#8706),(#8707,#8708),(#8709,#8710),(#8711,#8712),(#8713,#8714),
(#8715,#8716),(#8717,#8718),(#8719,#8720),(#8721,#8722),(#8723,#8724),(#8725,
#8726),(#8727,#8728),(#8729,#8730),(#8731,#8732),(#8733,#8734),(#8735,#8736),
(#8737,#8738)),.UNSPECIFIED.,.F.,.F.,.F.,(6,1,1,1,1,1,1,1,1,1,1,1,1,1,1,
1,1,1,1,1,1,1,1,1,1,1,1,1,1,1,1,1,1,1,1,1,1,1,1,1,1,1,1,1,1,1,1,1,1,1,1,
1,1,1,1,1,1,1,1,1,1,1,1,1,1,1,1,1,1,1,6),(2,2),(-1.,-0.985714285714284,
-0.97142857142857,-0.957142857142856,-0.942857142857141,-0.928571428571427,
-0.914285714285713,-0.899999999999999,-0.885714285714284,-0.87142857142857,
-0.857142857142856,-0.842857142857142,-0.828571428571428,-0.814285714285713,
-0.799999999999999,-0.785714285714285,-0.771428571428571,-0.757142857142856,
-0.742857142857142,-0.728571428571428,-0.714285714285714,-0.699999999999999,
-0.685714285714285,-0.671428571428571,-0.657142857142857,-0.642857142857142,
-0.628571428571428,-0.614285714285714,-0.6,-0.585714285714286,-0.571428571428571,
-0.557142857142857,-0.542857142857143,-0.528571428571429,-0.514285714285714,
-0.5,-0.485714285714286,-0.471428571428572,-0.457142857142857,-0.442857142857143,
-0.428571428571429,-0.414285714285714,-0.4,-0.385714285714286,-0.371428571428571,
-0.357142857142857,-0.342857142857143,-0.328571428571429,-0.314285714285714,
-0.3,-0.285714285714286,-0.271428571428571,-0.257142857142857,-0.242857142857143,
-0.228571428571429,-0.214285714285714,-0.2,-0.185714285714286,-0.171428571428571,
-0.157142857142857,-0.142857142857143,-0.128571428571429,-0.114285714285714,
-0.1,-0.0857142857142857,-0.0714285714285714,-0.0571428571428571,-0.0428571428571429,
-0.0285714285714286,-0.0142857142857143,0.),(0.,2.1),.UNSPECIFIED.);
#196=B_SPLINE_SURFACE_WITH_KNOTS('',5,1,((#8889,#8890),(#8891,#8892),(#8893,
#8894),(#8895,#8896),(#8897,#8898),(#8899,#8900),(#8901,#8902),(#8903,#8904),
(#8905,#8906),(#8907,#8908),(#8909,#8910),(#8911,#8912),(#8913,#8914),(#8915,
#8916),(#8917,#8918),(#8919,#8920),(#8921,#8922),(#8923,#8924),(#8925,#8926),
(#8927,#8928),(#8929,#8930),(#8931,#8932),(#8933,#8934),(#8935,#8936),(#8937,
#8938),(#8939,#8940),(#8941,#8942),(#8943,#8944),(#8945,#8946),(#8947,#8948),
(#8949,#8950),(#8951,#8952),(#8953,#8954),(#8955,#8956),(#8957,#8958),(#8959,
#8960),(#8961,#8962),(#8963,#8964),(#8965,#8966),(#8967,#8968),(#8969,#8970),
(#8971,#8972),(#8973,#8974),(#8975,#8976),(#8977,#8978),(#8979,#8980),(#8981,
#8982),(#8983,#8984),(#8985,#8986),(#8987,#8988),(#8989,#8990),(#8991,#8992),
(#8993,#8994),(#8995,#8996),(#8997,#8998),(#8999,#9000),(#9001,#9002),(#9003,
#9004),(#9005,#9006),(#9007,#9008),(#9009,#9010),(#9011,#9012),(#9013,#9014),
(#9015,#9016),(#9017,#9018),(#9019,#9020),(#9021,#9022),(#9023,#9024),(#9025,
#9026),(#9027,#9028),(#9029,#9030),(#9031,#9032),(#9033,#9034),(#9035,#9036),
(#9037,#9038)),.UNSPECIFIED.,.F.,.F.,.F.,(6,1,1,1,1,1,1,1,1,1,1,1,1,1,1,
1,1,1,1,1,1,1,1,1,1,1,1,1,1,1,1,1,1,1,1,1,1,1,1,1,1,1,1,1,1,1,1,1,1,1,1,
1,1,1,1,1,1,1,1,1,1,1,1,1,1,1,1,1,1,1,6),(2,2),(0.,0.0142857142857143,0.0285714285714286,
0.0428571428571429,0.0571428571428571,0.0714285714285714,0.0857142857142857,
0.1,0.114285714285714,0.128571428571429,0.142857142857143,0.157142857142857,
0.171428571428571,0.185714285714286,0.2,0.214285714285714,0.228571428571429,
0.242857142857143,0.257142857142857,0.271428571428571,0.285714285714286,
0.3,0.314285714285714,0.328571428571429,0.342857142857143,0.357142857142857,
0.371428571428571,0.385714285714286,0.4,0.414285714285714,0.428571428571429,
0.442857142857143,0.457142857142857,0.471428571428572,0.485714285714286,
0.5,0.514285714285714,0.528571428571429,0.542857142857143,0.557142857142857,
0.571428571428571,0.585714285714286,0.6,0.614285714285714,0.628571428571428,
0.642857142857142,0.657142857142857,0.671428571428571,0.685714285714285,
0.699999999999999,0.714285714285714,0.728571428571428,0.742857142857142,
0.757142857142856,0.771428571428571,0.785714285714285,0.799999999999999,
0.814285714285713,0.828571428571428,0.842857142857142,0.857142857142856,
0.87142857142857,0.885714285714284,0.899999999999999,0.914285714285713,
0.928571428571427,0.942857142857141,0.957142857142856,0.97142857142857,
0.985714285714284,1.),(0.,2.1),.UNSPECIFIED.);
#197=B_SPLINE_SURFACE_WITH_KNOTS('',5,1,((#9183,#9184),(#9185,#9186),(#9187,
#9188),(#9189,#9190),(#9191,#9192),(#9193,#9194),(#9195,#9196),(#9197,#9198),
(#9199,#9200),(#9201,#9202),(#9203,#9204),(#9205,#9206),(#9207,#9208),(#9209,
#9210),(#9211,#9212),(#9213,#9214),(#9215,#9216),(#9217,#9218),(#9219,#9220),
(#9221,#9222),(#9223,#9224),(#9225,#9226),(#9227,#9228),(#9229,#9230),(#9231,
#9232),(#9233,#9234),(#9235,#9236),(#9237,#9238),(#9239,#9240),(#9241,#9242),
(#9243,#9244),(#9245,#9246),(#9247,#9248),(#9249,#9250),(#9251,#9252),(#9253,
#9254),(#9255,#9256),(#9257,#9258),(#9259,#9260),(#9261,#9262),(#9263,#9264),
(#9265,#9266),(#9267,#9268),(#9269,#9270),(#9271,#9272),(#9273,#9274),(#9275,
#9276),(#9277,#9278),(#9279,#9280),(#9281,#9282),(#9283,#9284),(#9285,#9286),
(#9287,#9288),(#9289,#9290),(#9291,#9292),(#9293,#9294),(#9295,#9296),(#9297,
#9298),(#9299,#9300),(#9301,#9302),(#9303,#9304),(#9305,#9306),(#9307,#9308),
(#9309,#9310),(#9311,#9312),(#9313,#9314),(#9315,#9316),(#9317,#9318),(#9319,
#9320),(#9321,#9322),(#9323,#9324),(#9325,#9326),(#9327,#9328),(#9329,#9330),
(#9331,#9332)),.UNSPECIFIED.,.F.,.F.,.F.,(6,1,1,1,1,1,1,1,1,1,1,1,1,1,1,
1,1,1,1,1,1,1,1,1,1,1,1,1,1,1,1,1,1,1,1,1,1,1,1,1,1,1,1,1,1,1,1,1,1,1,1,
1,1,1,1,1,1,1,1,1,1,1,1,1,1,1,1,1,1,1,6),(2,2),(-1.,-0.985714285714284,
-0.97142857142857,-0.957142857142856,-0.942857142857141,-0.928571428571427,
-0.914285714285713,-0.899999999999999,-0.885714285714284,-0.87142857142857,
-0.857142857142856,-0.842857142857142,-0.828571428571428,-0.814285714285713,
-0.799999999999999,-0.785714285714285,-0.771428571428571,-0.757142857142856,
-0.742857142857142,-0.728571428571428,-0.714285714285714,-0.699999999999999,
-0.685714285714285,-0.671428571428571,-0.657142857142857,-0.642857142857142,
-0.628571428571428,-0.614285714285714,-0.6,-0.585714285714286,-0.571428571428571,
-0.557142857142857,-0.542857142857143,-0.528571428571429,-0.514285714285714,
-0.5,-0.485714285714286,-0.471428571428572,-0.457142857142857,-0.442857142857143,
-0.428571428571429,-0.414285714285714,-0.4,-0.385714285714286,-0.371428571428571,
-0.357142857142857,-0.342857142857143,-0.328571428571429,-0.314285714285714,
-0.3,-0.285714285714286,-0.271428571428571,-0.257142857142857,-0.242857142857143,
-0.228571428571429,-0.214285714285714,-0.2,-0.185714285714286,-0.171428571428571,
-0.157142857142857,-0.142857142857143,-0.128571428571429,-0.114285714285714,
-0.1,-0.0857142857142857,-0.0714285714285714,-0.0571428571428571,-0.0428571428571429,
-0.0285714285714286,-0.0142857142857143,0.),(0.,2.1),.UNSPECIFIED.);
#198=B_SPLINE_SURFACE_WITH_KNOTS('',5,1,((#9483,#9484),(#9485,#9486),(#9487,
#9488),(#9489,#9490),(#9491,#9492),(#9493,#9494),(#9495,#9496),(#9497,#9498),
(#9499,#9500),(#9501,#9502),(#9503,#9504),(#9505,#9506),(#9507,#9508),(#9509,
#9510),(#9511,#9512),(#9513,#9514),(#9515,#9516),(#9517,#9518),(#9519,#9520),
(#9521,#9522),(#9523,#9524),(#9525,#9526),(#9527,#9528),(#9529,#9530),(#9531,
#9532),(#9533,#9534),(#9535,#9536),(#9537,#9538),(#9539,#9540),(#9541,#9542),
(#9543,#9544),(#9545,#9546),(#9547,#9548),(#9549,#9550),(#9551,#9552),(#9553,
#9554),(#9555,#9556),(#9557,#9558),(#9559,#9560),(#9561,#9562),(#9563,#9564),
(#9565,#9566),(#9567,#9568),(#9569,#9570),(#9571,#9572),(#9573,#9574),(#9575,
#9576),(#9577,#9578),(#9579,#9580),(#9581,#9582),(#9583,#9584),(#9585,#9586),
(#9587,#9588),(#9589,#9590),(#9591,#9592),(#9593,#9594),(#9595,#9596),(#9597,
#9598),(#9599,#9600),(#9601,#9602),(#9603,#9604),(#9605,#9606),(#9607,#9608),
(#9609,#9610),(#9611,#9612),(#9613,#9614),(#9615,#9616),(#9617,#9618),(#9619,
#9620),(#9621,#9622),(#9623,#9624),(#9625,#9626),(#9627,#9628),(#9629,#9630),
(#9631,#9632)),.UNSPECIFIED.,.F.,.F.,.F.,(6,1,1,1,1,1,1,1,1,1,1,1,1,1,1,
1,1,1,1,1,1,1,1,1,1,1,1,1,1,1,1,1,1,1,1,1,1,1,1,1,1,1,1,1,1,1,1,1,1,1,1,
1,1,1,1,1,1,1,1,1,1,1,1,1,1,1,1,1,1,1,6),(2,2),(0.,0.0142857142857143,0.0285714285714286,
0.0428571428571429,0.0571428571428571,0.0714285714285714,0.0857142857142857,
0.1,0.114285714285714,0.128571428571429,0.142857142857143,0.157142857142857,
0.171428571428571,0.185714285714286,0.2,0.214285714285714,0.228571428571429,
0.242857142857143,0.257142857142857,0.271428571428571,0.285714285714286,
0.3,0.314285714285714,0.328571428571429,0.342857142857143,0.357142857142857,
0.371428571428571,0.385714285714286,0.4,0.414285714285714,0.428571428571429,
0.442857142857143,0.457142857142857,0.471428571428572,0.485714285714286,
0.5,0.514285714285714,0.528571428571429,0.542857142857143,0.557142857142857,
0.571428571428571,0.585714285714286,0.6,0.614285714285714,0.628571428571428,
0.642857142857142,0.657142857142857,0.671428571428571,0.685714285714285,
0.699999999999999,0.714285714285714,0.728571428571428,0.742857142857142,
0.757142857142856,0.771428571428571,0.785714285714285,0.799999999999999,
0.814285714285713,0.828571428571428,0.842857142857142,0.857142857142856,
0.87142857142857,0.885714285714284,0.899999999999999,0.914285714285713,
0.928571428571427,0.942857142857141,0.957142857142856,0.97142857142857,
0.985714285714284,1.),(0.,2.1),.UNSPECIFIED.);
#199=B_SPLINE_SURFACE_WITH_KNOTS('',5,1,((#9777,#9778),(#9779,#9780),(#9781,
#9782),(#9783,#9784),(#9785,#9786),(#9787,#9788),(#9789,#9790),(#9791,#9792),
(#9793,#9794),(#9795,#9796),(#9797,#9798),(#9799,#9800),(#9801,#9802),(#9803,
#9804),(#9805,#9806),(#9807,#9808),(#9809,#9810),(#9811,#9812),(#9813,#9814),
(#9815,#9816),(#9817,#9818),(#9819,#9820),(#9821,#9822),(#9823,#9824),(#9825,
#9826),(#9827,#9828),(#9829,#9830),(#9831,#9832),(#9833,#9834),(#9835,#9836),
(#9837,#9838),(#9839,#9840),(#9841,#9842),(#9843,#9844),(#9845,#9846),(#9847,
#9848),(#9849,#9850),(#9851,#9852),(#9853,#9854),(#9855,#9856),(#9857,#9858),
(#9859,#9860),(#9861,#9862),(#9863,#9864),(#9865,#9866),(#9867,#9868),(#9869,
#9870),(#9871,#9872),(#9873,#9874),(#9875,#9876),(#9877,#9878),(#9879,#9880),
(#9881,#9882),(#9883,#9884),(#9885,#9886),(#9887,#9888),(#9889,#9890),(#9891,
#9892),(#9893,#9894),(#9895,#9896),(#9897,#9898),(#9899,#9900),(#9901,#9902),
(#9903,#9904),(#9905,#9906),(#9907,#9908),(#9909,#9910),(#9911,#9912),(#9913,
#9914),(#9915,#9916),(#9917,#9918),(#9919,#9920),(#9921,#9922),(#9923,#9924),
(#9925,#9926)),.UNSPECIFIED.,.F.,.F.,.F.,(6,1,1,1,1,1,1,1,1,1,1,1,1,1,1,
1,1,1,1,1,1,1,1,1,1,1,1,1,1,1,1,1,1,1,1,1,1,1,1,1,1,1,1,1,1,1,1,1,1,1,1,
1,1,1,1,1,1,1,1,1,1,1,1,1,1,1,1,1,1,1,6),(2,2),(-1.,-0.985714285714284,
-0.97142857142857,-0.957142857142856,-0.942857142857141,-0.928571428571427,
-0.914285714285713,-0.899999999999999,-0.885714285714284,-0.87142857142857,
-0.857142857142856,-0.842857142857142,-0.828571428571428,-0.814285714285713,
-0.799999999999999,-0.785714285714285,-0.771428571428571,-0.757142857142856,
-0.742857142857142,-0.728571428571428,-0.714285714285714,-0.699999999999999,
-0.685714285714285,-0.671428571428571,-0.657142857142857,-0.642857142857142,
-0.628571428571428,-0.614285714285714,-0.6,-0.585714285714286,-0.571428571428571,
-0.557142857142857,-0.542857142857143,-0.528571428571429,-0.514285714285714,
-0.5,-0.485714285714286,-0.471428571428572,-0.457142857142857,-0.442857142857143,
-0.428571428571429,-0.414285714285714,-0.4,-0.385714285714286,-0.371428571428571,
-0.357142857142857,-0.342857142857143,-0.328571428571429,-0.314285714285714,
-0.3,-0.285714285714286,-0.271428571428571,-0.257142857142857,-0.242857142857143,
-0.228571428571429,-0.214285714285714,-0.2,-0.185714285714286,-0.171428571428571,
-0.157142857142857,-0.142857142857143,-0.128571428571429,-0.114285714285714,
-0.1,-0.0857142857142857,-0.0714285714285714,-0.0571428571428571,-0.0428571428571429,
-0.0285714285714286,-0.0142857142857143,0.),(0.,2.1),.UNSPECIFIED.);
#200=B_SPLINE_SURFACE_WITH_KNOTS('',5,1,((#10077,#10078),(#10079,#10080),
(#10081,#10082),(#10083,#10084),(#10085,#10086),(#10087,#10088),(#10089,
#10090),(#10091,#10092),(#10093,#10094),(#10095,#10096),(#10097,#10098),
(#10099,#10100),(#10101,#10102),(#10103,#10104),(#10105,#10106),(#10107,
#10108),(#10109,#10110),(#10111,#10112),(#10113,#10114),(#10115,#10116),
(#10117,#10118),(#10119,#10120),(#10121,#10122),(#10123,#10124),(#10125,
#10126),(#10127,#10128),(#10129,#10130),(#10131,#10132),(#10133,#10134),
(#10135,#10136),(#10137,#10138),(#10139,#10140),(#10141,#10142),(#10143,
#10144),(#10145,#10146),(#10147,#10148),(#10149,#10150),(#10151,#10152),
(#10153,#10154),(#10155,#10156),(#10157,#10158),(#10159,#10160),(#10161,
#10162),(#10163,#10164),(#10165,#10166),(#10167,#10168),(#10169,#10170),
(#10171,#10172),(#10173,#10174),(#10175,#10176),(#10177,#10178),(#10179,
#10180),(#10181,#10182),(#10183,#10184),(#10185,#10186),(#10187,#10188),
(#10189,#10190),(#10191,#10192),(#10193,#10194),(#10195,#10196),(#10197,
#10198),(#10199,#10200),(#10201,#10202),(#10203,#10204),(#10205,#10206),
(#10207,#10208),(#10209,#10210),(#10211,#10212),(#10213,#10214),(#10215,
#10216),(#10217,#10218),(#10219,#10220),(#10221,#10222),(#10223,#10224),
(#10225,#10226)),.UNSPECIFIED.,.F.,.F.,.F.,(6,1,1,1,1,1,1,1,1,1,1,1,1,1,
1,1,1,1,1,1,1,1,1,1,1,1,1,1,1,1,1,1,1,1,1,1,1,1,1,1,1,1,1,1,1,1,1,1,1,1,
1,1,1,1,1,1,1,1,1,1,1,1,1,1,1,1,1,1,1,1,6),(2,2),(0.,0.0142857142857143,
0.0285714285714286,0.0428571428571429,0.0571428571428571,0.0714285714285714,
0.0857142857142857,0.1,0.114285714285714,0.128571428571429,0.142857142857143,
0.157142857142857,0.171428571428571,0.185714285714286,0.2,0.214285714285714,
0.228571428571429,0.242857142857143,0.257142857142857,0.271428571428571,
0.285714285714286,0.3,0.314285714285714,0.328571428571429,0.342857142857143,
0.357142857142857,0.371428571428571,0.385714285714286,0.4,0.414285714285714,
0.428571428571429,0.442857142857143,0.457142857142857,0.471428571428572,
0.485714285714286,0.5,0.514285714285714,0.528571428571429,0.542857142857143,
0.557142857142857,0.571428571428571,0.585714285714286,0.6,0.614285714285714,
0.628571428571428,0.642857142857142,0.657142857142857,0.671428571428571,
0.685714285714285,0.699999999999999,0.714285714285714,0.728571428571428,
0.742857142857142,0.757142857142856,0.771428571428571,0.785714285714285,
0.799999999999999,0.814285714285713,0.828571428571428,0.842857142857142,
0.857142857142856,0.87142857142857,0.885714285714284,0.899999999999999,
0.914285714285713,0.928571428571427,0.942857142857141,0.957142857142856,
0.97142857142857,0.985714285714284,1.),(0.,2.1),.UNSPECIFIED.);
#201=B_SPLINE_SURFACE_WITH_KNOTS('',5,1,((#10371,#10372),(#10373,#10374),
(#10375,#10376),(#10377,#10378),(#10379,#10380),(#10381,#10382),(#10383,
#10384),(#10385,#10386),(#10387,#10388),(#10389,#10390),(#10391,#10392),
(#10393,#10394),(#10395,#10396),(#10397,#10398),(#10399,#10400),(#10401,
#10402),(#10403,#10404),(#10405,#10406),(#10407,#10408),(#10409,#10410),
(#10411,#10412),(#10413,#10414),(#10415,#10416),(#10417,#10418),(#10419,
#10420),(#10421,#10422),(#10423,#10424),(#10425,#10426),(#10427,#10428),
(#10429,#10430),(#10431,#10432),(#10433,#10434),(#10435,#10436),(#10437,
#10438),(#10439,#10440),(#10441,#10442),(#10443,#10444),(#10445,#10446),
(#10447,#10448),(#10449,#10450),(#10451,#10452),(#10453,#10454),(#10455,
#10456),(#10457,#10458),(#10459,#10460),(#10461,#10462),(#10463,#10464),
(#10465,#10466),(#10467,#10468),(#10469,#10470),(#10471,#10472),(#10473,
#10474),(#10475,#10476),(#10477,#10478),(#10479,#10480),(#10481,#10482),
(#10483,#10484),(#10485,#10486),(#10487,#10488),(#10489,#10490),(#10491,
#10492),(#10493,#10494),(#10495,#10496),(#10497,#10498),(#10499,#10500),
(#10501,#10502),(#10503,#10504),(#10505,#10506),(#10507,#10508),(#10509,
#10510),(#10511,#10512),(#10513,#10514),(#10515,#10516),(#10517,#10518),
(#10519,#10520)),.UNSPECIFIED.,.F.,.F.,.F.,(6,1,1,1,1,1,1,1,1,1,1,1,1,1,
1,1,1,1,1,1,1,1,1,1,1,1,1,1,1,1,1,1,1,1,1,1,1,1,1,1,1,1,1,1,1,1,1,1,1,1,
1,1,1,1,1,1,1,1,1,1,1,1,1,1,1,1,1,1,1,1,6),(2,2),(-1.,-0.985714285714284,
-0.97142857142857,-0.957142857142856,-0.942857142857141,-0.928571428571427,
-0.914285714285713,-0.899999999999999,-0.885714285714284,-0.87142857142857,
-0.857142857142856,-0.842857142857142,-0.828571428571428,-0.814285714285713,
-0.799999999999999,-0.785714285714285,-0.771428571428571,-0.757142857142856,
-0.742857142857142,-0.728571428571428,-0.714285714285714,-0.699999999999999,
-0.685714285714285,-0.671428571428571,-0.657142857142857,-0.642857142857142,
-0.628571428571428,-0.614285714285714,-0.6,-0.585714285714286,-0.571428571428571,
-0.557142857142857,-0.542857142857143,-0.528571428571429,-0.514285714285714,
-0.5,-0.485714285714286,-0.471428571428572,-0.457142857142857,-0.442857142857143,
-0.428571428571429,-0.414285714285714,-0.4,-0.385714285714286,-0.371428571428571,
-0.357142857142857,-0.342857142857143,-0.328571428571429,-0.314285714285714,
-0.3,-0.285714285714286,-0.271428571428571,-0.257142857142857,-0.242857142857143,
-0.228571428571429,-0.214285714285714,-0.2,-0.185714285714286,-0.171428571428571,
-0.157142857142857,-0.142857142857143,-0.128571428571429,-0.114285714285714,
-0.1,-0.0857142857142857,-0.0714285714285714,-0.0571428571428571,-0.0428571428571429,
-0.0285714285714286,-0.0142857142857143,0.),(0.,2.1),.UNSPECIFIED.);
#202=B_SPLINE_SURFACE_WITH_KNOTS('',5,1,((#10671,#10672),(#10673,#10674),
(#10675,#10676),(#10677,#10678),(#10679,#10680),(#10681,#10682),(#10683,
#10684),(#10685,#10686),(#10687,#10688),(#10689,#10690),(#10691,#10692),
(#10693,#10694),(#10695,#10696),(#10697,#10698),(#10699,#10700),(#10701,
#10702),(#10703,#10704),(#10705,#10706),(#10707,#10708),(#10709,#10710),
(#10711,#10712),(#10713,#10714),(#10715,#10716),(#10717,#10718),(#10719,
#10720),(#10721,#10722),(#10723,#10724),(#10725,#10726),(#10727,#10728),
(#10729,#10730),(#10731,#10732),(#10733,#10734),(#10735,#10736),(#10737,
#10738),(#10739,#10740),(#10741,#10742),(#10743,#10744),(#10745,#10746),
(#10747,#10748),(#10749,#10750),(#10751,#10752),(#10753,#10754),(#10755,
#10756),(#10757,#10758),(#10759,#10760),(#10761,#10762),(#10763,#10764),
(#10765,#10766),(#10767,#10768),(#10769,#10770),(#10771,#10772),(#10773,
#10774),(#10775,#10776),(#10777,#10778),(#10779,#10780),(#10781,#10782),
(#10783,#10784),(#10785,#10786),(#10787,#10788),(#10789,#10790),(#10791,
#10792),(#10793,#10794),(#10795,#10796),(#10797,#10798),(#10799,#10800),
(#10801,#10802),(#10803,#10804),(#10805,#10806),(#10807,#10808),(#10809,
#10810),(#10811,#10812),(#10813,#10814),(#10815,#10816),(#10817,#10818),
(#10819,#10820)),.UNSPECIFIED.,.F.,.F.,.F.,(6,1,1,1,1,1,1,1,1,1,1,1,1,1,
1,1,1,1,1,1,1,1,1,1,1,1,1,1,1,1,1,1,1,1,1,1,1,1,1,1,1,1,1,1,1,1,1,1,1,1,
1,1,1,1,1,1,1,1,1,1,1,1,1,1,1,1,1,1,1,1,6),(2,2),(0.,0.0142857142857143,
0.0285714285714286,0.0428571428571429,0.0571428571428571,0.0714285714285714,
0.0857142857142857,0.1,0.114285714285714,0.128571428571429,0.142857142857143,
0.157142857142857,0.171428571428571,0.185714285714286,0.2,0.214285714285714,
0.228571428571429,0.242857142857143,0.257142857142857,0.271428571428571,
0.285714285714286,0.3,0.314285714285714,0.328571428571429,0.342857142857143,
0.357142857142857,0.371428571428571,0.385714285714286,0.4,0.414285714285714,
0.428571428571429,0.442857142857143,0.457142857142857,0.471428571428572,
0.485714285714286,0.5,0.514285714285714,0.528571428571429,0.542857142857143,
0.557142857142857,0.571428571428571,0.585714285714286,0.6,0.614285714285714,
0.628571428571428,0.642857142857142,0.657142857142857,0.671428571428571,
0.685714285714285,0.699999999999999,0.714285714285714,0.728571428571428,
0.742857142857142,0.757142857142856,0.771428571428571,0.785714285714285,
0.799999999999999,0.814285714285713,0.828571428571428,0.842857142857142,
0.857142857142856,0.87142857142857,0.885714285714284,0.899999999999999,
0.914285714285713,0.928571428571427,0.942857142857141,0.957142857142856,
0.97142857142857,0.985714285714284,1.),(0.,2.1),.UNSPECIFIED.);
#203=B_SPLINE_SURFACE_WITH_KNOTS('',5,1,((#10965,#10966),(#10967,#10968),
(#10969,#10970),(#10971,#10972),(#10973,#10974),(#10975,#10976),(#10977,
#10978),(#10979,#10980),(#10981,#10982),(#10983,#10984),(#10985,#10986),
(#10987,#10988),(#10989,#10990),(#10991,#10992),(#10993,#10994),(#10995,
#10996),(#10997,#10998),(#10999,#11000),(#11001,#11002),(#11003,#11004),
(#11005,#11006),(#11007,#11008),(#11009,#11010),(#11011,#11012),(#11013,
#11014),(#11015,#11016),(#11017,#11018),(#11019,#11020),(#11021,#11022),
(#11023,#11024),(#11025,#11026),(#11027,#11028),(#11029,#11030),(#11031,
#11032),(#11033,#11034),(#11035,#11036),(#11037,#11038),(#11039,#11040),
(#11041,#11042),(#11043,#11044),(#11045,#11046),(#11047,#11048),(#11049,
#11050),(#11051,#11052),(#11053,#11054),(#11055,#11056),(#11057,#11058),
(#11059,#11060),(#11061,#11062),(#11063,#11064),(#11065,#11066),(#11067,
#11068),(#11069,#11070),(#11071,#11072),(#11073,#11074),(#11075,#11076),
(#11077,#11078),(#11079,#11080),(#11081,#11082),(#11083,#11084),(#11085,
#11086),(#11087,#11088),(#11089,#11090),(#11091,#11092),(#11093,#11094),
(#11095,#11096),(#11097,#11098),(#11099,#11100),(#11101,#11102),(#11103,
#11104),(#11105,#11106),(#11107,#11108),(#11109,#11110),(#11111,#11112),
(#11113,#11114)),.UNSPECIFIED.,.F.,.F.,.F.,(6,1,1,1,1,1,1,1,1,1,1,1,1,1,
1,1,1,1,1,1,1,1,1,1,1,1,1,1,1,1,1,1,1,1,1,1,1,1,1,1,1,1,1,1,1,1,1,1,1,1,
1,1,1,1,1,1,1,1,1,1,1,1,1,1,1,1,1,1,1,1,6),(2,2),(-1.,-0.985714285714284,
-0.97142857142857,-0.957142857142856,-0.942857142857141,-0.928571428571427,
-0.914285714285713,-0.899999999999999,-0.885714285714284,-0.87142857142857,
-0.857142857142856,-0.842857142857142,-0.828571428571428,-0.814285714285713,
-0.799999999999999,-0.785714285714285,-0.771428571428571,-0.757142857142856,
-0.742857142857142,-0.728571428571428,-0.714285714285714,-0.699999999999999,
-0.685714285714285,-0.671428571428571,-0.657142857142857,-0.642857142857142,
-0.628571428571428,-0.614285714285714,-0.6,-0.585714285714286,-0.571428571428571,
-0.557142857142857,-0.542857142857143,-0.528571428571429,-0.514285714285714,
-0.5,-0.485714285714286,-0.471428571428572,-0.457142857142857,-0.442857142857143,
-0.428571428571429,-0.414285714285714,-0.4,-0.385714285714286,-0.371428571428571,
-0.357142857142857,-0.342857142857143,-0.328571428571429,-0.314285714285714,
-0.3,-0.285714285714286,-0.271428571428571,-0.257142857142857,-0.242857142857143,
-0.228571428571429,-0.214285714285714,-0.2,-0.185714285714286,-0.171428571428571,
-0.157142857142857,-0.142857142857143,-0.128571428571429,-0.114285714285714,
-0.1,-0.0857142857142857,-0.0714285714285714,-0.0571428571428571,-0.0428571428571429,
-0.0285714285714286,-0.0142857142857143,0.),(0.,2.1),.UNSPECIFIED.);
#204=B_SPLINE_SURFACE_WITH_KNOTS('',5,1,((#11265,#11266),(#11267,#11268),
(#11269,#11270),(#11271,#11272),(#11273,#11274),(#11275,#11276),(#11277,
#11278),(#11279,#11280),(#11281,#11282),(#11283,#11284),(#11285,#11286),
(#11287,#11288),(#11289,#11290),(#11291,#11292),(#11293,#11294),(#11295,
#11296),(#11297,#11298),(#11299,#11300),(#11301,#11302),(#11303,#11304),
(#11305,#11306),(#11307,#11308),(#11309,#11310),(#11311,#11312),(#11313,
#11314),(#11315,#11316),(#11317,#11318),(#11319,#11320),(#11321,#11322),
(#11323,#11324),(#11325,#11326),(#11327,#11328),(#11329,#11330),(#11331,
#11332),(#11333,#11334),(#11335,#11336),(#11337,#11338),(#11339,#11340),
(#11341,#11342),(#11343,#11344),(#11345,#11346),(#11347,#11348),(#11349,
#11350),(#11351,#11352),(#11353,#11354),(#11355,#11356),(#11357,#11358),
(#11359,#11360),(#11361,#11362),(#11363,#11364),(#11365,#11366),(#11367,
#11368),(#11369,#11370),(#11371,#11372),(#11373,#11374),(#11375,#11376),
(#11377,#11378),(#11379,#11380),(#11381,#11382),(#11383,#11384),(#11385,
#11386),(#11387,#11388),(#11389,#11390),(#11391,#11392),(#11393,#11394),
(#11395,#11396),(#11397,#11398),(#11399,#11400),(#11401,#11402),(#11403,
#11404),(#11405,#11406),(#11407,#11408),(#11409,#11410),(#11411,#11412),
(#11413,#11414)),.UNSPECIFIED.,.F.,.F.,.F.,(6,1,1,1,1,1,1,1,1,1,1,1,1,1,
1,1,1,1,1,1,1,1,1,1,1,1,1,1,1,1,1,1,1,1,1,1,1,1,1,1,1,1,1,1,1,1,1,1,1,1,
1,1,1,1,1,1,1,1,1,1,1,1,1,1,1,1,1,1,1,1,6),(2,2),(0.,0.0142857142857143,
0.0285714285714286,0.0428571428571429,0.0571428571428571,0.0714285714285714,
0.0857142857142857,0.1,0.114285714285714,0.128571428571429,0.142857142857143,
0.157142857142857,0.171428571428571,0.185714285714286,0.2,0.214285714285714,
0.228571428571429,0.242857142857143,0.257142857142857,0.271428571428571,
0.285714285714286,0.3,0.314285714285714,0.328571428571429,0.342857142857143,
0.357142857142857,0.371428571428571,0.385714285714286,0.4,0.414285714285714,
0.428571428571429,0.442857142857143,0.457142857142857,0.471428571428572,
0.485714285714286,0.5,0.514285714285714,0.528571428571429,0.542857142857143,
0.557142857142857,0.571428571428571,0.585714285714286,0.6,0.614285714285714,
0.628571428571428,0.642857142857142,0.657142857142857,0.671428571428571,
0.685714285714285,0.699999999999999,0.714285714285714,0.728571428571428,
0.742857142857142,0.757142857142856,0.771428571428571,0.785714285714285,
0.799999999999999,0.814285714285713,0.828571428571428,0.842857142857142,
0.857142857142856,0.87142857142857,0.885714285714284,0.899999999999999,
0.914285714285713,0.928571428571427,0.942857142857141,0.957142857142856,
0.97142857142857,0.985714285714284,1.),(0.,2.1),.UNSPECIFIED.);
#205=B_SPLINE_SURFACE_WITH_KNOTS('',5,1,((#11559,#11560),(#11561,#11562),
(#11563,#11564),(#11565,#11566),(#11567,#11568),(#11569,#11570),(#11571,
#11572),(#11573,#11574),(#11575,#11576),(#11577,#11578),(#11579,#11580),
(#11581,#11582),(#11583,#11584),(#11585,#11586),(#11587,#11588),(#11589,
#11590),(#11591,#11592),(#11593,#11594),(#11595,#11596),(#11597,#11598),
(#11599,#11600),(#11601,#11602),(#11603,#11604),(#11605,#11606),(#11607,
#11608),(#11609,#11610),(#11611,#11612),(#11613,#11614),(#11615,#11616),
(#11617,#11618),(#11619,#11620),(#11621,#11622),(#11623,#11624),(#11625,
#11626),(#11627,#11628),(#11629,#11630),(#11631,#11632),(#11633,#11634),
(#11635,#11636),(#11637,#11638),(#11639,#11640),(#11641,#11642),(#11643,
#11644),(#11645,#11646),(#11647,#11648),(#11649,#11650),(#11651,#11652),
(#11653,#11654),(#11655,#11656),(#11657,#11658),(#11659,#11660),(#11661,
#11662),(#11663,#11664),(#11665,#11666),(#11667,#11668),(#11669,#11670),
(#11671,#11672),(#11673,#11674),(#11675,#11676),(#11677,#11678),(#11679,
#11680),(#11681,#11682),(#11683,#11684),(#11685,#11686),(#11687,#11688),
(#11689,#11690),(#11691,#11692),(#11693,#11694),(#11695,#11696),(#11697,
#11698),(#11699,#11700),(#11701,#11702),(#11703,#11704),(#11705,#11706),
(#11707,#11708)),.UNSPECIFIED.,.F.,.F.,.F.,(6,1,1,1,1,1,1,1,1,1,1,1,1,1,
1,1,1,1,1,1,1,1,1,1,1,1,1,1,1,1,1,1,1,1,1,1,1,1,1,1,1,1,1,1,1,1,1,1,1,1,
1,1,1,1,1,1,1,1,1,1,1,1,1,1,1,1,1,1,1,1,6),(2,2),(-1.,-0.985714285714284,
-0.97142857142857,-0.957142857142856,-0.942857142857141,-0.928571428571427,
-0.914285714285713,-0.899999999999999,-0.885714285714284,-0.87142857142857,
-0.857142857142856,-0.842857142857142,-0.828571428571428,-0.814285714285713,
-0.799999999999999,-0.785714285714285,-0.771428571428571,-0.757142857142856,
-0.742857142857142,-0.728571428571428,-0.714285714285714,-0.699999999999999,
-0.685714285714285,-0.671428571428571,-0.657142857142857,-0.642857142857142,
-0.628571428571428,-0.614285714285714,-0.6,-0.585714285714286,-0.571428571428571,
-0.557142857142857,-0.542857142857143,-0.528571428571429,-0.514285714285714,
-0.5,-0.485714285714286,-0.471428571428572,-0.457142857142857,-0.442857142857143,
-0.428571428571429,-0.414285714285714,-0.4,-0.385714285714286,-0.371428571428571,
-0.357142857142857,-0.342857142857143,-0.328571428571429,-0.314285714285714,
-0.3,-0.285714285714286,-0.271428571428571,-0.257142857142857,-0.242857142857143,
-0.228571428571429,-0.214285714285714,-0.2,-0.185714285714286,-0.171428571428571,
-0.157142857142857,-0.142857142857143,-0.128571428571429,-0.114285714285714,
-0.1,-0.0857142857142857,-0.0714285714285714,-0.0571428571428571,-0.0428571428571429,
-0.0285714285714286,-0.0142857142857143,0.),(0.,2.1),.UNSPECIFIED.);
#206=B_SPLINE_SURFACE_WITH_KNOTS('',5,1,((#11859,#11860),(#11861,#11862),
(#11863,#11864),(#11865,#11866),(#11867,#11868),(#11869,#11870),(#11871,
#11872),(#11873,#11874),(#11875,#11876),(#11877,#11878),(#11879,#11880),
(#11881,#11882),(#11883,#11884),(#11885,#11886),(#11887,#11888),(#11889,
#11890),(#11891,#11892),(#11893,#11894),(#11895,#11896),(#11897,#11898),
(#11899,#11900),(#11901,#11902),(#11903,#11904),(#11905,#11906),(#11907,
#11908),(#11909,#11910),(#11911,#11912),(#11913,#11914),(#11915,#11916),
(#11917,#11918),(#11919,#11920),(#11921,#11922),(#11923,#11924),(#11925,
#11926),(#11927,#11928),(#11929,#11930),(#11931,#11932),(#11933,#11934),
(#11935,#11936),(#11937,#11938),(#11939,#11940),(#11941,#11942),(#11943,
#11944),(#11945,#11946),(#11947,#11948),(#11949,#11950),(#11951,#11952),
(#11953,#11954),(#11955,#11956),(#11957,#11958),(#11959,#11960),(#11961,
#11962),(#11963,#11964),(#11965,#11966),(#11967,#11968),(#11969,#11970),
(#11971,#11972),(#11973,#11974),(#11975,#11976),(#11977,#11978),(#11979,
#11980),(#11981,#11982),(#11983,#11984),(#11985,#11986),(#11987,#11988),
(#11989,#11990),(#11991,#11992),(#11993,#11994),(#11995,#11996),(#11997,
#11998),(#11999,#12000),(#12001,#12002),(#12003,#12004),(#12005,#12006),
(#12007,#12008)),.UNSPECIFIED.,.F.,.F.,.F.,(6,1,1,1,1,1,1,1,1,1,1,1,1,1,
1,1,1,1,1,1,1,1,1,1,1,1,1,1,1,1,1,1,1,1,1,1,1,1,1,1,1,1,1,1,1,1,1,1,1,1,
1,1,1,1,1,1,1,1,1,1,1,1,1,1,1,1,1,1,1,1,6),(2,2),(0.,0.0142857142857143,
0.0285714285714286,0.0428571428571429,0.0571428571428571,0.0714285714285714,
0.0857142857142857,0.1,0.114285714285714,0.128571428571429,0.142857142857143,
0.157142857142857,0.171428571428571,0.185714285714286,0.2,0.214285714285714,
0.228571428571429,0.242857142857143,0.257142857142857,0.271428571428571,
0.285714285714286,0.3,0.314285714285714,0.328571428571429,0.342857142857143,
0.357142857142857,0.371428571428571,0.385714285714286,0.4,0.414285714285714,
0.428571428571429,0.442857142857143,0.457142857142857,0.471428571428572,
0.485714285714286,0.5,0.514285714285714,0.528571428571429,0.542857142857143,
0.557142857142857,0.571428571428571,0.585714285714286,0.6,0.614285714285714,
0.628571428571428,0.642857142857142,0.657142857142857,0.671428571428571,
0.685714285714285,0.699999999999999,0.714285714285714,0.728571428571428,
0.742857142857142,0.757142857142856,0.771428571428571,0.785714285714285,
0.799999999999999,0.814285714285713,0.828571428571428,0.842857142857142,
0.857142857142856,0.87142857142857,0.885714285714284,0.899999999999999,
0.914285714285713,0.928571428571427,0.942857142857141,0.957142857142856,
0.97142857142857,0.985714285714284,1.),(0.,2.1),.UNSPECIFIED.);
#207=B_SPLINE_SURFACE_WITH_KNOTS('',5,1,((#12153,#12154),(#12155,#12156),
(#12157,#12158),(#12159,#12160),(#12161,#12162),(#12163,#12164),(#12165,
#12166),(#12167,#12168),(#12169,#12170),(#12171,#12172),(#12173,#12174),
(#12175,#12176),(#12177,#12178),(#12179,#12180),(#12181,#12182),(#12183,
#12184),(#12185,#12186),(#12187,#12188),(#12189,#12190),(#12191,#12192),
(#12193,#12194),(#12195,#12196),(#12197,#12198),(#12199,#12200),(#12201,
#12202),(#12203,#12204),(#12205,#12206),(#12207,#12208),(#12209,#12210),
(#12211,#12212),(#12213,#12214),(#12215,#12216),(#12217,#12218),(#12219,
#12220),(#12221,#12222),(#12223,#12224),(#12225,#12226),(#12227,#12228),
(#12229,#12230),(#12231,#12232),(#12233,#12234),(#12235,#12236),(#12237,
#12238),(#12239,#12240),(#12241,#12242),(#12243,#12244),(#12245,#12246),
(#12247,#12248),(#12249,#12250),(#12251,#12252),(#12253,#12254),(#12255,
#12256),(#12257,#12258),(#12259,#12260),(#12261,#12262),(#12263,#12264),
(#12265,#12266),(#12267,#12268),(#12269,#12270),(#12271,#12272),(#12273,
#12274),(#12275,#12276),(#12277,#12278),(#12279,#12280),(#12281,#12282),
(#12283,#12284),(#12285,#12286),(#12287,#12288),(#12289,#12290),(#12291,
#12292),(#12293,#12294),(#12295,#12296),(#12297,#12298),(#12299,#12300),
(#12301,#12302)),.UNSPECIFIED.,.F.,.F.,.F.,(6,1,1,1,1,1,1,1,1,1,1,1,1,1,
1,1,1,1,1,1,1,1,1,1,1,1,1,1,1,1,1,1,1,1,1,1,1,1,1,1,1,1,1,1,1,1,1,1,1,1,
1,1,1,1,1,1,1,1,1,1,1,1,1,1,1,1,1,1,1,1,6),(2,2),(-1.,-0.985714285714284,
-0.97142857142857,-0.957142857142856,-0.942857142857141,-0.928571428571427,
-0.914285714285713,-0.899999999999999,-0.885714285714284,-0.87142857142857,
-0.857142857142856,-0.842857142857142,-0.828571428571428,-0.814285714285713,
-0.799999999999999,-0.785714285714285,-0.771428571428571,-0.757142857142856,
-0.742857142857142,-0.728571428571428,-0.714285714285714,-0.699999999999999,
-0.685714285714285,-0.671428571428571,-0.657142857142857,-0.642857142857142,
-0.628571428571428,-0.614285714285714,-0.6,-0.585714285714286,-0.571428571428571,
-0.557142857142857,-0.542857142857143,-0.528571428571429,-0.514285714285714,
-0.5,-0.485714285714286,-0.471428571428572,-0.457142857142857,-0.442857142857143,
-0.428571428571429,-0.414285714285714,-0.4,-0.385714285714286,-0.371428571428571,
-0.357142857142857,-0.342857142857143,-0.328571428571429,-0.314285714285714,
-0.3,-0.285714285714286,-0.271428571428571,-0.257142857142857,-0.242857142857143,
-0.228571428571429,-0.214285714285714,-0.2,-0.185714285714286,-0.171428571428571,
-0.157142857142857,-0.142857142857143,-0.128571428571429,-0.114285714285714,
-0.1,-0.0857142857142857,-0.0714285714285714,-0.0571428571428571,-0.0428571428571429,
-0.0285714285714286,-0.0142857142857143,0.),(0.,2.1),.UNSPECIFIED.);
#208=B_SPLINE_SURFACE_WITH_KNOTS('',5,1,((#12453,#12454),(#12455,#12456),
(#12457,#12458),(#12459,#12460),(#12461,#12462),(#12463,#12464),(#12465,
#12466),(#12467,#12468),(#12469,#12470),(#12471,#12472),(#12473,#12474),
(#12475,#12476),(#12477,#12478),(#12479,#12480),(#12481,#12482),(#12483,
#12484),(#12485,#12486),(#12487,#12488),(#12489,#12490),(#12491,#12492),
(#12493,#12494),(#12495,#12496),(#12497,#12498),(#12499,#12500),(#12501,
#12502),(#12503,#12504),(#12505,#12506),(#12507,#12508),(#12509,#12510),
(#12511,#12512),(#12513,#12514),(#12515,#12516),(#12517,#12518),(#12519,
#12520),(#12521,#12522),(#12523,#12524),(#12525,#12526),(#12527,#12528),
(#12529,#12530),(#12531,#12532),(#12533,#12534),(#12535,#12536),(#12537,
#12538),(#12539,#12540),(#12541,#12542),(#12543,#12544),(#12545,#12546),
(#12547,#12548),(#12549,#12550),(#12551,#12552),(#12553,#12554),(#12555,
#12556),(#12557,#12558),(#12559,#12560),(#12561,#12562),(#12563,#12564),
(#12565,#12566),(#12567,#12568),(#12569,#12570),(#12571,#12572),(#12573,
#12574),(#12575,#12576),(#12577,#12578),(#12579,#12580),(#12581,#12582),
(#12583,#12584),(#12585,#12586),(#12587,#12588),(#12589,#12590),(#12591,
#12592),(#12593,#12594),(#12595,#12596),(#12597,#12598),(#12599,#12600),
(#12601,#12602)),.UNSPECIFIED.,.F.,.F.,.F.,(6,1,1,1,1,1,1,1,1,1,1,1,1,1,
1,1,1,1,1,1,1,1,1,1,1,1,1,1,1,1,1,1,1,1,1,1,1,1,1,1,1,1,1,1,1,1,1,1,1,1,
1,1,1,1,1,1,1,1,1,1,1,1,1,1,1,1,1,1,1,1,6),(2,2),(0.,0.0142857142857143,
0.0285714285714286,0.0428571428571429,0.0571428571428571,0.0714285714285714,
0.0857142857142857,0.1,0.114285714285714,0.128571428571429,0.142857142857143,
0.157142857142857,0.171428571428571,0.185714285714286,0.2,0.214285714285714,
0.228571428571429,0.242857142857143,0.257142857142857,0.271428571428571,
0.285714285714286,0.3,0.314285714285714,0.328571428571429,0.342857142857143,
0.357142857142857,0.371428571428571,0.385714285714286,0.4,0.414285714285714,
0.428571428571429,0.442857142857143,0.457142857142857,0.471428571428572,
0.485714285714286,0.5,0.514285714285714,0.528571428571429,0.542857142857143,
0.557142857142857,0.571428571428571,0.585714285714286,0.6,0.614285714285714,
0.628571428571428,0.642857142857142,0.657142857142857,0.671428571428571,
0.685714285714285,0.699999999999999,0.714285714285714,0.728571428571428,
0.742857142857142,0.757142857142856,0.771428571428571,0.785714285714285,
0.799999999999999,0.814285714285713,0.828571428571428,0.842857142857142,
0.857142857142856,0.87142857142857,0.885714285714284,0.899999999999999,
0.914285714285713,0.928571428571427,0.942857142857141,0.957142857142856,
0.97142857142857,0.985714285714284,1.),(0.,2.1),.UNSPECIFIED.);
#209=B_SPLINE_SURFACE_WITH_KNOTS('',5,1,((#12747,#12748),(#12749,#12750),
(#12751,#12752),(#12753,#12754),(#12755,#12756),(#12757,#12758),(#12759,
#12760),(#12761,#12762),(#12763,#12764),(#12765,#12766),(#12767,#12768),
(#12769,#12770),(#12771,#12772),(#12773,#12774),(#12775,#12776),(#12777,
#12778),(#12779,#12780),(#12781,#12782),(#12783,#12784),(#12785,#12786),
(#12787,#12788),(#12789,#12790),(#12791,#12792),(#12793,#12794),(#12795,
#12796),(#12797,#12798),(#12799,#12800),(#12801,#12802),(#12803,#12804),
(#12805,#12806),(#12807,#12808),(#12809,#12810),(#12811,#12812),(#12813,
#12814),(#12815,#12816),(#12817,#12818),(#12819,#12820),(#12821,#12822),
(#12823,#12824),(#12825,#12826),(#12827,#12828),(#12829,#12830),(#12831,
#12832),(#12833,#12834),(#12835,#12836),(#12837,#12838),(#12839,#12840),
(#12841,#12842),(#12843,#12844),(#12845,#12846),(#12847,#12848),(#12849,
#12850),(#12851,#12852),(#12853,#12854),(#12855,#12856),(#12857,#12858),
(#12859,#12860),(#12861,#12862),(#12863,#12864),(#12865,#12866),(#12867,
#12868),(#12869,#12870),(#12871,#12872),(#12873,#12874),(#12875,#12876),
(#12877,#12878),(#12879,#12880),(#12881,#12882),(#12883,#12884),(#12885,
#12886),(#12887,#12888),(#12889,#12890),(#12891,#12892),(#12893,#12894),
(#12895,#12896)),.UNSPECIFIED.,.F.,.F.,.F.,(6,1,1,1,1,1,1,1,1,1,1,1,1,1,
1,1,1,1,1,1,1,1,1,1,1,1,1,1,1,1,1,1,1,1,1,1,1,1,1,1,1,1,1,1,1,1,1,1,1,1,
1,1,1,1,1,1,1,1,1,1,1,1,1,1,1,1,1,1,1,1,6),(2,2),(-1.,-0.985714285714284,
-0.97142857142857,-0.957142857142856,-0.942857142857141,-0.928571428571427,
-0.914285714285713,-0.899999999999999,-0.885714285714284,-0.87142857142857,
-0.857142857142856,-0.842857142857142,-0.828571428571428,-0.814285714285713,
-0.799999999999999,-0.785714285714285,-0.771428571428571,-0.757142857142856,
-0.742857142857142,-0.728571428571428,-0.714285714285714,-0.699999999999999,
-0.685714285714285,-0.671428571428571,-0.657142857142857,-0.642857142857142,
-0.628571428571428,-0.614285714285714,-0.6,-0.585714285714286,-0.571428571428571,
-0.557142857142857,-0.542857142857143,-0.528571428571429,-0.514285714285714,
-0.5,-0.485714285714286,-0.471428571428572,-0.457142857142857,-0.442857142857143,
-0.428571428571429,-0.414285714285714,-0.4,-0.385714285714286,-0.371428571428571,
-0.357142857142857,-0.342857142857143,-0.328571428571429,-0.314285714285714,
-0.3,-0.285714285714286,-0.271428571428571,-0.257142857142857,-0.242857142857143,
-0.228571428571429,-0.214285714285714,-0.2,-0.185714285714286,-0.171428571428571,
-0.157142857142857,-0.142857142857143,-0.128571428571429,-0.114285714285714,
-0.1,-0.0857142857142857,-0.0714285714285714,-0.0571428571428571,-0.0428571428571429,
-0.0285714285714286,-0.0142857142857143,0.),(0.,2.1),.UNSPECIFIED.);
#210=B_SPLINE_SURFACE_WITH_KNOTS('',5,1,((#13047,#13048),(#13049,#13050),
(#13051,#13052),(#13053,#13054),(#13055,#13056),(#13057,#13058),(#13059,
#13060),(#13061,#13062),(#13063,#13064),(#13065,#13066),(#13067,#13068),
(#13069,#13070),(#13071,#13072),(#13073,#13074),(#13075,#13076),(#13077,
#13078),(#13079,#13080),(#13081,#13082),(#13083,#13084),(#13085,#13086),
(#13087,#13088),(#13089,#13090),(#13091,#13092),(#13093,#13094),(#13095,
#13096),(#13097,#13098),(#13099,#13100),(#13101,#13102),(#13103,#13104),
(#13105,#13106),(#13107,#13108),(#13109,#13110),(#13111,#13112),(#13113,
#13114),(#13115,#13116),(#13117,#13118),(#13119,#13120),(#13121,#13122),
(#13123,#13124),(#13125,#13126),(#13127,#13128),(#13129,#13130),(#13131,
#13132),(#13133,#13134),(#13135,#13136),(#13137,#13138),(#13139,#13140),
(#13141,#13142),(#13143,#13144),(#13145,#13146),(#13147,#13148),(#13149,
#13150),(#13151,#13152),(#13153,#13154),(#13155,#13156),(#13157,#13158),
(#13159,#13160),(#13161,#13162),(#13163,#13164),(#13165,#13166),(#13167,
#13168),(#13169,#13170),(#13171,#13172),(#13173,#13174),(#13175,#13176),
(#13177,#13178),(#13179,#13180),(#13181,#13182),(#13183,#13184),(#13185,
#13186),(#13187,#13188),(#13189,#13190),(#13191,#13192),(#13193,#13194),
(#13195,#13196)),.UNSPECIFIED.,.F.,.F.,.F.,(6,1,1,1,1,1,1,1,1,1,1,1,1,1,
1,1,1,1,1,1,1,1,1,1,1,1,1,1,1,1,1,1,1,1,1,1,1,1,1,1,1,1,1,1,1,1,1,1,1,1,
1,1,1,1,1,1,1,1,1,1,1,1,1,1,1,1,1,1,1,1,6),(2,2),(0.,0.0142857142857143,
0.0285714285714286,0.0428571428571429,0.0571428571428571,0.0714285714285714,
0.0857142857142857,0.1,0.114285714285714,0.128571428571429,0.142857142857143,
0.157142857142857,0.171428571428571,0.185714285714286,0.2,0.214285714285714,
0.228571428571429,0.242857142857143,0.257142857142857,0.271428571428571,
0.285714285714286,0.3,0.314285714285714,0.328571428571429,0.342857142857143,
0.357142857142857,0.371428571428571,0.385714285714286,0.4,0.414285714285714,
0.428571428571429,0.442857142857143,0.457142857142857,0.471428571428572,
0.485714285714286,0.5,0.514285714285714,0.528571428571429,0.542857142857143,
0.557142857142857,0.571428571428571,0.585714285714286,0.6,0.614285714285714,
0.628571428571428,0.642857142857142,0.657142857142857,0.671428571428571,
0.685714285714285,0.699999999999999,0.714285714285714,0.728571428571428,
0.742857142857142,0.757142857142856,0.771428571428571,0.785714285714285,
0.799999999999999,0.814285714285713,0.828571428571428,0.842857142857142,
0.857142857142856,0.87142857142857,0.885714285714284,0.899999999999999,
0.914285714285713,0.928571428571427,0.942857142857141,0.957142857142856,
0.97142857142857,0.985714285714284,1.),(0.,2.1),.UNSPECIFIED.);
#211=B_SPLINE_SURFACE_WITH_KNOTS('',5,1,((#13341,#13342),(#13343,#13344),
(#13345,#13346),(#13347,#13348),(#13349,#13350),(#13351,#13352),(#13353,
#13354),(#13355,#13356),(#13357,#13358),(#13359,#13360),(#13361,#13362),
(#13363,#13364),(#13365,#13366),(#13367,#13368),(#13369,#13370),(#13371,
#13372),(#13373,#13374),(#13375,#13376),(#13377,#13378),(#13379,#13380),
(#13381,#13382),(#13383,#13384),(#13385,#13386),(#13387,#13388),(#13389,
#13390),(#13391,#13392),(#13393,#13394),(#13395,#13396),(#13397,#13398),
(#13399,#13400),(#13401,#13402),(#13403,#13404),(#13405,#13406),(#13407,
#13408),(#13409,#13410),(#13411,#13412),(#13413,#13414),(#13415,#13416),
(#13417,#13418),(#13419,#13420),(#13421,#13422),(#13423,#13424),(#13425,
#13426),(#13427,#13428),(#13429,#13430),(#13431,#13432),(#13433,#13434),
(#13435,#13436),(#13437,#13438),(#13439,#13440),(#13441,#13442),(#13443,
#13444),(#13445,#13446),(#13447,#13448),(#13449,#13450),(#13451,#13452),
(#13453,#13454),(#13455,#13456),(#13457,#13458),(#13459,#13460),(#13461,
#13462),(#13463,#13464),(#13465,#13466),(#13467,#13468),(#13469,#13470),
(#13471,#13472),(#13473,#13474),(#13475,#13476),(#13477,#13478),(#13479,
#13480),(#13481,#13482),(#13483,#13484),(#13485,#13486),(#13487,#13488),
(#13489,#13490)),.UNSPECIFIED.,.F.,.F.,.F.,(6,1,1,1,1,1,1,1,1,1,1,1,1,1,
1,1,1,1,1,1,1,1,1,1,1,1,1,1,1,1,1,1,1,1,1,1,1,1,1,1,1,1,1,1,1,1,1,1,1,1,
1,1,1,1,1,1,1,1,1,1,1,1,1,1,1,1,1,1,1,1,6),(2,2),(-1.,-0.985714285714284,
-0.97142857142857,-0.957142857142856,-0.942857142857141,-0.928571428571427,
-0.914285714285713,-0.899999999999999,-0.885714285714284,-0.87142857142857,
-0.857142857142856,-0.842857142857142,-0.828571428571428,-0.814285714285713,
-0.799999999999999,-0.785714285714285,-0.771428571428571,-0.757142857142856,
-0.742857142857142,-0.728571428571428,-0.714285714285714,-0.699999999999999,
-0.685714285714285,-0.671428571428571,-0.657142857142857,-0.642857142857142,
-0.628571428571428,-0.614285714285714,-0.6,-0.585714285714286,-0.571428571428571,
-0.557142857142857,-0.542857142857143,-0.528571428571429,-0.514285714285714,
-0.5,-0.485714285714286,-0.471428571428572,-0.457142857142857,-0.442857142857143,
-0.428571428571429,-0.414285714285714,-0.4,-0.385714285714286,-0.371428571428571,
-0.357142857142857,-0.342857142857143,-0.328571428571429,-0.314285714285714,
-0.3,-0.285714285714286,-0.271428571428571,-0.257142857142857,-0.242857142857143,
-0.228571428571429,-0.214285714285714,-0.2,-0.185714285714286,-0.171428571428571,
-0.157142857142857,-0.142857142857143,-0.128571428571429,-0.114285714285714,
-0.1,-0.0857142857142857,-0.0714285714285714,-0.0571428571428571,-0.0428571428571429,
-0.0285714285714286,-0.0142857142857143,0.),(0.,2.1),.UNSPECIFIED.);
#212=B_SPLINE_SURFACE_WITH_KNOTS('',5,1,((#13641,#13642),(#13643,#13644),
(#13645,#13646),(#13647,#13648),(#13649,#13650),(#13651,#13652),(#13653,
#13654),(#13655,#13656),(#13657,#13658),(#13659,#13660),(#13661,#13662),
(#13663,#13664),(#13665,#13666),(#13667,#13668),(#13669,#13670),(#13671,
#13672),(#13673,#13674),(#13675,#13676),(#13677,#13678),(#13679,#13680),
(#13681,#13682),(#13683,#13684),(#13685,#13686),(#13687,#13688),(#13689,
#13690),(#13691,#13692),(#13693,#13694),(#13695,#13696),(#13697,#13698),
(#13699,#13700),(#13701,#13702),(#13703,#13704),(#13705,#13706),(#13707,
#13708),(#13709,#13710),(#13711,#13712),(#13713,#13714),(#13715,#13716),
(#13717,#13718),(#13719,#13720),(#13721,#13722),(#13723,#13724),(#13725,
#13726),(#13727,#13728),(#13729,#13730),(#13731,#13732),(#13733,#13734),
(#13735,#13736),(#13737,#13738),(#13739,#13740),(#13741,#13742),(#13743,
#13744),(#13745,#13746),(#13747,#13748),(#13749,#13750),(#13751,#13752),
(#13753,#13754),(#13755,#13756),(#13757,#13758),(#13759,#13760),(#13761,
#13762),(#13763,#13764),(#13765,#13766),(#13767,#13768),(#13769,#13770),
(#13771,#13772),(#13773,#13774),(#13775,#13776),(#13777,#13778),(#13779,
#13780),(#13781,#13782),(#13783,#13784),(#13785,#13786),(#13787,#13788),
(#13789,#13790)),.UNSPECIFIED.,.F.,.F.,.F.,(6,1,1,1,1,1,1,1,1,1,1,1,1,1,
1,1,1,1,1,1,1,1,1,1,1,1,1,1,1,1,1,1,1,1,1,1,1,1,1,1,1,1,1,1,1,1,1,1,1,1,
1,1,1,1,1,1,1,1,1,1,1,1,1,1,1,1,1,1,1,1,6),(2,2),(0.,0.0142857142857143,
0.0285714285714286,0.0428571428571429,0.0571428571428571,0.0714285714285714,
0.0857142857142857,0.1,0.114285714285714,0.128571428571429,0.142857142857143,
0.157142857142857,0.171428571428571,0.185714285714286,0.2,0.214285714285714,
0.228571428571429,0.242857142857143,0.257142857142857,0.271428571428571,
0.285714285714286,0.3,0.314285714285714,0.328571428571429,0.342857142857143,
0.357142857142857,0.371428571428571,0.385714285714286,0.4,0.414285714285714,
0.428571428571429,0.442857142857143,0.457142857142857,0.471428571428572,
0.485714285714286,0.5,0.514285714285714,0.528571428571429,0.542857142857143,
0.557142857142857,0.571428571428571,0.585714285714286,0.6,0.614285714285714,
0.628571428571428,0.642857142857142,0.657142857142857,0.671428571428571,
0.685714285714285,0.699999999999999,0.714285714285714,0.728571428571428,
0.742857142857142,0.757142857142856,0.771428571428571,0.785714285714285,
0.799999999999999,0.814285714285713,0.828571428571428,0.842857142857142,
0.857142857142856,0.87142857142857,0.885714285714284,0.899999999999999,
0.914285714285713,0.928571428571427,0.942857142857141,0.957142857142856,
0.97142857142857,0.985714285714284,1.),(0.,2.1),.UNSPECIFIED.);
#213=B_SPLINE_SURFACE_WITH_KNOTS('',5,1,((#13935,#13936),(#13937,#13938),
(#13939,#13940),(#13941,#13942),(#13943,#13944),(#13945,#13946),(#13947,
#13948),(#13949,#13950),(#13951,#13952),(#13953,#13954),(#13955,#13956),
(#13957,#13958),(#13959,#13960),(#13961,#13962),(#13963,#13964),(#13965,
#13966),(#13967,#13968),(#13969,#13970),(#13971,#13972),(#13973,#13974),
(#13975,#13976),(#13977,#13978),(#13979,#13980),(#13981,#13982),(#13983,
#13984),(#13985,#13986),(#13987,#13988),(#13989,#13990),(#13991,#13992),
(#13993,#13994),(#13995,#13996),(#13997,#13998),(#13999,#14000),(#14001,
#14002),(#14003,#14004),(#14005,#14006),(#14007,#14008),(#14009,#14010),
(#14011,#14012),(#14013,#14014),(#14015,#14016),(#14017,#14018),(#14019,
#14020),(#14021,#14022),(#14023,#14024),(#14025,#14026),(#14027,#14028),
(#14029,#14030),(#14031,#14032),(#14033,#14034),(#14035,#14036),(#14037,
#14038),(#14039,#14040),(#14041,#14042),(#14043,#14044),(#14045,#14046),
(#14047,#14048),(#14049,#14050),(#14051,#14052),(#14053,#14054),(#14055,
#14056),(#14057,#14058),(#14059,#14060),(#14061,#14062),(#14063,#14064),
(#14065,#14066),(#14067,#14068),(#14069,#14070),(#14071,#14072),(#14073,
#14074),(#14075,#14076),(#14077,#14078),(#14079,#14080),(#14081,#14082),
(#14083,#14084)),.UNSPECIFIED.,.F.,.F.,.F.,(6,1,1,1,1,1,1,1,1,1,1,1,1,1,
1,1,1,1,1,1,1,1,1,1,1,1,1,1,1,1,1,1,1,1,1,1,1,1,1,1,1,1,1,1,1,1,1,1,1,1,
1,1,1,1,1,1,1,1,1,1,1,1,1,1,1,1,1,1,1,1,6),(2,2),(-1.,-0.985714285714284,
-0.97142857142857,-0.957142857142856,-0.942857142857141,-0.928571428571427,
-0.914285714285713,-0.899999999999999,-0.885714285714284,-0.87142857142857,
-0.857142857142856,-0.842857142857142,-0.828571428571428,-0.814285714285713,
-0.799999999999999,-0.785714285714285,-0.771428571428571,-0.757142857142856,
-0.742857142857142,-0.728571428571428,-0.714285714285714,-0.699999999999999,
-0.685714285714285,-0.671428571428571,-0.657142857142857,-0.642857142857142,
-0.628571428571428,-0.614285714285714,-0.6,-0.585714285714286,-0.571428571428571,
-0.557142857142857,-0.542857142857143,-0.528571428571429,-0.514285714285714,
-0.5,-0.485714285714286,-0.471428571428572,-0.457142857142857,-0.442857142857143,
-0.428571428571429,-0.414285714285714,-0.4,-0.385714285714286,-0.371428571428571,
-0.357142857142857,-0.342857142857143,-0.328571428571429,-0.314285714285714,
-0.3,-0.285714285714286,-0.271428571428571,-0.257142857142857,-0.242857142857143,
-0.228571428571429,-0.214285714285714,-0.2,-0.185714285714286,-0.171428571428571,
-0.157142857142857,-0.142857142857143,-0.128571428571429,-0.114285714285714,
-0.1,-0.0857142857142857,-0.0714285714285714,-0.0571428571428571,-0.0428571428571429,
-0.0285714285714286,-0.0142857142857143,0.),(0.,2.1),.UNSPECIFIED.);
#214=B_SPLINE_SURFACE_WITH_KNOTS('',5,1,((#14235,#14236),(#14237,#14238),
(#14239,#14240),(#14241,#14242),(#14243,#14244),(#14245,#14246),(#14247,
#14248),(#14249,#14250),(#14251,#14252),(#14253,#14254),(#14255,#14256),
(#14257,#14258),(#14259,#14260),(#14261,#14262),(#14263,#14264),(#14265,
#14266),(#14267,#14268),(#14269,#14270),(#14271,#14272),(#14273,#14274),
(#14275,#14276),(#14277,#14278),(#14279,#14280),(#14281,#14282),(#14283,
#14284),(#14285,#14286),(#14287,#14288),(#14289,#14290),(#14291,#14292),
(#14293,#14294),(#14295,#14296),(#14297,#14298),(#14299,#14300),(#14301,
#14302),(#14303,#14304),(#14305,#14306),(#14307,#14308),(#14309,#14310),
(#14311,#14312),(#14313,#14314),(#14315,#14316),(#14317,#14318),(#14319,
#14320),(#14321,#14322),(#14323,#14324),(#14325,#14326),(#14327,#14328),
(#14329,#14330),(#14331,#14332),(#14333,#14334),(#14335,#14336),(#14337,
#14338),(#14339,#14340),(#14341,#14342),(#14343,#14344),(#14345,#14346),
(#14347,#14348),(#14349,#14350),(#14351,#14352),(#14353,#14354),(#14355,
#14356),(#14357,#14358),(#14359,#14360),(#14361,#14362),(#14363,#14364),
(#14365,#14366),(#14367,#14368),(#14369,#14370),(#14371,#14372),(#14373,
#14374),(#14375,#14376),(#14377,#14378),(#14379,#14380),(#14381,#14382),
(#14383,#14384)),.UNSPECIFIED.,.F.,.F.,.F.,(6,1,1,1,1,1,1,1,1,1,1,1,1,1,
1,1,1,1,1,1,1,1,1,1,1,1,1,1,1,1,1,1,1,1,1,1,1,1,1,1,1,1,1,1,1,1,1,1,1,1,
1,1,1,1,1,1,1,1,1,1,1,1,1,1,1,1,1,1,1,1,6),(2,2),(0.,0.0142857142857143,
0.0285714285714286,0.0428571428571429,0.0571428571428571,0.0714285714285714,
0.0857142857142857,0.1,0.114285714285714,0.128571428571429,0.142857142857143,
0.157142857142857,0.171428571428571,0.185714285714286,0.2,0.214285714285714,
0.228571428571429,0.242857142857143,0.257142857142857,0.271428571428571,
0.285714285714286,0.3,0.314285714285714,0.328571428571429,0.342857142857143,
0.357142857142857,0.371428571428571,0.385714285714286,0.4,0.414285714285714,
0.428571428571429,0.442857142857143,0.457142857142857,0.471428571428572,
0.485714285714286,0.5,0.514285714285714,0.528571428571429,0.542857142857143,
0.557142857142857,0.571428571428571,0.585714285714286,0.6,0.614285714285714,
0.628571428571428,0.642857142857142,0.657142857142857,0.671428571428571,
0.685714285714285,0.699999999999999,0.714285714285714,0.728571428571428,
0.742857142857142,0.757142857142856,0.771428571428571,0.785714285714285,
0.799999999999999,0.814285714285713,0.828571428571428,0.842857142857142,
0.857142857142856,0.87142857142857,0.885714285714284,0.899999999999999,
0.914285714285713,0.928571428571427,0.942857142857141,0.957142857142856,
0.97142857142857,0.985714285714284,1.),(0.,2.1),.UNSPECIFIED.);
#215=B_SPLINE_SURFACE_WITH_KNOTS('',5,1,((#14529,#14530),(#14531,#14532),
(#14533,#14534),(#14535,#14536),(#14537,#14538),(#14539,#14540),(#14541,
#14542),(#14543,#14544),(#14545,#14546),(#14547,#14548),(#14549,#14550),
(#14551,#14552),(#14553,#14554),(#14555,#14556),(#14557,#14558),(#14559,
#14560),(#14561,#14562),(#14563,#14564),(#14565,#14566),(#14567,#14568),
(#14569,#14570),(#14571,#14572),(#14573,#14574),(#14575,#14576),(#14577,
#14578),(#14579,#14580),(#14581,#14582),(#14583,#14584),(#14585,#14586),
(#14587,#14588),(#14589,#14590),(#14591,#14592),(#14593,#14594),(#14595,
#14596),(#14597,#14598),(#14599,#14600),(#14601,#14602),(#14603,#14604),
(#14605,#14606),(#14607,#14608),(#14609,#14610),(#14611,#14612),(#14613,
#14614),(#14615,#14616),(#14617,#14618),(#14619,#14620),(#14621,#14622),
(#14623,#14624),(#14625,#14626),(#14627,#14628),(#14629,#14630),(#14631,
#14632),(#14633,#14634),(#14635,#14636),(#14637,#14638),(#14639,#14640),
(#14641,#14642),(#14643,#14644),(#14645,#14646),(#14647,#14648),(#14649,
#14650),(#14651,#14652),(#14653,#14654),(#14655,#14656),(#14657,#14658),
(#14659,#14660),(#14661,#14662),(#14663,#14664),(#14665,#14666),(#14667,
#14668),(#14669,#14670),(#14671,#14672),(#14673,#14674),(#14675,#14676),
(#14677,#14678)),.UNSPECIFIED.,.F.,.F.,.F.,(6,1,1,1,1,1,1,1,1,1,1,1,1,1,
1,1,1,1,1,1,1,1,1,1,1,1,1,1,1,1,1,1,1,1,1,1,1,1,1,1,1,1,1,1,1,1,1,1,1,1,
1,1,1,1,1,1,1,1,1,1,1,1,1,1,1,1,1,1,1,1,6),(2,2),(-1.,-0.985714285714284,
-0.97142857142857,-0.957142857142856,-0.942857142857141,-0.928571428571427,
-0.914285714285713,-0.899999999999999,-0.885714285714284,-0.87142857142857,
-0.857142857142856,-0.842857142857142,-0.828571428571428,-0.814285714285713,
-0.799999999999999,-0.785714285714285,-0.771428571428571,-0.757142857142856,
-0.742857142857142,-0.728571428571428,-0.714285714285714,-0.699999999999999,
-0.685714285714285,-0.671428571428571,-0.657142857142857,-0.642857142857142,
-0.628571428571428,-0.614285714285714,-0.6,-0.585714285714286,-0.571428571428571,
-0.557142857142857,-0.542857142857143,-0.528571428571429,-0.514285714285714,
-0.5,-0.485714285714286,-0.471428571428572,-0.457142857142857,-0.442857142857143,
-0.428571428571429,-0.414285714285714,-0.4,-0.385714285714286,-0.371428571428571,
-0.357142857142857,-0.342857142857143,-0.328571428571429,-0.314285714285714,
-0.3,-0.285714285714286,-0.271428571428571,-0.257142857142857,-0.242857142857143,
-0.228571428571429,-0.214285714285714,-0.2,-0.185714285714286,-0.171428571428571,
-0.157142857142857,-0.142857142857143,-0.128571428571429,-0.114285714285714,
-0.1,-0.0857142857142857,-0.0714285714285714,-0.0571428571428571,-0.0428571428571429,
-0.0285714285714286,-0.0142857142857143,0.),(0.,2.1),.UNSPECIFIED.);
#216=B_SPLINE_SURFACE_WITH_KNOTS('',5,1,((#14829,#14830),(#14831,#14832),
(#14833,#14834),(#14835,#14836),(#14837,#14838),(#14839,#14840),(#14841,
#14842),(#14843,#14844),(#14845,#14846),(#14847,#14848),(#14849,#14850),
(#14851,#14852),(#14853,#14854),(#14855,#14856),(#14857,#14858),(#14859,
#14860),(#14861,#14862),(#14863,#14864),(#14865,#14866),(#14867,#14868),
(#14869,#14870),(#14871,#14872),(#14873,#14874),(#14875,#14876),(#14877,
#14878),(#14879,#14880),(#14881,#14882),(#14883,#14884),(#14885,#14886),
(#14887,#14888),(#14889,#14890),(#14891,#14892),(#14893,#14894),(#14895,
#14896),(#14897,#14898),(#14899,#14900),(#14901,#14902),(#14903,#14904),
(#14905,#14906),(#14907,#14908),(#14909,#14910),(#14911,#14912),(#14913,
#14914),(#14915,#14916),(#14917,#14918),(#14919,#14920),(#14921,#14922),
(#14923,#14924),(#14925,#14926),(#14927,#14928),(#14929,#14930),(#14931,
#14932),(#14933,#14934),(#14935,#14936),(#14937,#14938),(#14939,#14940),
(#14941,#14942),(#14943,#14944),(#14945,#14946),(#14947,#14948),(#14949,
#14950),(#14951,#14952),(#14953,#14954),(#14955,#14956),(#14957,#14958),
(#14959,#14960),(#14961,#14962),(#14963,#14964),(#14965,#14966),(#14967,
#14968),(#14969,#14970),(#14971,#14972),(#14973,#14974),(#14975,#14976),
(#14977,#14978)),.UNSPECIFIED.,.F.,.F.,.F.,(6,1,1,1,1,1,1,1,1,1,1,1,1,1,
1,1,1,1,1,1,1,1,1,1,1,1,1,1,1,1,1,1,1,1,1,1,1,1,1,1,1,1,1,1,1,1,1,1,1,1,
1,1,1,1,1,1,1,1,1,1,1,1,1,1,1,1,1,1,1,1,6),(2,2),(0.,0.0142857142857143,
0.0285714285714286,0.0428571428571429,0.0571428571428571,0.0714285714285714,
0.0857142857142857,0.1,0.114285714285714,0.128571428571429,0.142857142857143,
0.157142857142857,0.171428571428571,0.185714285714286,0.2,0.214285714285714,
0.228571428571429,0.242857142857143,0.257142857142857,0.271428571428571,
0.285714285714286,0.3,0.314285714285714,0.328571428571429,0.342857142857143,
0.357142857142857,0.371428571428571,0.385714285714286,0.4,0.414285714285714,
0.428571428571429,0.442857142857143,0.457142857142857,0.471428571428572,
0.485714285714286,0.5,0.514285714285714,0.528571428571429,0.542857142857143,
0.557142857142857,0.571428571428571,0.585714285714286,0.6,0.614285714285714,
0.628571428571428,0.642857142857142,0.657142857142857,0.671428571428571,
0.685714285714285,0.699999999999999,0.714285714285714,0.728571428571428,
0.742857142857142,0.757142857142856,0.771428571428571,0.785714285714285,
0.799999999999999,0.814285714285713,0.828571428571428,0.842857142857142,
0.857142857142856,0.87142857142857,0.885714285714284,0.899999999999999,
0.914285714285713,0.928571428571427,0.942857142857141,0.957142857142856,
0.97142857142857,0.985714285714284,1.),(0.,2.1),.UNSPECIFIED.);
#217=B_SPLINE_SURFACE_WITH_KNOTS('',5,1,((#15123,#15124),(#15125,#15126),
(#15127,#15128),(#15129,#15130),(#15131,#15132),(#15133,#15134),(#15135,
#15136),(#15137,#15138),(#15139,#15140),(#15141,#15142),(#15143,#15144),
(#15145,#15146),(#15147,#15148),(#15149,#15150),(#15151,#15152),(#15153,
#15154),(#15155,#15156),(#15157,#15158),(#15159,#15160),(#15161,#15162),
(#15163,#15164),(#15165,#15166),(#15167,#15168),(#15169,#15170),(#15171,
#15172),(#15173,#15174),(#15175,#15176),(#15177,#15178),(#15179,#15180),
(#15181,#15182),(#15183,#15184),(#15185,#15186),(#15187,#15188),(#15189,
#15190),(#15191,#15192),(#15193,#15194),(#15195,#15196),(#15197,#15198),
(#15199,#15200),(#15201,#15202),(#15203,#15204),(#15205,#15206),(#15207,
#15208),(#15209,#15210),(#15211,#15212),(#15213,#15214),(#15215,#15216),
(#15217,#15218),(#15219,#15220),(#15221,#15222),(#15223,#15224),(#15225,
#15226),(#15227,#15228),(#15229,#15230),(#15231,#15232),(#15233,#15234),
(#15235,#15236),(#15237,#15238),(#15239,#15240),(#15241,#15242),(#15243,
#15244),(#15245,#15246),(#15247,#15248),(#15249,#15250),(#15251,#15252),
(#15253,#15254),(#15255,#15256),(#15257,#15258),(#15259,#15260),(#15261,
#15262),(#15263,#15264),(#15265,#15266),(#15267,#15268),(#15269,#15270),
(#15271,#15272)),.UNSPECIFIED.,.F.,.F.,.F.,(6,1,1,1,1,1,1,1,1,1,1,1,1,1,
1,1,1,1,1,1,1,1,1,1,1,1,1,1,1,1,1,1,1,1,1,1,1,1,1,1,1,1,1,1,1,1,1,1,1,1,
1,1,1,1,1,1,1,1,1,1,1,1,1,1,1,1,1,1,1,1,6),(2,2),(-1.,-0.985714285714284,
-0.97142857142857,-0.957142857142856,-0.942857142857141,-0.928571428571427,
-0.914285714285713,-0.899999999999999,-0.885714285714284,-0.87142857142857,
-0.857142857142856,-0.842857142857142,-0.828571428571428,-0.814285714285713,
-0.799999999999999,-0.785714285714285,-0.771428571428571,-0.757142857142856,
-0.742857142857142,-0.728571428571428,-0.714285714285714,-0.699999999999999,
-0.685714285714285,-0.671428571428571,-0.657142857142857,-0.642857142857142,
-0.628571428571428,-0.614285714285714,-0.6,-0.585714285714286,-0.571428571428571,
-0.557142857142857,-0.542857142857143,-0.528571428571429,-0.514285714285714,
-0.5,-0.485714285714286,-0.471428571428572,-0.457142857142857,-0.442857142857143,
-0.428571428571429,-0.414285714285714,-0.4,-0.385714285714286,-0.371428571428571,
-0.357142857142857,-0.342857142857143,-0.328571428571429,-0.314285714285714,
-0.3,-0.285714285714286,-0.271428571428571,-0.257142857142857,-0.242857142857143,
-0.228571428571429,-0.214285714285714,-0.2,-0.185714285714286,-0.171428571428571,
-0.157142857142857,-0.142857142857143,-0.128571428571429,-0.114285714285714,
-0.1,-0.0857142857142857,-0.0714285714285714,-0.0571428571428571,-0.0428571428571429,
-0.0285714285714286,-0.0142857142857143,0.),(0.,2.1),.UNSPECIFIED.);
#218=B_SPLINE_SURFACE_WITH_KNOTS('',5,1,((#15423,#15424),(#15425,#15426),
(#15427,#15428),(#15429,#15430),(#15431,#15432),(#15433,#15434),(#15435,
#15436),(#15437,#15438),(#15439,#15440),(#15441,#15442),(#15443,#15444),
(#15445,#15446),(#15447,#15448),(#15449,#15450),(#15451,#15452),(#15453,
#15454),(#15455,#15456),(#15457,#15458),(#15459,#15460),(#15461,#15462),
(#15463,#15464),(#15465,#15466),(#15467,#15468),(#15469,#15470),(#15471,
#15472),(#15473,#15474),(#15475,#15476),(#15477,#15478),(#15479,#15480),
(#15481,#15482),(#15483,#15484),(#15485,#15486),(#15487,#15488),(#15489,
#15490),(#15491,#15492),(#15493,#15494),(#15495,#15496),(#15497,#15498),
(#15499,#15500),(#15501,#15502),(#15503,#15504),(#15505,#15506),(#15507,
#15508),(#15509,#15510),(#15511,#15512),(#15513,#15514),(#15515,#15516),
(#15517,#15518),(#15519,#15520),(#15521,#15522),(#15523,#15524),(#15525,
#15526),(#15527,#15528),(#15529,#15530),(#15531,#15532),(#15533,#15534),
(#15535,#15536),(#15537,#15538),(#15539,#15540),(#15541,#15542),(#15543,
#15544),(#15545,#15546),(#15547,#15548),(#15549,#15550),(#15551,#15552),
(#15553,#15554),(#15555,#15556),(#15557,#15558),(#15559,#15560),(#15561,
#15562),(#15563,#15564),(#15565,#15566),(#15567,#15568),(#15569,#15570),
(#15571,#15572)),.UNSPECIFIED.,.F.,.F.,.F.,(6,1,1,1,1,1,1,1,1,1,1,1,1,1,
1,1,1,1,1,1,1,1,1,1,1,1,1,1,1,1,1,1,1,1,1,1,1,1,1,1,1,1,1,1,1,1,1,1,1,1,
1,1,1,1,1,1,1,1,1,1,1,1,1,1,1,1,1,1,1,1,6),(2,2),(0.,0.0142857142857143,
0.0285714285714286,0.0428571428571429,0.0571428571428571,0.0714285714285714,
0.0857142857142857,0.1,0.114285714285714,0.128571428571429,0.142857142857143,
0.157142857142857,0.171428571428571,0.185714285714286,0.2,0.214285714285714,
0.228571428571429,0.242857142857143,0.257142857142857,0.271428571428571,
0.285714285714286,0.3,0.314285714285714,0.328571428571429,0.342857142857143,
0.357142857142857,0.371428571428571,0.385714285714286,0.4,0.414285714285714,
0.428571428571429,0.442857142857143,0.457142857142857,0.471428571428572,
0.485714285714286,0.5,0.514285714285714,0.528571428571429,0.542857142857143,
0.557142857142857,0.571428571428571,0.585714285714286,0.6,0.614285714285714,
0.628571428571428,0.642857142857142,0.657142857142857,0.671428571428571,
0.685714285714285,0.699999999999999,0.714285714285714,0.728571428571428,
0.742857142857142,0.757142857142856,0.771428571428571,0.785714285714285,
0.799999999999999,0.814285714285713,0.828571428571428,0.842857142857142,
0.857142857142856,0.87142857142857,0.885714285714284,0.899999999999999,
0.914285714285713,0.928571428571427,0.942857142857141,0.957142857142856,
0.97142857142857,0.985714285714284,1.),(0.,2.1),.UNSPECIFIED.);
#219=B_SPLINE_SURFACE_WITH_KNOTS('',5,1,((#15717,#15718),(#15719,#15720),
(#15721,#15722),(#15723,#15724),(#15725,#15726),(#15727,#15728),(#15729,
#15730),(#15731,#15732),(#15733,#15734),(#15735,#15736),(#15737,#15738),
(#15739,#15740),(#15741,#15742),(#15743,#15744),(#15745,#15746),(#15747,
#15748),(#15749,#15750),(#15751,#15752),(#15753,#15754),(#15755,#15756),
(#15757,#15758),(#15759,#15760),(#15761,#15762),(#15763,#15764),(#15765,
#15766),(#15767,#15768),(#15769,#15770),(#15771,#15772),(#15773,#15774),
(#15775,#15776),(#15777,#15778),(#15779,#15780),(#15781,#15782),(#15783,
#15784),(#15785,#15786),(#15787,#15788),(#15789,#15790),(#15791,#15792),
(#15793,#15794),(#15795,#15796),(#15797,#15798),(#15799,#15800),(#15801,
#15802),(#15803,#15804),(#15805,#15806),(#15807,#15808),(#15809,#15810),
(#15811,#15812),(#15813,#15814),(#15815,#15816),(#15817,#15818),(#15819,
#15820),(#15821,#15822),(#15823,#15824),(#15825,#15826),(#15827,#15828),
(#15829,#15830),(#15831,#15832),(#15833,#15834),(#15835,#15836),(#15837,
#15838),(#15839,#15840),(#15841,#15842),(#15843,#15844),(#15845,#15846),
(#15847,#15848),(#15849,#15850),(#15851,#15852),(#15853,#15854),(#15855,
#15856),(#15857,#15858),(#15859,#15860),(#15861,#15862),(#15863,#15864),
(#15865,#15866)),.UNSPECIFIED.,.F.,.F.,.F.,(6,1,1,1,1,1,1,1,1,1,1,1,1,1,
1,1,1,1,1,1,1,1,1,1,1,1,1,1,1,1,1,1,1,1,1,1,1,1,1,1,1,1,1,1,1,1,1,1,1,1,
1,1,1,1,1,1,1,1,1,1,1,1,1,1,1,1,1,1,1,1,6),(2,2),(-1.,-0.985714285714284,
-0.97142857142857,-0.957142857142856,-0.942857142857141,-0.928571428571427,
-0.914285714285713,-0.899999999999999,-0.885714285714284,-0.87142857142857,
-0.857142857142856,-0.842857142857142,-0.828571428571428,-0.814285714285713,
-0.799999999999999,-0.785714285714285,-0.771428571428571,-0.757142857142856,
-0.742857142857142,-0.728571428571428,-0.714285714285714,-0.699999999999999,
-0.685714285714285,-0.671428571428571,-0.657142857142857,-0.642857142857142,
-0.628571428571428,-0.614285714285714,-0.6,-0.585714285714286,-0.571428571428571,
-0.557142857142857,-0.542857142857143,-0.528571428571429,-0.514285714285714,
-0.5,-0.485714285714286,-0.471428571428572,-0.457142857142857,-0.442857142857143,
-0.428571428571429,-0.414285714285714,-0.4,-0.385714285714286,-0.371428571428571,
-0.357142857142857,-0.342857142857143,-0.328571428571429,-0.314285714285714,
-0.3,-0.285714285714286,-0.271428571428571,-0.257142857142857,-0.242857142857143,
-0.228571428571429,-0.214285714285714,-0.2,-0.185714285714286,-0.171428571428571,
-0.157142857142857,-0.142857142857143,-0.128571428571429,-0.114285714285714,
-0.1,-0.0857142857142857,-0.0714285714285714,-0.0571428571428571,-0.0428571428571429,
-0.0285714285714286,-0.0142857142857143,0.),(0.,2.1),.UNSPECIFIED.);
#220=B_SPLINE_SURFACE_WITH_KNOTS('',5,1,((#16017,#16018),(#16019,#16020),
(#16021,#16022),(#16023,#16024),(#16025,#16026),(#16027,#16028),(#16029,
#16030),(#16031,#16032),(#16033,#16034),(#16035,#16036),(#16037,#16038),
(#16039,#16040),(#16041,#16042),(#16043,#16044),(#16045,#16046),(#16047,
#16048),(#16049,#16050),(#16051,#16052),(#16053,#16054),(#16055,#16056),
(#16057,#16058),(#16059,#16060),(#16061,#16062),(#16063,#16064),(#16065,
#16066),(#16067,#16068),(#16069,#16070),(#16071,#16072),(#16073,#16074),
(#16075,#16076),(#16077,#16078),(#16079,#16080),(#16081,#16082),(#16083,
#16084),(#16085,#16086),(#16087,#16088),(#16089,#16090),(#16091,#16092),
(#16093,#16094),(#16095,#16096),(#16097,#16098),(#16099,#16100),(#16101,
#16102),(#16103,#16104),(#16105,#16106),(#16107,#16108),(#16109,#16110),
(#16111,#16112),(#16113,#16114),(#16115,#16116),(#16117,#16118),(#16119,
#16120),(#16121,#16122),(#16123,#16124),(#16125,#16126),(#16127,#16128),
(#16129,#16130),(#16131,#16132),(#16133,#16134),(#16135,#16136),(#16137,
#16138),(#16139,#16140),(#16141,#16142),(#16143,#16144),(#16145,#16146),
(#16147,#16148),(#16149,#16150),(#16151,#16152),(#16153,#16154),(#16155,
#16156),(#16157,#16158),(#16159,#16160),(#16161,#16162),(#16163,#16164),
(#16165,#16166)),.UNSPECIFIED.,.F.,.F.,.F.,(6,1,1,1,1,1,1,1,1,1,1,1,1,1,
1,1,1,1,1,1,1,1,1,1,1,1,1,1,1,1,1,1,1,1,1,1,1,1,1,1,1,1,1,1,1,1,1,1,1,1,
1,1,1,1,1,1,1,1,1,1,1,1,1,1,1,1,1,1,1,1,6),(2,2),(0.,0.0142857142857143,
0.0285714285714286,0.0428571428571429,0.0571428571428571,0.0714285714285714,
0.0857142857142857,0.1,0.114285714285714,0.128571428571429,0.142857142857143,
0.157142857142857,0.171428571428571,0.185714285714286,0.2,0.214285714285714,
0.228571428571429,0.242857142857143,0.257142857142857,0.271428571428571,
0.285714285714286,0.3,0.314285714285714,0.328571428571429,0.342857142857143,
0.357142857142857,0.371428571428571,0.385714285714286,0.4,0.414285714285714,
0.428571428571429,0.442857142857143,0.457142857142857,0.471428571428572,
0.485714285714286,0.5,0.514285714285714,0.528571428571429,0.542857142857143,
0.557142857142857,0.571428571428571,0.585714285714286,0.6,0.614285714285714,
0.628571428571428,0.642857142857142,0.657142857142857,0.671428571428571,
0.685714285714285,0.699999999999999,0.714285714285714,0.728571428571428,
0.742857142857142,0.757142857142856,0.771428571428571,0.785714285714285,
0.799999999999999,0.814285714285713,0.828571428571428,0.842857142857142,
0.857142857142856,0.87142857142857,0.885714285714284,0.899999999999999,
0.914285714285713,0.928571428571427,0.942857142857141,0.957142857142856,
0.97142857142857,0.985714285714284,1.),(0.,2.1),.UNSPECIFIED.);
#221=B_SPLINE_SURFACE_WITH_KNOTS('',5,1,((#16311,#16312),(#16313,#16314),
(#16315,#16316),(#16317,#16318),(#16319,#16320),(#16321,#16322),(#16323,
#16324),(#16325,#16326),(#16327,#16328),(#16329,#16330),(#16331,#16332),
(#16333,#16334),(#16335,#16336),(#16337,#16338),(#16339,#16340),(#16341,
#16342),(#16343,#16344),(#16345,#16346),(#16347,#16348),(#16349,#16350),
(#16351,#16352),(#16353,#16354),(#16355,#16356),(#16357,#16358),(#16359,
#16360),(#16361,#16362),(#16363,#16364),(#16365,#16366),(#16367,#16368),
(#16369,#16370),(#16371,#16372),(#16373,#16374),(#16375,#16376),(#16377,
#16378),(#16379,#16380),(#16381,#16382),(#16383,#16384),(#16385,#16386),
(#16387,#16388),(#16389,#16390),(#16391,#16392),(#16393,#16394),(#16395,
#16396),(#16397,#16398),(#16399,#16400),(#16401,#16402),(#16403,#16404),
(#16405,#16406),(#16407,#16408),(#16409,#16410),(#16411,#16412),(#16413,
#16414),(#16415,#16416),(#16417,#16418),(#16419,#16420),(#16421,#16422),
(#16423,#16424),(#16425,#16426),(#16427,#16428),(#16429,#16430),(#16431,
#16432),(#16433,#16434),(#16435,#16436),(#16437,#16438),(#16439,#16440),
(#16441,#16442),(#16443,#16444),(#16445,#16446),(#16447,#16448),(#16449,
#16450),(#16451,#16452),(#16453,#16454),(#16455,#16456),(#16457,#16458),
(#16459,#16460)),.UNSPECIFIED.,.F.,.F.,.F.,(6,1,1,1,1,1,1,1,1,1,1,1,1,1,
1,1,1,1,1,1,1,1,1,1,1,1,1,1,1,1,1,1,1,1,1,1,1,1,1,1,1,1,1,1,1,1,1,1,1,1,
1,1,1,1,1,1,1,1,1,1,1,1,1,1,1,1,1,1,1,1,6),(2,2),(-1.,-0.985714285714284,
-0.97142857142857,-0.957142857142856,-0.942857142857141,-0.928571428571427,
-0.914285714285713,-0.899999999999999,-0.885714285714284,-0.87142857142857,
-0.857142857142856,-0.842857142857142,-0.828571428571428,-0.814285714285713,
-0.799999999999999,-0.785714285714285,-0.771428571428571,-0.757142857142856,
-0.742857142857142,-0.728571428571428,-0.714285714285714,-0.699999999999999,
-0.685714285714285,-0.671428571428571,-0.657142857142857,-0.642857142857142,
-0.628571428571428,-0.614285714285714,-0.6,-0.585714285714286,-0.571428571428571,
-0.557142857142857,-0.542857142857143,-0.528571428571429,-0.514285714285714,
-0.5,-0.485714285714286,-0.471428571428572,-0.457142857142857,-0.442857142857143,
-0.428571428571429,-0.414285714285714,-0.4,-0.385714285714286,-0.371428571428571,
-0.357142857142857,-0.342857142857143,-0.328571428571429,-0.314285714285714,
-0.3,-0.285714285714286,-0.271428571428571,-0.257142857142857,-0.242857142857143,
-0.228571428571429,-0.214285714285714,-0.2,-0.185714285714286,-0.171428571428571,
-0.157142857142857,-0.142857142857143,-0.128571428571429,-0.114285714285714,
-0.1,-0.0857142857142857,-0.0714285714285714,-0.0571428571428571,-0.0428571428571429,
-0.0285714285714286,-0.0142857142857143,0.),(0.,2.1),.UNSPECIFIED.);
#222=B_SPLINE_SURFACE_WITH_KNOTS('',5,1,((#16611,#16612),(#16613,#16614),
(#16615,#16616),(#16617,#16618),(#16619,#16620),(#16621,#16622),(#16623,
#16624),(#16625,#16626),(#16627,#16628),(#16629,#16630),(#16631,#16632),
(#16633,#16634),(#16635,#16636),(#16637,#16638),(#16639,#16640),(#16641,
#16642),(#16643,#16644),(#16645,#16646),(#16647,#16648),(#16649,#16650),
(#16651,#16652),(#16653,#16654),(#16655,#16656),(#16657,#16658),(#16659,
#16660),(#16661,#16662),(#16663,#16664),(#16665,#16666),(#16667,#16668),
(#16669,#16670),(#16671,#16672),(#16673,#16674),(#16675,#16676),(#16677,
#16678),(#16679,#16680),(#16681,#16682),(#16683,#16684),(#16685,#16686),
(#16687,#16688),(#16689,#16690),(#16691,#16692),(#16693,#16694),(#16695,
#16696),(#16697,#16698),(#16699,#16700),(#16701,#16702),(#16703,#16704),
(#16705,#16706),(#16707,#16708),(#16709,#16710),(#16711,#16712),(#16713,
#16714),(#16715,#16716),(#16717,#16718),(#16719,#16720),(#16721,#16722),
(#16723,#16724),(#16725,#16726),(#16727,#16728),(#16729,#16730),(#16731,
#16732),(#16733,#16734),(#16735,#16736),(#16737,#16738),(#16739,#16740),
(#16741,#16742),(#16743,#16744),(#16745,#16746),(#16747,#16748),(#16749,
#16750),(#16751,#16752),(#16753,#16754),(#16755,#16756),(#16757,#16758),
(#16759,#16760)),.UNSPECIFIED.,.F.,.F.,.F.,(6,1,1,1,1,1,1,1,1,1,1,1,1,1,
1,1,1,1,1,1,1,1,1,1,1,1,1,1,1,1,1,1,1,1,1,1,1,1,1,1,1,1,1,1,1,1,1,1,1,1,
1,1,1,1,1,1,1,1,1,1,1,1,1,1,1,1,1,1,1,1,6),(2,2),(0.,0.0142857142857143,
0.0285714285714286,0.0428571428571429,0.0571428571428571,0.0714285714285714,
0.0857142857142857,0.1,0.114285714285714,0.128571428571429,0.142857142857143,
0.157142857142857,0.171428571428571,0.185714285714286,0.2,0.214285714285714,
0.228571428571429,0.242857142857143,0.257142857142857,0.271428571428571,
0.285714285714286,0.3,0.314285714285714,0.328571428571429,0.342857142857143,
0.357142857142857,0.371428571428571,0.385714285714286,0.4,0.414285714285714,
0.428571428571429,0.442857142857143,0.457142857142857,0.471428571428572,
0.485714285714286,0.5,0.514285714285714,0.528571428571429,0.542857142857143,
0.557142857142857,0.571428571428571,0.585714285714286,0.6,0.614285714285714,
0.628571428571428,0.642857142857142,0.657142857142857,0.671428571428571,
0.685714285714285,0.699999999999999,0.714285714285714,0.728571428571428,
0.742857142857142,0.757142857142856,0.771428571428571,0.785714285714285,
0.799999999999999,0.814285714285713,0.828571428571428,0.842857142857142,
0.857142857142856,0.87142857142857,0.885714285714284,0.899999999999999,
0.914285714285713,0.928571428571427,0.942857142857141,0.957142857142856,
0.97142857142857,0.985714285714284,1.),(0.,2.1),.UNSPECIFIED.);
#223=B_SPLINE_SURFACE_WITH_KNOTS('',5,1,((#16905,#16906),(#16907,#16908),
(#16909,#16910),(#16911,#16912),(#16913,#16914),(#16915,#16916),(#16917,
#16918),(#16919,#16920),(#16921,#16922),(#16923,#16924),(#16925,#16926),
(#16927,#16928),(#16929,#16930),(#16931,#16932),(#16933,#16934),(#16935,
#16936),(#16937,#16938),(#16939,#16940),(#16941,#16942),(#16943,#16944),
(#16945,#16946),(#16947,#16948),(#16949,#16950),(#16951,#16952),(#16953,
#16954),(#16955,#16956),(#16957,#16958),(#16959,#16960),(#16961,#16962),
(#16963,#16964),(#16965,#16966),(#16967,#16968),(#16969,#16970),(#16971,
#16972),(#16973,#16974),(#16975,#16976),(#16977,#16978),(#16979,#16980),
(#16981,#16982),(#16983,#16984),(#16985,#16986),(#16987,#16988),(#16989,
#16990),(#16991,#16992),(#16993,#16994),(#16995,#16996),(#16997,#16998),
(#16999,#17000),(#17001,#17002),(#17003,#17004),(#17005,#17006),(#17007,
#17008),(#17009,#17010),(#17011,#17012),(#17013,#17014),(#17015,#17016),
(#17017,#17018),(#17019,#17020),(#17021,#17022),(#17023,#17024),(#17025,
#17026),(#17027,#17028),(#17029,#17030),(#17031,#17032),(#17033,#17034),
(#17035,#17036),(#17037,#17038),(#17039,#17040),(#17041,#17042),(#17043,
#17044),(#17045,#17046),(#17047,#17048),(#17049,#17050),(#17051,#17052),
(#17053,#17054)),.UNSPECIFIED.,.F.,.F.,.F.,(6,1,1,1,1,1,1,1,1,1,1,1,1,1,
1,1,1,1,1,1,1,1,1,1,1,1,1,1,1,1,1,1,1,1,1,1,1,1,1,1,1,1,1,1,1,1,1,1,1,1,
1,1,1,1,1,1,1,1,1,1,1,1,1,1,1,1,1,1,1,1,6),(2,2),(-1.,-0.985714285714284,
-0.97142857142857,-0.957142857142856,-0.942857142857141,-0.928571428571427,
-0.914285714285713,-0.899999999999999,-0.885714285714284,-0.87142857142857,
-0.857142857142856,-0.842857142857142,-0.828571428571428,-0.814285714285713,
-0.799999999999999,-0.785714285714285,-0.771428571428571,-0.757142857142856,
-0.742857142857142,-0.728571428571428,-0.714285714285714,-0.699999999999999,
-0.685714285714285,-0.671428571428571,-0.657142857142857,-0.642857142857142,
-0.628571428571428,-0.614285714285714,-0.6,-0.585714285714286,-0.571428571428571,
-0.557142857142857,-0.542857142857143,-0.528571428571429,-0.514285714285714,
-0.5,-0.485714285714286,-0.471428571428572,-0.457142857142857,-0.442857142857143,
-0.428571428571429,-0.414285714285714,-0.4,-0.385714285714286,-0.371428571428571,
-0.357142857142857,-0.342857142857143,-0.328571428571429,-0.314285714285714,
-0.3,-0.285714285714286,-0.271428571428571,-0.257142857142857,-0.242857142857143,
-0.228571428571429,-0.214285714285714,-0.2,-0.185714285714286,-0.171428571428571,
-0.157142857142857,-0.142857142857143,-0.128571428571429,-0.114285714285714,
-0.1,-0.0857142857142857,-0.0714285714285714,-0.0571428571428571,-0.0428571428571429,
-0.0285714285714286,-0.0142857142857143,0.),(0.,2.1),.UNSPECIFIED.);
#224=B_SPLINE_SURFACE_WITH_KNOTS('',5,1,((#17220,#17221),(#17222,#17223),
(#17224,#17225),(#17226,#17227),(#17228,#17229),(#17230,#17231),(#17232,
#17233),(#17234,#17235),(#17236,#17237),(#17238,#17239),(#17240,#17241),
(#17242,#17243),(#17244,#17245),(#17246,#17247),(#17248,#17249),(#17250,
#17251),(#17252,#17253),(#17254,#17255),(#17256,#17257),(#17258,#17259),
(#17260,#17261),(#17262,#17263),(#17264,#17265),(#17266,#17267),(#17268,
#17269),(#17270,#17271),(#17272,#17273),(#17274,#17275),(#17276,#17277),
(#17278,#17279),(#17280,#17281),(#17282,#17283),(#17284,#17285),(#17286,
#17287),(#17288,#17289),(#17290,#17291),(#17292,#17293),(#17294,#17295),
(#17296,#17297),(#17298,#17299),(#17300,#17301),(#17302,#17303),(#17304,
#17305),(#17306,#17307),(#17308,#17309),(#17310,#17311),(#17312,#17313),
(#17314,#17315),(#17316,#17317),(#17318,#17319),(#17320,#17321),(#17322,
#17323),(#17324,#17325),(#17326,#17327),(#17328,#17329),(#17330,#17331),
(#17332,#17333),(#17334,#17335),(#17336,#17337),(#17338,#17339),(#17340,
#17341),(#17342,#17343),(#17344,#17345),(#17346,#17347),(#17348,#17349),
(#17350,#17351),(#17352,#17353),(#17354,#17355),(#17356,#17357),(#17358,
#17359),(#17360,#17361),(#17362,#17363),(#17364,#17365),(#17366,#17367),
(#17368,#17369)),.UNSPECIFIED.,.F.,.F.,.F.,(6,1,1,1,1,1,1,1,1,1,1,1,1,1,
1,1,1,1,1,1,1,1,1,1,1,1,1,1,1,1,1,1,1,1,1,1,1,1,1,1,1,1,1,1,1,1,1,1,1,1,
1,1,1,1,1,1,1,1,1,1,1,1,1,1,1,1,1,1,1,1,6),(2,2),(0.,0.0142857142857143,
0.0285714285714286,0.0428571428571429,0.0571428571428571,0.0714285714285714,
0.0857142857142857,0.1,0.114285714285714,0.128571428571429,0.142857142857143,
0.157142857142857,0.171428571428571,0.185714285714286,0.2,0.214285714285714,
0.228571428571429,0.242857142857143,0.257142857142857,0.271428571428571,
0.285714285714286,0.3,0.314285714285714,0.328571428571429,0.342857142857143,
0.357142857142857,0.371428571428571,0.385714285714286,0.4,0.414285714285714,
0.428571428571429,0.442857142857143,0.457142857142857,0.471428571428572,
0.485714285714286,0.5,0.514285714285714,0.528571428571429,0.542857142857143,
0.557142857142857,0.571428571428571,0.585714285714286,0.6,0.614285714285714,
0.628571428571428,0.642857142857142,0.657142857142857,0.671428571428571,
0.685714285714285,0.699999999999999,0.714285714285714,0.728571428571428,
0.742857142857142,0.757142857142856,0.771428571428571,0.785714285714285,
0.799999999999999,0.814285714285713,0.828571428571428,0.842857142857142,
0.857142857142856,0.87142857142857,0.885714285714284,0.899999999999999,
0.914285714285713,0.928571428571427,0.942857142857141,0.957142857142856,
0.97142857142857,0.985714285714284,1.),(0.,2.1),.UNSPECIFIED.);
#225=B_SPLINE_SURFACE_WITH_KNOTS('',5,1,((#17514,#17515),(#17516,#17517),
(#17518,#17519),(#17520,#17521),(#17522,#17523),(#17524,#17525),(#17526,
#17527),(#17528,#17529),(#17530,#17531),(#17532,#17533),(#17534,#17535),
(#17536,#17537),(#17538,#17539),(#17540,#17541),(#17542,#17543),(#17544,
#17545),(#17546,#17547),(#17548,#17549),(#17550,#17551),(#17552,#17553),
(#17554,#17555),(#17556,#17557),(#17558,#17559),(#17560,#17561),(#17562,
#17563),(#17564,#17565),(#17566,#17567),(#17568,#17569),(#17570,#17571),
(#17572,#17573),(#17574,#17575),(#17576,#17577),(#17578,#17579),(#17580,
#17581),(#17582,#17583),(#17584,#17585),(#17586,#17587),(#17588,#17589),
(#17590,#17591),(#17592,#17593),(#17594,#17595),(#17596,#17597),(#17598,
#17599),(#17600,#17601),(#17602,#17603),(#17604,#17605),(#17606,#17607),
(#17608,#17609),(#17610,#17611),(#17612,#17613),(#17614,#17615),(#17616,
#17617),(#17618,#17619),(#17620,#17621),(#17622,#17623),(#17624,#17625),
(#17626,#17627),(#17628,#17629),(#17630,#17631),(#17632,#17633),(#17634,
#17635),(#17636,#17637),(#17638,#17639),(#17640,#17641),(#17642,#17643),
(#17644,#17645),(#17646,#17647),(#17648,#17649),(#17650,#17651),(#17652,
#17653),(#17654,#17655),(#17656,#17657),(#17658,#17659),(#17660,#17661),
(#17662,#17663)),.UNSPECIFIED.,.F.,.F.,.F.,(6,1,1,1,1,1,1,1,1,1,1,1,1,1,
1,1,1,1,1,1,1,1,1,1,1,1,1,1,1,1,1,1,1,1,1,1,1,1,1,1,1,1,1,1,1,1,1,1,1,1,
1,1,1,1,1,1,1,1,1,1,1,1,1,1,1,1,1,1,1,1,6),(2,2),(-1.,-0.985714285714284,
-0.97142857142857,-0.957142857142856,-0.942857142857141,-0.928571428571427,
-0.914285714285713,-0.899999999999999,-0.885714285714284,-0.87142857142857,
-0.857142857142856,-0.842857142857142,-0.828571428571428,-0.814285714285713,
-0.799999999999999,-0.785714285714285,-0.771428571428571,-0.757142857142856,
-0.742857142857142,-0.728571428571428,-0.714285714285714,-0.699999999999999,
-0.685714285714285,-0.671428571428571,-0.657142857142857,-0.642857142857142,
-0.628571428571428,-0.614285714285714,-0.6,-0.585714285714286,-0.571428571428571,
-0.557142857142857,-0.542857142857143,-0.528571428571429,-0.514285714285714,
-0.5,-0.485714285714286,-0.471428571428572,-0.457142857142857,-0.442857142857143,
-0.428571428571429,-0.414285714285714,-0.4,-0.385714285714286,-0.371428571428571,
-0.357142857142857,-0.342857142857143,-0.328571428571429,-0.314285714285714,
-0.3,-0.285714285714286,-0.271428571428571,-0.257142857142857,-0.242857142857143,
-0.228571428571429,-0.214285714285714,-0.2,-0.185714285714286,-0.171428571428571,
-0.157142857142857,-0.142857142857143,-0.128571428571429,-0.114285714285714,
-0.1,-0.0857142857142857,-0.0714285714285714,-0.0571428571428571,-0.0428571428571429,
-0.0285714285714286,-0.0142857142857143,0.),(0.,2.1),.UNSPECIFIED.);
#226=B_SPLINE_SURFACE_WITH_KNOTS('',5,1,((#17814,#17815),(#17816,#17817),
(#17818,#17819),(#17820,#17821),(#17822,#17823),(#17824,#17825),(#17826,
#17827),(#17828,#17829),(#17830,#17831),(#17832,#17833),(#17834,#17835),
(#17836,#17837),(#17838,#17839),(#17840,#17841),(#17842,#17843),(#17844,
#17845),(#17846,#17847),(#17848,#17849),(#17850,#17851),(#17852,#17853),
(#17854,#17855),(#17856,#17857),(#17858,#17859),(#17860,#17861),(#17862,
#17863),(#17864,#17865),(#17866,#17867),(#17868,#17869),(#17870,#17871),
(#17872,#17873),(#17874,#17875),(#17876,#17877),(#17878,#17879),(#17880,
#17881),(#17882,#17883),(#17884,#17885),(#17886,#17887),(#17888,#17889),
(#17890,#17891),(#17892,#17893),(#17894,#17895),(#17896,#17897),(#17898,
#17899),(#17900,#17901),(#17902,#17903),(#17904,#17905),(#17906,#17907),
(#17908,#17909),(#17910,#17911),(#17912,#17913),(#17914,#17915),(#17916,
#17917),(#17918,#17919),(#17920,#17921),(#17922,#17923),(#17924,#17925),
(#17926,#17927),(#17928,#17929),(#17930,#17931),(#17932,#17933),(#17934,
#17935),(#17936,#17937),(#17938,#17939),(#17940,#17941),(#17942,#17943),
(#17944,#17945),(#17946,#17947),(#17948,#17949),(#17950,#17951),(#17952,
#17953),(#17954,#17955),(#17956,#17957),(#17958,#17959),(#17960,#17961),
(#17962,#17963)),.UNSPECIFIED.,.F.,.F.,.F.,(6,1,1,1,1,1,1,1,1,1,1,1,1,1,
1,1,1,1,1,1,1,1,1,1,1,1,1,1,1,1,1,1,1,1,1,1,1,1,1,1,1,1,1,1,1,1,1,1,1,1,
1,1,1,1,1,1,1,1,1,1,1,1,1,1,1,1,1,1,1,1,6),(2,2),(0.,0.0142857142857143,
0.0285714285714286,0.0428571428571429,0.0571428571428571,0.0714285714285714,
0.0857142857142857,0.1,0.114285714285714,0.128571428571429,0.142857142857143,
0.157142857142857,0.171428571428571,0.185714285714286,0.2,0.214285714285714,
0.228571428571429,0.242857142857143,0.257142857142857,0.271428571428571,
0.285714285714286,0.3,0.314285714285714,0.328571428571429,0.342857142857143,
0.357142857142857,0.371428571428571,0.385714285714286,0.4,0.414285714285714,
0.428571428571429,0.442857142857143,0.457142857142857,0.471428571428572,
0.485714285714286,0.5,0.514285714285714,0.528571428571429,0.542857142857143,
0.557142857142857,0.571428571428571,0.585714285714286,0.6,0.614285714285714,
0.628571428571428,0.642857142857142,0.657142857142857,0.671428571428571,
0.685714285714285,0.699999999999999,0.714285714285714,0.728571428571428,
0.742857142857142,0.757142857142856,0.771428571428571,0.785714285714285,
0.799999999999999,0.814285714285713,0.828571428571428,0.842857142857142,
0.857142857142856,0.87142857142857,0.885714285714284,0.899999999999999,
0.914285714285713,0.928571428571427,0.942857142857141,0.957142857142856,
0.97142857142857,0.985714285714284,1.),(0.,2.1),.UNSPECIFIED.);
#227=B_SPLINE_SURFACE_WITH_KNOTS('',5,1,((#18108,#18109),(#18110,#18111),
(#18112,#18113),(#18114,#18115),(#18116,#18117),(#18118,#18119),(#18120,
#18121),(#18122,#18123),(#18124,#18125),(#18126,#18127),(#18128,#18129),
(#18130,#18131),(#18132,#18133),(#18134,#18135),(#18136,#18137),(#18138,
#18139),(#18140,#18141),(#18142,#18143),(#18144,#18145),(#18146,#18147),
(#18148,#18149),(#18150,#18151),(#18152,#18153),(#18154,#18155),(#18156,
#18157),(#18158,#18159),(#18160,#18161),(#18162,#18163),(#18164,#18165),
(#18166,#18167),(#18168,#18169),(#18170,#18171),(#18172,#18173),(#18174,
#18175),(#18176,#18177),(#18178,#18179),(#18180,#18181),(#18182,#18183),
(#18184,#18185),(#18186,#18187),(#18188,#18189),(#18190,#18191),(#18192,
#18193),(#18194,#18195),(#18196,#18197),(#18198,#18199),(#18200,#18201),
(#18202,#18203),(#18204,#18205),(#18206,#18207),(#18208,#18209),(#18210,
#18211),(#18212,#18213),(#18214,#18215),(#18216,#18217),(#18218,#18219),
(#18220,#18221),(#18222,#18223),(#18224,#18225),(#18226,#18227),(#18228,
#18229),(#18230,#18231),(#18232,#18233),(#18234,#18235),(#18236,#18237),
(#18238,#18239),(#18240,#18241),(#18242,#18243),(#18244,#18245),(#18246,
#18247),(#18248,#18249),(#18250,#18251),(#18252,#18253),(#18254,#18255),
(#18256,#18257)),.UNSPECIFIED.,.F.,.F.,.F.,(6,1,1,1,1,1,1,1,1,1,1,1,1,1,
1,1,1,1,1,1,1,1,1,1,1,1,1,1,1,1,1,1,1,1,1,1,1,1,1,1,1,1,1,1,1,1,1,1,1,1,
1,1,1,1,1,1,1,1,1,1,1,1,1,1,1,1,1,1,1,1,6),(2,2),(-1.,-0.985714285714284,
-0.97142857142857,-0.957142857142856,-0.942857142857141,-0.928571428571427,
-0.914285714285713,-0.899999999999999,-0.885714285714284,-0.87142857142857,
-0.857142857142856,-0.842857142857142,-0.828571428571428,-0.814285714285713,
-0.799999999999999,-0.785714285714285,-0.771428571428571,-0.757142857142856,
-0.742857142857142,-0.728571428571428,-0.714285714285714,-0.699999999999999,
-0.685714285714285,-0.671428571428571,-0.657142857142857,-0.642857142857142,
-0.628571428571428,-0.614285714285714,-0.6,-0.585714285714286,-0.571428571428571,
-0.557142857142857,-0.542857142857143,-0.528571428571429,-0.514285714285714,
-0.5,-0.485714285714286,-0.471428571428572,-0.457142857142857,-0.442857142857143,
-0.428571428571429,-0.414285714285714,-0.4,-0.385714285714286,-0.371428571428571,
-0.357142857142857,-0.342857142857143,-0.328571428571429,-0.314285714285714,
-0.3,-0.285714285714286,-0.271428571428571,-0.257142857142857,-0.242857142857143,
-0.228571428571429,-0.214285714285714,-0.2,-0.185714285714286,-0.171428571428571,
-0.157142857142857,-0.142857142857143,-0.128571428571429,-0.114285714285714,
-0.1,-0.0857142857142857,-0.0714285714285714,-0.0571428571428571,-0.0428571428571429,
-0.0285714285714286,-0.0142857142857143,0.),(0.,2.1),.UNSPECIFIED.);
#228=B_SPLINE_SURFACE_WITH_KNOTS('',5,1,((#18408,#18409),(#18410,#18411),
(#18412,#18413),(#18414,#18415),(#18416,#18417),(#18418,#18419),(#18420,
#18421),(#18422,#18423),(#18424,#18425),(#18426,#18427),(#18428,#18429),
(#18430,#18431),(#18432,#18433),(#18434,#18435),(#18436,#18437),(#18438,
#18439),(#18440,#18441),(#18442,#18443),(#18444,#18445),(#18446,#18447),
(#18448,#18449),(#18450,#18451),(#18452,#18453),(#18454,#18455),(#18456,
#18457),(#18458,#18459),(#18460,#18461),(#18462,#18463),(#18464,#18465),
(#18466,#18467),(#18468,#18469),(#18470,#18471),(#18472,#18473),(#18474,
#18475),(#18476,#18477),(#18478,#18479),(#18480,#18481),(#18482,#18483),
(#18484,#18485),(#18486,#18487),(#18488,#18489),(#18490,#18491),(#18492,
#18493),(#18494,#18495),(#18496,#18497),(#18498,#18499),(#18500,#18501),
(#18502,#18503),(#18504,#18505),(#18506,#18507),(#18508,#18509),(#18510,
#18511),(#18512,#18513),(#18514,#18515),(#18516,#18517),(#18518,#18519),
(#18520,#18521),(#18522,#18523),(#18524,#18525),(#18526,#18527),(#18528,
#18529),(#18530,#18531),(#18532,#18533),(#18534,#18535),(#18536,#18537),
(#18538,#18539),(#18540,#18541),(#18542,#18543),(#18544,#18545),(#18546,
#18547),(#18548,#18549),(#18550,#18551),(#18552,#18553),(#18554,#18555),
(#18556,#18557)),.UNSPECIFIED.,.F.,.F.,.F.,(6,1,1,1,1,1,1,1,1,1,1,1,1,1,
1,1,1,1,1,1,1,1,1,1,1,1,1,1,1,1,1,1,1,1,1,1,1,1,1,1,1,1,1,1,1,1,1,1,1,1,
1,1,1,1,1,1,1,1,1,1,1,1,1,1,1,1,1,1,1,1,6),(2,2),(0.,0.0142857142857143,
0.0285714285714286,0.0428571428571429,0.0571428571428571,0.0714285714285714,
0.0857142857142857,0.1,0.114285714285714,0.128571428571429,0.142857142857143,
0.157142857142857,0.171428571428571,0.185714285714286,0.2,0.214285714285714,
0.228571428571429,0.242857142857143,0.257142857142857,0.271428571428571,
0.285714285714286,0.3,0.314285714285714,0.328571428571429,0.342857142857143,
0.357142857142857,0.371428571428571,0.385714285714286,0.4,0.414285714285714,
0.428571428571429,0.442857142857143,0.457142857142857,0.471428571428572,
0.485714285714286,0.5,0.514285714285714,0.528571428571429,0.542857142857143,
0.557142857142857,0.571428571428571,0.585714285714286,0.6,0.614285714285714,
0.628571428571428,0.642857142857142,0.657142857142857,0.671428571428571,
0.685714285714285,0.699999999999999,0.714285714285714,0.728571428571428,
0.742857142857142,0.757142857142856,0.771428571428571,0.785714285714285,
0.799999999999999,0.814285714285713,0.828571428571428,0.842857142857142,
0.857142857142856,0.87142857142857,0.885714285714284,0.899999999999999,
0.914285714285713,0.928571428571427,0.942857142857141,0.957142857142856,
0.97142857142857,0.985714285714284,1.),(0.,2.1),.UNSPECIFIED.);
#229=B_SPLINE_SURFACE_WITH_KNOTS('',5,1,((#19084,#19085),(#19086,#19087),
(#19088,#19089),(#19090,#19091),(#19092,#19093),(#19094,#19095),(#19096,
#19097),(#19098,#19099),(#19100,#19101),(#19102,#19103),(#19104,#19105),
(#19106,#19107),(#19108,#19109),(#19110,#19111),(#19112,#19113),(#19114,
#19115),(#19116,#19117),(#19118,#19119),(#19120,#19121),(#19122,#19123),
(#19124,#19125),(#19126,#19127),(#19128,#19129),(#19130,#19131),(#19132,
#19133),(#19134,#19135),(#19136,#19137),(#19138,#19139),(#19140,#19141),
(#19142,#19143),(#19144,#19145),(#19146,#19147),(#19148,#19149),(#19150,
#19151),(#19152,#19153),(#19154,#19155),(#19156,#19157),(#19158,#19159),
(#19160,#19161),(#19162,#19163),(#19164,#19165),(#19166,#19167),(#19168,
#19169),(#19170,#19171),(#19172,#19173),(#19174,#19175),(#19176,#19177),
(#19178,#19179),(#19180,#19181),(#19182,#19183),(#19184,#19185),(#19186,
#19187),(#19188,#19189),(#19190,#19191),(#19192,#19193),(#19194,#19195),
(#19196,#19197),(#19198,#19199),(#19200,#19201),(#19202,#19203),(#19204,
#19205),(#19206,#19207),(#19208,#19209),(#19210,#19211),(#19212,#19213),
(#19214,#19215),(#19216,#19217),(#19218,#19219),(#19220,#19221),(#19222,
#19223),(#19224,#19225),(#19226,#19227),(#19228,#19229),(#19230,#19231),
(#19232,#19233)),.UNSPECIFIED.,.F.,.F.,.F.,(6,1,1,1,1,1,1,1,1,1,1,1,1,1,
1,1,1,1,1,1,1,1,1,1,1,1,1,1,1,1,1,1,1,1,1,1,1,1,1,1,1,1,1,1,1,1,1,1,1,1,
1,1,1,1,1,1,1,1,1,1,1,1,1,1,1,1,1,1,1,1,6),(2,2),(-1.,-0.985714285714284,
-0.97142857142857,-0.957142857142856,-0.942857142857141,-0.928571428571427,
-0.914285714285713,-0.899999999999999,-0.885714285714284,-0.87142857142857,
-0.857142857142856,-0.842857142857142,-0.828571428571428,-0.814285714285713,
-0.799999999999999,-0.785714285714285,-0.771428571428571,-0.757142857142856,
-0.742857142857142,-0.728571428571428,-0.714285714285714,-0.699999999999999,
-0.685714285714285,-0.671428571428571,-0.657142857142857,-0.642857142857142,
-0.628571428571428,-0.614285714285714,-0.6,-0.585714285714286,-0.571428571428571,
-0.557142857142857,-0.542857142857143,-0.528571428571429,-0.514285714285714,
-0.5,-0.485714285714286,-0.471428571428572,-0.457142857142857,-0.442857142857143,
-0.428571428571429,-0.414285714285714,-0.4,-0.385714285714286,-0.371428571428571,
-0.357142857142857,-0.342857142857143,-0.328571428571429,-0.314285714285714,
-0.3,-0.285714285714286,-0.271428571428571,-0.257142857142857,-0.242857142857143,
-0.228571428571429,-0.214285714285714,-0.2,-0.185714285714286,-0.171428571428571,
-0.157142857142857,-0.142857142857143,-0.128571428571429,-0.114285714285714,
-0.1,-0.0857142857142857,-0.0714285714285714,-0.0571428571428571,-0.0428571428571429,
-0.0285714285714286,-0.0142857142857143,0.),(0.,2.1),.UNSPECIFIED.);
#230=B_SPLINE_SURFACE_WITH_KNOTS('',5,1,((#19237,#19238),(#19239,#19240),
(#19241,#19242),(#19243,#19244),(#19245,#19246),(#19247,#19248),(#19249,
#19250),(#19251,#19252),(#19253,#19254),(#19255,#19256),(#19257,#19258),
(#19259,#19260),(#19261,#19262),(#19263,#19264),(#19265,#19266),(#19267,
#19268),(#19269,#19270),(#19271,#19272),(#19273,#19274),(#19275,#19276),
(#19277,#19278),(#19279,#19280),(#19281,#19282),(#19283,#19284),(#19285,
#19286),(#19287,#19288),(#19289,#19290),(#19291,#19292),(#19293,#19294),
(#19295,#19296),(#19297,#19298),(#19299,#19300),(#19301,#19302),(#19303,
#19304),(#19305,#19306),(#19307,#19308),(#19309,#19310),(#19311,#19312),
(#19313,#19314),(#19315,#19316),(#19317,#19318),(#19319,#19320),(#19321,
#19322),(#19323,#19324),(#19325,#19326),(#19327,#19328),(#19329,#19330),
(#19331,#19332),(#19333,#19334),(#19335,#19336),(#19337,#19338),(#19339,
#19340),(#19341,#19342),(#19343,#19344),(#19345,#19346),(#19347,#19348),
(#19349,#19350),(#19351,#19352),(#19353,#19354),(#19355,#19356),(#19357,
#19358),(#19359,#19360),(#19361,#19362),(#19363,#19364),(#19365,#19366),
(#19367,#19368),(#19369,#19370),(#19371,#19372),(#19373,#19374),(#19375,
#19376),(#19377,#19378),(#19379,#19380),(#19381,#19382),(#19383,#19384),
(#19385,#19386)),.UNSPECIFIED.,.F.,.F.,.F.,(6,1,1,1,1,1,1,1,1,1,1,1,1,1,
1,1,1,1,1,1,1,1,1,1,1,1,1,1,1,1,1,1,1,1,1,1,1,1,1,1,1,1,1,1,1,1,1,1,1,1,
1,1,1,1,1,1,1,1,1,1,1,1,1,1,1,1,1,1,1,1,6),(2,2),(0.,0.0142857142857143,
0.0285714285714286,0.0428571428571429,0.0571428571428571,0.0714285714285714,
0.0857142857142857,0.1,0.114285714285714,0.128571428571429,0.142857142857143,
0.157142857142857,0.171428571428571,0.185714285714286,0.2,0.214285714285714,
0.228571428571429,0.242857142857143,0.257142857142857,0.271428571428571,
0.285714285714286,0.3,0.314285714285714,0.328571428571429,0.342857142857143,
0.357142857142857,0.371428571428571,0.385714285714286,0.4,0.414285714285714,
0.428571428571429,0.442857142857143,0.457142857142857,0.471428571428572,
0.485714285714286,0.5,0.514285714285714,0.528571428571429,0.542857142857143,
0.557142857142857,0.571428571428571,0.585714285714286,0.6,0.614285714285714,
0.628571428571428,0.642857142857142,0.657142857142857,0.671428571428571,
0.685714285714285,0.699999999999999,0.714285714285714,0.728571428571428,
0.742857142857142,0.757142857142856,0.771428571428571,0.785714285714285,
0.799999999999999,0.814285714285713,0.828571428571428,0.842857142857142,
0.857142857142856,0.87142857142857,0.885714285714284,0.899999999999999,
0.914285714285713,0.928571428571427,0.942857142857141,0.957142857142856,
0.97142857142857,0.985714285714284,1.),(0.,2.1),.UNSPECIFIED.);
#231=PLANE('',#4918);
#232=PLANE('',#4922);
#233=PLANE('',#4926);
#234=PLANE('',#4930);
#235=PLANE('',#4934);
#236=PLANE('',#4938);
#237=PLANE('',#4942);
#238=PLANE('',#4946);
#239=PLANE('',#4950);
#240=PLANE('',#4954);
#241=PLANE('',#4958);
#242=PLANE('',#4962);
#243=PLANE('',#4966);
#244=PLANE('',#4970);
#245=PLANE('',#4974);
#246=PLANE('',#4978);
#247=PLANE('',#4982);
#248=PLANE('',#4986);
#249=PLANE('',#4990);
#250=PLANE('',#4994);
#251=PLANE('',#4998);
#252=PLANE('',#5002);
#253=PLANE('',#5006);
#254=PLANE('',#5010);
#255=PLANE('',#5014);
#256=PLANE('',#5018);
#257=PLANE('',#5022);
#258=PLANE('',#5026);
#259=PLANE('',#5030);
#260=PLANE('',#5034);
#261=PLANE('',#5038);
#262=PLANE('',#5042);
#263=PLANE('',#5046);
#264=PLANE('',#5050);
#265=PLANE('',#5054);
#266=PLANE('',#5058);
#267=PLANE('',#5062);
#268=PLANE('',#5066);
#269=PLANE('',#5124);
#270=PLANE('',#5148);
#271=PLANE('',#5192);
#272=PLANE('',#5194);
#325=FACE_OUTER_BOUND('',#601,.T.);
#326=FACE_OUTER_BOUND('',#602,.T.);
#327=FACE_OUTER_BOUND('',#603,.T.);
#328=FACE_OUTER_BOUND('',#604,.T.);
#329=FACE_OUTER_BOUND('',#605,.T.);
#330=FACE_OUTER_BOUND('',#606,.T.);
#331=FACE_OUTER_BOUND('',#607,.T.);
#332=FACE_OUTER_BOUND('',#608,.T.);
#333=FACE_OUTER_BOUND('',#609,.T.);
#334=FACE_OUTER_BOUND('',#610,.T.);
#335=FACE_OUTER_BOUND('',#611,.T.);
#336=FACE_OUTER_BOUND('',#612,.T.);
#337=FACE_OUTER_BOUND('',#613,.T.);
#338=FACE_OUTER_BOUND('',#614,.T.);
#339=FACE_OUTER_BOUND('',#615,.T.);
#340=FACE_OUTER_BOUND('',#616,.T.);
#341=FACE_OUTER_BOUND('',#617,.T.);
#342=FACE_OUTER_BOUND('',#618,.T.);
#343=FACE_OUTER_BOUND('',#619,.T.);
#344=FACE_OUTER_BOUND('',#620,.T.);
#345=FACE_OUTER_BOUND('',#621,.T.);
#346=FACE_OUTER_BOUND('',#622,.T.);
#347=FACE_OUTER_BOUND('',#623,.T.);
#348=FACE_OUTER_BOUND('',#624,.T.);
#349=FACE_OUTER_BOUND('',#625,.T.);
#350=FACE_OUTER_BOUND('',#626,.T.);
#351=FACE_OUTER_BOUND('',#627,.T.);
#352=FACE_OUTER_BOUND('',#628,.T.);
#353=FACE_OUTER_BOUND('',#629,.T.);
#354=FACE_OUTER_BOUND('',#630,.T.);
#355=FACE_OUTER_BOUND('',#631,.T.);
#356=FACE_OUTER_BOUND('',#632,.T.);
#357=FACE_OUTER_BOUND('',#633,.T.);
#358=FACE_OUTER_BOUND('',#634,.T.);
#359=FACE_OUTER_BOUND('',#635,.T.);
#360=FACE_OUTER_BOUND('',#636,.T.);
#361=FACE_OUTER_BOUND('',#637,.T.);
#362=FACE_OUTER_BOUND('',#638,.T.);
#363=FACE_OUTER_BOUND('',#639,.T.);
#364=FACE_OUTER_BOUND('',#640,.T.);
#365=FACE_OUTER_BOUND('',#641,.T.);
#366=FACE_OUTER_BOUND('',#642,.T.);
#367=FACE_OUTER_BOUND('',#643,.T.);
#368=FACE_OUTER_BOUND('',#644,.T.);
#369=FACE_OUTER_BOUND('',#645,.T.);
#370=FACE_OUTER_BOUND('',#646,.T.);
#371=FACE_OUTER_BOUND('',#647,.T.);
#372=FACE_OUTER_BOUND('',#648,.T.);
#373=FACE_OUTER_BOUND('',#649,.T.);
#374=FACE_OUTER_BOUND('',#650,.T.);
#375=FACE_OUTER_BOUND('',#651,.T.);
#376=FACE_OUTER_BOUND('',#652,.T.);
#377=FACE_OUTER_BOUND('',#653,.T.);
#378=FACE_OUTER_BOUND('',#654,.T.);
#379=FACE_OUTER_BOUND('',#655,.T.);
#380=FACE_OUTER_BOUND('',#656,.T.);
#381=FACE_OUTER_BOUND('',#657,.T.);
#382=FACE_OUTER_BOUND('',#658,.T.);
#383=FACE_OUTER_BOUND('',#659,.T.);
#384=FACE_OUTER_BOUND('',#660,.T.);
#385=FACE_OUTER_BOUND('',#661,.T.);
#386=FACE_OUTER_BOUND('',#662,.T.);
#387=FACE_OUTER_BOUND('',#663,.T.);
#388=FACE_OUTER_BOUND('',#664,.T.);
#389=FACE_OUTER_BOUND('',#665,.T.);
#390=FACE_OUTER_BOUND('',#666,.T.);
#391=FACE_OUTER_BOUND('',#667,.T.);
#392=FACE_OUTER_BOUND('',#668,.T.);
#393=FACE_OUTER_BOUND('',#669,.T.);
#394=FACE_OUTER_BOUND('',#670,.T.);
#395=FACE_OUTER_BOUND('',#671,.T.);
#396=FACE_OUTER_BOUND('',#672,.T.);
#397=FACE_OUTER_BOUND('',#673,.T.);
#398=FACE_OUTER_BOUND('',#674,.T.);
#399=FACE_OUTER_BOUND('',#675,.T.);
#400=FACE_OUTER_BOUND('',#676,.T.);
#401=FACE_OUTER_BOUND('',#677,.T.);
#402=FACE_OUTER_BOUND('',#678,.T.);
#403=FACE_OUTER_BOUND('',#679,.T.);
#404=FACE_OUTER_BOUND('',#680,.T.);
#405=FACE_OUTER_BOUND('',#681,.T.);
#406=FACE_OUTER_BOUND('',#682,.T.);
#407=FACE_OUTER_BOUND('',#683,.T.);
#408=FACE_OUTER_BOUND('',#684,.T.);
#409=FACE_OUTER_BOUND('',#685,.T.);
#410=FACE_OUTER_BOUND('',#686,.T.);
#411=FACE_OUTER_BOUND('',#687,.T.);
#412=FACE_OUTER_BOUND('',#688,.T.);
#413=FACE_OUTER_BOUND('',#689,.T.);
#414=FACE_OUTER_BOUND('',#690,.T.);
#415=FACE_OUTER_BOUND('',#691,.T.);
#416=FACE_OUTER_BOUND('',#692,.T.);
#417=FACE_OUTER_BOUND('',#693,.T.);
#418=FACE_OUTER_BOUND('',#694,.T.);
#419=FACE_OUTER_BOUND('',#695,.T.);
#420=FACE_OUTER_BOUND('',#696,.T.);
#421=FACE_OUTER_BOUND('',#697,.T.);
#422=FACE_OUTER_BOUND('',#698,.T.);
#423=FACE_OUTER_BOUND('',#699,.T.);
#424=FACE_OUTER_BOUND('',#700,.T.);
#425=FACE_OUTER_BOUND('',#701,.T.);
#426=FACE_OUTER_BOUND('',#702,.T.);
#427=FACE_OUTER_BOUND('',#703,.T.);
#428=FACE_OUTER_BOUND('',#704,.T.);
#429=FACE_OUTER_BOUND('',#705,.T.);
#430=FACE_OUTER_BOUND('',#706,.T.);
#431=FACE_OUTER_BOUND('',#707,.T.);
#432=FACE_OUTER_BOUND('',#708,.T.);
#433=FACE_OUTER_BOUND('',#709,.T.);
#434=FACE_OUTER_BOUND('',#710,.T.);
#435=FACE_OUTER_BOUND('',#711,.T.);
#436=FACE_OUTER_BOUND('',#712,.T.);
#437=FACE_OUTER_BOUND('',#713,.T.);
#438=FACE_OUTER_BOUND('',#714,.T.);
#439=FACE_OUTER_BOUND('',#715,.T.);
#440=FACE_OUTER_BOUND('',#716,.T.);
#441=FACE_OUTER_BOUND('',#717,.T.);
#442=FACE_OUTER_BOUND('',#718,.T.);
#443=FACE_OUTER_BOUND('',#719,.T.);
#444=FACE_OUTER_BOUND('',#720,.T.);
#445=FACE_OUTER_BOUND('',#721,.T.);
#446=FACE_OUTER_BOUND('',#722,.T.);
#447=FACE_OUTER_BOUND('',#723,.T.);
#448=FACE_OUTER_BOUND('',#724,.T.);
#449=FACE_OUTER_BOUND('',#725,.T.);
#450=FACE_OUTER_BOUND('',#726,.T.);
#451=FACE_OUTER_BOUND('',#727,.T.);
#452=FACE_OUTER_BOUND('',#728,.T.);
#453=FACE_OUTER_BOUND('',#729,.T.);
#454=FACE_OUTER_BOUND('',#730,.T.);
#455=FACE_OUTER_BOUND('',#731,.T.);
#456=FACE_OUTER_BOUND('',#732,.T.);
#457=FACE_OUTER_BOUND('',#733,.T.);
#458=FACE_OUTER_BOUND('',#734,.T.);
#459=FACE_OUTER_BOUND('',#735,.T.);
#460=FACE_OUTER_BOUND('',#737,.T.);
#461=FACE_OUTER_BOUND('',#739,.T.);
#462=FACE_OUTER_BOUND('',#740,.T.);
#463=FACE_OUTER_BOUND('',#741,.T.);
#464=FACE_OUTER_BOUND('',#742,.T.);
#465=FACE_OUTER_BOUND('',#743,.T.);
#466=FACE_OUTER_BOUND('',#744,.T.);
#467=FACE_OUTER_BOUND('',#745,.T.);
#468=FACE_OUTER_BOUND('',#746,.T.);
#469=FACE_OUTER_BOUND('',#747,.T.);
#470=FACE_OUTER_BOUND('',#748,.T.);
#471=FACE_OUTER_BOUND('',#749,.T.);
#472=FACE_OUTER_BOUND('',#750,.T.);
#473=FACE_OUTER_BOUND('',#751,.T.);
#474=FACE_OUTER_BOUND('',#752,.T.);
#475=FACE_OUTER_BOUND('',#753,.T.);
#476=FACE_OUTER_BOUND('',#754,.T.);
#477=FACE_OUTER_BOUND('',#755,.T.);
#478=FACE_OUTER_BOUND('',#756,.T.);
#479=FACE_OUTER_BOUND('',#757,.T.);
#480=FACE_OUTER_BOUND('',#758,.T.);
#481=FACE_OUTER_BOUND('',#759,.T.);
#482=FACE_OUTER_BOUND('',#760,.T.);
#483=FACE_OUTER_BOUND('',#761,.T.);
#484=FACE_OUTER_BOUND('',#762,.T.);
#485=FACE_OUTER_BOUND('',#763,.T.);
#486=FACE_OUTER_BOUND('',#764,.T.);
#487=FACE_OUTER_BOUND('',#765,.T.);
#601=EDGE_LOOP('',(#3027,#3028,#3029,#3030));
#602=EDGE_LOOP('',(#3031,#3032,#3033,#3034));
#603=EDGE_LOOP('',(#3035,#3036,#3037,#3038));
#604=EDGE_LOOP('',(#3039,#3040,#3041,#3042));
#605=EDGE_LOOP('',(#3043,#3044,#3045,#3046));
#606=EDGE_LOOP('',(#3047,#3048,#3049,#3050));
#607=EDGE_LOOP('',(#3051,#3052,#3053,#3054));
#608=EDGE_LOOP('',(#3055,#3056,#3057,#3058));
#609=EDGE_LOOP('',(#3059,#3060,#3061,#3062));
#610=EDGE_LOOP('',(#3063,#3064,#3065,#3066));
#611=EDGE_LOOP('',(#3067,#3068,#3069,#3070));
#612=EDGE_LOOP('',(#3071,#3072,#3073,#3074));
#613=EDGE_LOOP('',(#3075,#3076,#3077,#3078));
#614=EDGE_LOOP('',(#3079,#3080,#3081,#3082));
#615=EDGE_LOOP('',(#3083,#3084,#3085,#3086));
#616=EDGE_LOOP('',(#3087,#3088,#3089,#3090));
#617=EDGE_LOOP('',(#3091,#3092,#3093,#3094));
#618=EDGE_LOOP('',(#3095,#3096,#3097,#3098));
#619=EDGE_LOOP('',(#3099,#3100,#3101,#3102));
#620=EDGE_LOOP('',(#3103,#3104,#3105,#3106));
#621=EDGE_LOOP('',(#3107,#3108,#3109,#3110));
#622=EDGE_LOOP('',(#3111,#3112,#3113,#3114));
#623=EDGE_LOOP('',(#3115,#3116,#3117,#3118));
#624=EDGE_LOOP('',(#3119,#3120,#3121,#3122));
#625=EDGE_LOOP('',(#3123,#3124,#3125,#3126));
#626=EDGE_LOOP('',(#3127,#3128,#3129,#3130));
#627=EDGE_LOOP('',(#3131,#3132,#3133,#3134));
#628=EDGE_LOOP('',(#3135,#3136,#3137,#3138));
#629=EDGE_LOOP('',(#3139,#3140,#3141,#3142));
#630=EDGE_LOOP('',(#3143,#3144,#3145,#3146));
#631=EDGE_LOOP('',(#3147,#3148,#3149,#3150));
#632=EDGE_LOOP('',(#3151,#3152,#3153,#3154));
#633=EDGE_LOOP('',(#3155,#3156,#3157,#3158));
#634=EDGE_LOOP('',(#3159,#3160,#3161,#3162));
#635=EDGE_LOOP('',(#3163,#3164,#3165,#3166));
#636=EDGE_LOOP('',(#3167,#3168,#3169,#3170));
#637=EDGE_LOOP('',(#3171,#3172,#3173,#3174));
#638=EDGE_LOOP('',(#3175,#3176,#3177,#3178));
#639=EDGE_LOOP('',(#3179,#3180,#3181,#3182));
#640=EDGE_LOOP('',(#3183,#3184,#3185,#3186));
#641=EDGE_LOOP('',(#3187,#3188,#3189,#3190));
#642=EDGE_LOOP('',(#3191,#3192,#3193,#3194));
#643=EDGE_LOOP('',(#3195,#3196,#3197,#3198));
#644=EDGE_LOOP('',(#3199,#3200,#3201,#3202));
#645=EDGE_LOOP('',(#3203,#3204,#3205,#3206));
#646=EDGE_LOOP('',(#3207,#3208,#3209,#3210));
#647=EDGE_LOOP('',(#3211,#3212,#3213,#3214));
#648=EDGE_LOOP('',(#3215,#3216,#3217,#3218));
#649=EDGE_LOOP('',(#3219,#3220,#3221,#3222));
#650=EDGE_LOOP('',(#3223,#3224,#3225,#3226));
#651=EDGE_LOOP('',(#3227,#3228,#3229,#3230));
#652=EDGE_LOOP('',(#3231,#3232,#3233,#3234));
#653=EDGE_LOOP('',(#3235,#3236,#3237,#3238));
#654=EDGE_LOOP('',(#3239,#3240,#3241,#3242));
#655=EDGE_LOOP('',(#3243,#3244,#3245,#3246));
#656=EDGE_LOOP('',(#3247,#3248,#3249,#3250));
#657=EDGE_LOOP('',(#3251,#3252,#3253,#3254));
#658=EDGE_LOOP('',(#3255,#3256,#3257,#3258));
#659=EDGE_LOOP('',(#3259,#3260,#3261,#3262));
#660=EDGE_LOOP('',(#3263,#3264,#3265,#3266));
#661=EDGE_LOOP('',(#3267,#3268,#3269,#3270));
#662=EDGE_LOOP('',(#3271,#3272,#3273,#3274));
#663=EDGE_LOOP('',(#3275,#3276,#3277,#3278));
#664=EDGE_LOOP('',(#3279,#3280,#3281,#3282));
#665=EDGE_LOOP('',(#3283,#3284,#3285,#3286));
#666=EDGE_LOOP('',(#3287,#3288,#3289,#3290));
#667=EDGE_LOOP('',(#3291,#3292,#3293,#3294));
#668=EDGE_LOOP('',(#3295,#3296,#3297,#3298));
#669=EDGE_LOOP('',(#3299,#3300,#3301,#3302));
#670=EDGE_LOOP('',(#3303,#3304,#3305,#3306));
#671=EDGE_LOOP('',(#3307,#3308,#3309,#3310));
#672=EDGE_LOOP('',(#3311,#3312,#3313,#3314));
#673=EDGE_LOOP('',(#3315,#3316,#3317,#3318));
#674=EDGE_LOOP('',(#3319,#3320,#3321,#3322));
#675=EDGE_LOOP('',(#3323,#3324,#3325,#3326));
#676=EDGE_LOOP('',(#3327,#3328,#3329,#3330));
#677=EDGE_LOOP('',(#3331,#3332,#3333,#3334));
#678=EDGE_LOOP('',(#3335,#3336,#3337,#3338));
#679=EDGE_LOOP('',(#3339,#3340,#3341,#3342));
#680=EDGE_LOOP('',(#3343,#3344,#3345,#3346));
#681=EDGE_LOOP('',(#3347,#3348,#3349,#3350));
#682=EDGE_LOOP('',(#3351,#3352,#3353,#3354));
#683=EDGE_LOOP('',(#3355,#3356,#3357,#3358));
#684=EDGE_LOOP('',(#3359,#3360,#3361,#3362));
#685=EDGE_LOOP('',(#3363,#3364,#3365,#3366));
#686=EDGE_LOOP('',(#3367,#3368,#3369,#3370));
#687=EDGE_LOOP('',(#3371,#3372,#3373,#3374));
#688=EDGE_LOOP('',(#3375,#3376,#3377,#3378));
#689=EDGE_LOOP('',(#3379,#3380,#3381,#3382));
#690=EDGE_LOOP('',(#3383,#3384,#3385,#3386));
#691=EDGE_LOOP('',(#3387,#3388,#3389,#3390));
#692=EDGE_LOOP('',(#3391,#3392,#3393,#3394));
#693=EDGE_LOOP('',(#3395,#3396,#3397,#3398));
#694=EDGE_LOOP('',(#3399,#3400,#3401,#3402));
#695=EDGE_LOOP('',(#3403,#3404,#3405,#3406));
#696=EDGE_LOOP('',(#3407,#3408,#3409,#3410));
#697=EDGE_LOOP('',(#3411,#3412,#3413,#3414));
#698=EDGE_LOOP('',(#3415,#3416,#3417,#3418));
#699=EDGE_LOOP('',(#3419,#3420,#3421,#3422));
#700=EDGE_LOOP('',(#3423,#3424,#3425,#3426));
#701=EDGE_LOOP('',(#3427,#3428,#3429,#3430));
#702=EDGE_LOOP('',(#3431,#3432,#3433,#3434));
#703=EDGE_LOOP('',(#3435,#3436,#3437,#3438));
#704=EDGE_LOOP('',(#3439,#3440,#3441,#3442));
#705=EDGE_LOOP('',(#3443,#3444,#3445,#3446));
#706=EDGE_LOOP('',(#3447,#3448,#3449,#3450));
#707=EDGE_LOOP('',(#3451,#3452,#3453,#3454));
#708=EDGE_LOOP('',(#3455,#3456,#3457,#3458));
#709=EDGE_LOOP('',(#3459,#3460,#3461,#3462));
#710=EDGE_LOOP('',(#3463,#3464,#3465,#3466));
#711=EDGE_LOOP('',(#3467,#3468,#3469,#3470));
#712=EDGE_LOOP('',(#3471,#3472,#3473,#3474));
#713=EDGE_LOOP('',(#3475,#3476,#3477,#3478));
#714=EDGE_LOOP('',(#3479,#3480,#3481,#3482));
#715=EDGE_LOOP('',(#3483,#3484,#3485,#3486));
#716=EDGE_LOOP('',(#3487,#3488,#3489,#3490));
#717=EDGE_LOOP('',(#3491,#3492,#3493,#3494));
#718=EDGE_LOOP('',(#3495,#3496,#3497,#3498));
#719=EDGE_LOOP('',(#3499,#3500,#3501,#3502));
#720=EDGE_LOOP('',(#3503,#3504,#3505,#3506));
#721=EDGE_LOOP('',(#3507,#3508,#3509,#3510));
#722=EDGE_LOOP('',(#3511,#3512,#3513,#3514));
#723=EDGE_LOOP('',(#3515,#3516,#3517,#3518));
#724=EDGE_LOOP('',(#3519,#3520,#3521,#3522));
#725=EDGE_LOOP('',(#3523,#3524,#3525,#3526));
#726=EDGE_LOOP('',(#3527,#3528,#3529,#3530));
#727=EDGE_LOOP('',(#3531,#3532,#3533,#3534));
#728=EDGE_LOOP('',(#3535,#3536,#3537,#3538));
#729=EDGE_LOOP('',(#3539,#3540,#3541,#3542));
#730=EDGE_LOOP('',(#3543,#3544,#3545,#3546));
#731=EDGE_LOOP('',(#3547,#3548,#3549,#3550));
#732=EDGE_LOOP('',(#3551,#3552,#3553,#3554));
#733=EDGE_LOOP('',(#3555,#3556,#3557,#3558));
#734=EDGE_LOOP('',(#3559,#3560,#3561,#3562));
#735=EDGE_LOOP('',(#3563,#3564,#3565,#3566,#3567,#3568,#3569,#3570,#3571,
#3572,#3573,#3574,#3575,#3576,#3577,#3578,#3579,#3580,#3581,#3582,#3583,
#3584,#3585,#3586,#3587,#3588,#3589,#3590,#3591,#3592,#3593,#3594,#3595,
#3596,#3597,#3598,#3599,#3600,#3601,#3602,#3603,#3604,#3605,#3606,#3607,
#3608,#3609,#3610,#3611,#3612,#3613,#3614,#3615,#3616,#3617,#3618,#3619,
#3620,#3621,#3622,#3623,#3624,#3625,#3626,#3627,#3628,#3629,#3630,#3631,
#3632,#3633,#3634,#3635,#3636,#3637,#3638,#3639,#3640,#3641,#3642,#3643,
#3644,#3645,#3646,#3647,#3648,#3649,#3650,#3651,#3652,#3653,#3654,#3655,
#3656,#3657,#3658,#3659,#3660,#3661,#3662,#3663,#3664,#3665,#3666,#3667,
#3668,#3669,#3670,#3671,#3672,#3673,#3674,#3675,#3676,#3677,#3678,#3679,
#3680,#3681,#3682,#3683,#3684,#3685,#3686,#3687,#3688,#3689,#3690,#3691,
#3692,#3693,#3694,#3695,#3696,#3697,#3698,#3699,#3700,#3701,#3702,#3703,
#3704,#3705,#3706,#3707,#3708,#3709,#3710,#3711,#3712,#3713,#3714,#3715,
#3716,#3717,#3718,#3719,#3720,#3721,#3722));
#736=EDGE_LOOP('',(#3723));
#737=EDGE_LOOP('',(#3724,#3725,#3726,#3727,#3728,#3729,#3730,#3731,#3732,
#3733,#3734,#3735,#3736,#3737,#3738,#3739,#3740,#3741,#3742,#3743,#3744,
#3745,#3746,#3747,#3748,#3749,#3750,#3751,#3752,#3753,#3754,#3755,#3756,
#3757,#3758,#3759,#3760,#3761,#3762,#3763,#3764,#3765,#3766,#3767,#3768,
#3769,#3770,#3771,#3772,#3773,#3774,#3775,#3776,#3777,#3778,#3779,#3780,
#3781,#3782,#3783,#3784,#3785,#3786,#3787,#3788,#3789,#3790,#3791,#3792,
#3793,#3794,#3795,#3796,#3797,#3798,#3799,#3800,#3801,#3802,#3803,#3804,
#3805,#3806,#3807,#3808,#3809,#3810,#3811,#3812,#3813,#3814,#3815,#3816,
#3817,#3818,#3819,#3820,#3821,#3822,#3823,#3824,#3825,#3826,#3827,#3828,
#3829,#3830,#3831,#3832,#3833,#3834,#3835,#3836,#3837,#3838,#3839,#3840,
#3841,#3842,#3843,#3844,#3845,#3846,#3847,#3848,#3849,#3850,#3851,#3852,
#3853,#3854,#3855,#3856,#3857,#3858,#3859,#3860,#3861,#3862,#3863,#3864,
#3865,#3866,#3867,#3868,#3869,#3870,#3871,#3872,#3873,#3874,#3875,#3876,
#3877,#3878,#3879,#3880,#3881,#3882,#3883));
#738=EDGE_LOOP('',(#3884));
#739=EDGE_LOOP('',(#3885,#3886,#3887,#3888));
#740=EDGE_LOOP('',(#3889,#3890,#3891,#3892));
#741=EDGE_LOOP('',(#3893,#3894,#3895,#3896));
#742=EDGE_LOOP('',(#3897,#3898,#3899,#3900));
#743=EDGE_LOOP('',(#3901,#3902,#3903,#3904));
#744=EDGE_LOOP('',(#3905,#3906,#3907,#3908));
#745=EDGE_LOOP('',(#3909,#3910,#3911,#3912));
#746=EDGE_LOOP('',(#3913,#3914,#3915,#3916));
#747=EDGE_LOOP('',(#3917,#3918,#3919,#3920));
#748=EDGE_LOOP('',(#3921,#3922,#3923,#3924));
#749=EDGE_LOOP('',(#3925,#3926,#3927,#3928));
#750=EDGE_LOOP('',(#3929,#3930,#3931,#3932));
#751=EDGE_LOOP('',(#3933,#3934,#3935,#3936));
#752=EDGE_LOOP('',(#3937,#3938,#3939,#3940));
#753=EDGE_LOOP('',(#3941,#3942,#3943,#3944));
#754=EDGE_LOOP('',(#3945,#3946,#3947,#3948));
#755=EDGE_LOOP('',(#3949,#3950,#3951,#3952));
#756=EDGE_LOOP('',(#3953,#3954,#3955,#3956));
#757=EDGE_LOOP('',(#3957,#3958,#3959,#3960));
#758=EDGE_LOOP('',(#3961,#3962,#3963,#3964));
#759=EDGE_LOOP('',(#3965,#3966,#3967,#3968));
#760=EDGE_LOOP('',(#3969,#3970,#3971,#3972));
#761=EDGE_LOOP('',(#3973,#3974,#3975,#3976));
#762=EDGE_LOOP('',(#3977,#3978,#3979,#3980));
#763=EDGE_LOOP('',(#3981,#3982,#3983,#3984));
#764=EDGE_LOOP('',(#3985,#3986,#3987,#3988));
#765=EDGE_LOOP('',(#3989,#3990,#3991,#3992));
#897=LINE('',#6823,#1253);
#898=LINE('',#6830,#1254);
#899=LINE('',#6833,#1255);
#900=LINE('',#6836,#1256);
#901=LINE('',#6838,#1257);
#902=LINE('',#6839,#1258);
#903=LINE('',#6845,#1259);
#904=LINE('',#6848,#1260);
#905=LINE('',#6851,#1261);
#906=LINE('',#6853,#1262);
#907=LINE('',#6854,#1263);
#908=LINE('',#6860,#1264);
#909=LINE('',#6863,#1265);
#910=LINE('',#6866,#1266);
#911=LINE('',#6868,#1267);
#912=LINE('',#6869,#1268);
#913=LINE('',#6875,#1269);
#914=LINE('',#6878,#1270);
#915=LINE('',#6881,#1271);
#916=LINE('',#6883,#1272);
#917=LINE('',#6884,#1273);
#918=LINE('',#6890,#1274);
#919=LINE('',#6893,#1275);
#920=LINE('',#6896,#1276);
#921=LINE('',#6898,#1277);
#922=LINE('',#6899,#1278);
#923=LINE('',#6905,#1279);
#924=LINE('',#6908,#1280);
#925=LINE('',#6911,#1281);
#926=LINE('',#6913,#1282);
#927=LINE('',#6914,#1283);
#928=LINE('',#6920,#1284);
#929=LINE('',#6923,#1285);
#930=LINE('',#6926,#1286);
#931=LINE('',#6928,#1287);
#932=LINE('',#6929,#1288);
#933=LINE('',#6935,#1289);
#934=LINE('',#6938,#1290);
#935=LINE('',#6941,#1291);
#936=LINE('',#6943,#1292);
#937=LINE('',#6944,#1293);
#938=LINE('',#6950,#1294);
#939=LINE('',#6953,#1295);
#940=LINE('',#6956,#1296);
#941=LINE('',#6958,#1297);
#942=LINE('',#6959,#1298);
#943=LINE('',#6965,#1299);
#944=LINE('',#6968,#1300);
#945=LINE('',#6971,#1301);
#946=LINE('',#6973,#1302);
#947=LINE('',#6974,#1303);
#948=LINE('',#6980,#1304);
#949=LINE('',#6983,#1305);
#950=LINE('',#6986,#1306);
#951=LINE('',#6988,#1307);
#952=LINE('',#6989,#1308);
#953=LINE('',#6995,#1309);
#954=LINE('',#6998,#1310);
#955=LINE('',#7001,#1311);
#956=LINE('',#7003,#1312);
#957=LINE('',#7004,#1313);
#958=LINE('',#7010,#1314);
#959=LINE('',#7013,#1315);
#960=LINE('',#7016,#1316);
#961=LINE('',#7018,#1317);
#962=LINE('',#7019,#1318);
#963=LINE('',#7025,#1319);
#964=LINE('',#7028,#1320);
#965=LINE('',#7031,#1321);
#966=LINE('',#7033,#1322);
#967=LINE('',#7034,#1323);
#968=LINE('',#7040,#1324);
#969=LINE('',#7043,#1325);
#970=LINE('',#7046,#1326);
#971=LINE('',#7048,#1327);
#972=LINE('',#7049,#1328);
#973=LINE('',#7055,#1329);
#974=LINE('',#7058,#1330);
#975=LINE('',#7061,#1331);
#976=LINE('',#7063,#1332);
#977=LINE('',#7064,#1333);
#978=LINE('',#7070,#1334);
#979=LINE('',#7073,#1335);
#980=LINE('',#7076,#1336);
#981=LINE('',#7078,#1337);
#982=LINE('',#7079,#1338);
#983=LINE('',#7085,#1339);
#984=LINE('',#7088,#1340);
#985=LINE('',#7091,#1341);
#986=LINE('',#7093,#1342);
#987=LINE('',#7094,#1343);
#988=LINE('',#7100,#1344);
#989=LINE('',#7103,#1345);
#990=LINE('',#7106,#1346);
#991=LINE('',#7108,#1347);
#992=LINE('',#7109,#1348);
#993=LINE('',#7115,#1349);
#994=LINE('',#7118,#1350);
#995=LINE('',#7121,#1351);
#996=LINE('',#7123,#1352);
#997=LINE('',#7124,#1353);
#998=LINE('',#7130,#1354);
#999=LINE('',#7133,#1355);
#1000=LINE('',#7136,#1356);
#1001=LINE('',#7138,#1357);
#1002=LINE('',#7139,#1358);
#1003=LINE('',#7145,#1359);
#1004=LINE('',#7148,#1360);
#1005=LINE('',#7151,#1361);
#1006=LINE('',#7153,#1362);
#1007=LINE('',#7154,#1363);
#1008=LINE('',#7160,#1364);
#1009=LINE('',#7163,#1365);
#1010=LINE('',#7166,#1366);
#1011=LINE('',#7168,#1367);
#1012=LINE('',#7169,#1368);
#1013=LINE('',#7175,#1369);
#1014=LINE('',#7178,#1370);
#1015=LINE('',#7181,#1371);
#1016=LINE('',#7183,#1372);
#1017=LINE('',#7184,#1373);
#1018=LINE('',#7190,#1374);
#1019=LINE('',#7193,#1375);
#1020=LINE('',#7196,#1376);
#1021=LINE('',#7198,#1377);
#1022=LINE('',#7199,#1378);
#1023=LINE('',#7205,#1379);
#1024=LINE('',#7208,#1380);
#1025=LINE('',#7211,#1381);
#1026=LINE('',#7213,#1382);
#1027=LINE('',#7214,#1383);
#1028=LINE('',#7220,#1384);
#1029=LINE('',#7223,#1385);
#1030=LINE('',#7226,#1386);
#1031=LINE('',#7228,#1387);
#1032=LINE('',#7229,#1388);
#1033=LINE('',#7235,#1389);
#1034=LINE('',#7238,#1390);
#1035=LINE('',#7241,#1391);
#1036=LINE('',#7243,#1392);
#1037=LINE('',#7244,#1393);
#1038=LINE('',#7250,#1394);
#1039=LINE('',#7253,#1395);
#1040=LINE('',#7256,#1396);
#1041=LINE('',#7258,#1397);
#1042=LINE('',#7259,#1398);
#1043=LINE('',#7265,#1399);
#1044=LINE('',#7268,#1400);
#1045=LINE('',#7271,#1401);
#1046=LINE('',#7273,#1402);
#1047=LINE('',#7274,#1403);
#1048=LINE('',#7280,#1404);
#1049=LINE('',#7283,#1405);
#1050=LINE('',#7286,#1406);
#1051=LINE('',#7288,#1407);
#1052=LINE('',#7289,#1408);
#1053=LINE('',#7295,#1409);
#1054=LINE('',#7298,#1410);
#1055=LINE('',#7301,#1411);
#1056=LINE('',#7303,#1412);
#1057=LINE('',#7304,#1413);
#1058=LINE('',#7310,#1414);
#1059=LINE('',#7313,#1415);
#1060=LINE('',#7316,#1416);
#1061=LINE('',#7318,#1417);
#1062=LINE('',#7319,#1418);
#1063=LINE('',#7325,#1419);
#1064=LINE('',#7328,#1420);
#1065=LINE('',#7331,#1421);
#1066=LINE('',#7333,#1422);
#1067=LINE('',#7334,#1423);
#1068=LINE('',#7340,#1424);
#1069=LINE('',#7343,#1425);
#1070=LINE('',#7346,#1426);
#1071=LINE('',#7348,#1427);
#1072=LINE('',#7349,#1428);
#1073=LINE('',#7355,#1429);
#1074=LINE('',#7358,#1430);
#1075=LINE('',#7361,#1431);
#1076=LINE('',#7363,#1432);
#1077=LINE('',#7364,#1433);
#1078=LINE('',#7370,#1434);
#1079=LINE('',#7373,#1435);
#1080=LINE('',#7376,#1436);
#1081=LINE('',#7378,#1437);
#1082=LINE('',#7379,#1438);
#1083=LINE('',#7385,#1439);
#1084=LINE('',#7388,#1440);
#1085=LINE('',#7391,#1441);
#1086=LINE('',#7393,#1442);
#1087=LINE('',#7394,#1443);
#1088=LINE('',#7688,#1444);
#1089=LINE('',#7694,#1445);
#1090=LINE('',#8282,#1446);
#1091=LINE('',#8288,#1447);
#1092=LINE('',#8882,#1448);
#1093=LINE('',#8888,#1449);
#1094=LINE('',#9476,#1450);
#1095=LINE('',#9482,#1451);
#1096=LINE('',#10070,#1452);
#1097=LINE('',#10076,#1453);
#1098=LINE('',#10664,#1454);
#1099=LINE('',#10670,#1455);
#1100=LINE('',#11258,#1456);
#1101=LINE('',#11264,#1457);
#1102=LINE('',#11852,#1458);
#1103=LINE('',#11858,#1459);
#1104=LINE('',#12446,#1460);
#1105=LINE('',#12452,#1461);
#1106=LINE('',#13040,#1462);
#1107=LINE('',#13046,#1463);
#1108=LINE('',#13634,#1464);
#1109=LINE('',#13640,#1465);
#1110=LINE('',#14228,#1466);
#1111=LINE('',#14234,#1467);
#1112=LINE('',#14822,#1468);
#1113=LINE('',#14828,#1469);
#1114=LINE('',#15416,#1470);
#1115=LINE('',#15422,#1471);
#1116=LINE('',#16010,#1472);
#1117=LINE('',#16016,#1473);
#1118=LINE('',#16604,#1474);
#1119=LINE('',#16610,#1475);
#1120=LINE('',#17213,#1476);
#1121=LINE('',#17219,#1477);
#1122=LINE('',#17807,#1478);
#1123=LINE('',#17813,#1479);
#1124=LINE('',#18401,#1480);
#1125=LINE('',#18407,#1481);
#1126=LINE('',#18725,#1482);
#1127=LINE('',#18879,#1483);
#1128=LINE('',#18890,#1484);
#1129=LINE('',#19033,#1485);
#1130=LINE('',#19056,#1486);
#1131=LINE('',#19076,#1487);
#1132=LINE('',#19078,#1488);
#1133=LINE('',#19080,#1489);
#1134=LINE('',#19081,#1490);
#1135=LINE('',#19083,#1491);
#1136=LINE('',#19234,#1492);
#1137=LINE('',#19236,#1493);
#1253=VECTOR('',#5435,5.);
#1254=VECTOR('',#5442,10.);
#1255=VECTOR('',#5445,10.);
#1256=VECTOR('',#5448,10.);
#1257=VECTOR('',#5449,10.);
#1258=VECTOR('',#5450,10.);
#1259=VECTOR('',#5455,10.);
#1260=VECTOR('',#5458,10.);
#1261=VECTOR('',#5461,10.);
#1262=VECTOR('',#5462,10.);
#1263=VECTOR('',#5463,10.);
#1264=VECTOR('',#5468,10.);
#1265=VECTOR('',#5471,10.);
#1266=VECTOR('',#5474,10.);
#1267=VECTOR('',#5475,10.);
#1268=VECTOR('',#5476,10.);
#1269=VECTOR('',#5481,10.);
#1270=VECTOR('',#5484,10.);
#1271=VECTOR('',#5487,10.);
#1272=VECTOR('',#5488,10.);
#1273=VECTOR('',#5489,10.);
#1274=VECTOR('',#5494,10.);
#1275=VECTOR('',#5497,10.);
#1276=VECTOR('',#5500,10.);
#1277=VECTOR('',#5501,10.);
#1278=VECTOR('',#5502,10.);
#1279=VECTOR('',#5507,10.);
#1280=VECTOR('',#5510,10.);
#1281=VECTOR('',#5513,10.);
#1282=VECTOR('',#5514,10.);
#1283=VECTOR('',#5515,10.);
#1284=VECTOR('',#5520,10.);
#1285=VECTOR('',#5523,10.);
#1286=VECTOR('',#5526,10.);
#1287=VECTOR('',#5527,10.);
#1288=VECTOR('',#5528,10.);
#1289=VECTOR('',#5533,10.);
#1290=VECTOR('',#5536,10.);
#1291=VECTOR('',#5539,10.);
#1292=VECTOR('',#5540,10.);
#1293=VECTOR('',#5541,10.);
#1294=VECTOR('',#5546,10.);
#1295=VECTOR('',#5549,10.);
#1296=VECTOR('',#5552,10.);
#1297=VECTOR('',#5553,10.);
#1298=VECTOR('',#5554,10.);
#1299=VECTOR('',#5559,10.);
#1300=VECTOR('',#5562,10.);
#1301=VECTOR('',#5565,10.);
#1302=VECTOR('',#5566,10.);
#1303=VECTOR('',#5567,10.);
#1304=VECTOR('',#5572,10.);
#1305=VECTOR('',#5575,10.);
#1306=VECTOR('',#5578,10.);
#1307=VECTOR('',#5579,10.);
#1308=VECTOR('',#5580,10.);
#1309=VECTOR('',#5585,10.);
#1310=VECTOR('',#5588,10.);
#1311=VECTOR('',#5591,10.);
#1312=VECTOR('',#5592,10.);
#1313=VECTOR('',#5593,10.);
#1314=VECTOR('',#5598,10.);
#1315=VECTOR('',#5601,10.);
#1316=VECTOR('',#5604,10.);
#1317=VECTOR('',#5605,10.);
#1318=VECTOR('',#5606,10.);
#1319=VECTOR('',#5611,10.);
#1320=VECTOR('',#5614,10.);
#1321=VECTOR('',#5617,10.);
#1322=VECTOR('',#5618,10.);
#1323=VECTOR('',#5619,10.);
#1324=VECTOR('',#5624,10.);
#1325=VECTOR('',#5627,10.);
#1326=VECTOR('',#5630,10.);
#1327=VECTOR('',#5631,10.);
#1328=VECTOR('',#5632,10.);
#1329=VECTOR('',#5637,10.);
#1330=VECTOR('',#5640,10.);
#1331=VECTOR('',#5643,10.);
#1332=VECTOR('',#5644,10.);
#1333=VECTOR('',#5645,10.);
#1334=VECTOR('',#5650,10.);
#1335=VECTOR('',#5653,10.);
#1336=VECTOR('',#5656,10.);
#1337=VECTOR('',#5657,10.);
#1338=VECTOR('',#5658,10.);
#1339=VECTOR('',#5663,10.);
#1340=VECTOR('',#5666,10.);
#1341=VECTOR('',#5669,10.);
#1342=VECTOR('',#5670,10.);
#1343=VECTOR('',#5671,10.);
#1344=VECTOR('',#5676,10.);
#1345=VECTOR('',#5679,10.);
#1346=VECTOR('',#5682,10.);
#1347=VECTOR('',#5683,10.);
#1348=VECTOR('',#5684,10.);
#1349=VECTOR('',#5689,10.);
#1350=VECTOR('',#5692,10.);
#1351=VECTOR('',#5695,10.);
#1352=VECTOR('',#5696,10.);
#1353=VECTOR('',#5697,10.);
#1354=VECTOR('',#5702,10.);
#1355=VECTOR('',#5705,10.);
#1356=VECTOR('',#5708,10.);
#1357=VECTOR('',#5709,10.);
#1358=VECTOR('',#5710,10.);
#1359=VECTOR('',#5715,10.);
#1360=VECTOR('',#5718,10.);
#1361=VECTOR('',#5721,10.);
#1362=VECTOR('',#5722,10.);
#1363=VECTOR('',#5723,10.);
#1364=VECTOR('',#5728,10.);
#1365=VECTOR('',#5731,10.);
#1366=VECTOR('',#5734,10.);
#1367=VECTOR('',#5735,10.);
#1368=VECTOR('',#5736,10.);
#1369=VECTOR('',#5741,10.);
#1370=VECTOR('',#5744,10.);
#1371=VECTOR('',#5747,10.);
#1372=VECTOR('',#5748,10.);
#1373=VECTOR('',#5749,10.);
#1374=VECTOR('',#5754,10.);
#1375=VECTOR('',#5757,10.);
#1376=VECTOR('',#5760,10.);
#1377=VECTOR('',#5761,10.);
#1378=VECTOR('',#5762,10.);
#1379=VECTOR('',#5767,10.);
#1380=VECTOR('',#5770,10.);
#1381=VECTOR('',#5773,10.);
#1382=VECTOR('',#5774,10.);
#1383=VECTOR('',#5775,10.);
#1384=VECTOR('',#5780,10.);
#1385=VECTOR('',#5783,10.);
#1386=VECTOR('',#5786,10.);
#1387=VECTOR('',#5787,10.);
#1388=VECTOR('',#5788,10.);
#1389=VECTOR('',#5793,10.);
#1390=VECTOR('',#5796,10.);
#1391=VECTOR('',#5799,10.);
#1392=VECTOR('',#5800,10.);
#1393=VECTOR('',#5801,10.);
#1394=VECTOR('',#5806,10.);
#1395=VECTOR('',#5809,10.);
#1396=VECTOR('',#5812,10.);
#1397=VECTOR('',#5813,10.);
#1398=VECTOR('',#5814,10.);
#1399=VECTOR('',#5819,10.);
#1400=VECTOR('',#5822,10.);
#1401=VECTOR('',#5825,10.);
#1402=VECTOR('',#5826,10.);
#1403=VECTOR('',#5827,10.);
#1404=VECTOR('',#5832,10.);
#1405=VECTOR('',#5835,10.);
#1406=VECTOR('',#5838,10.);
#1407=VECTOR('',#5839,10.);
#1408=VECTOR('',#5840,10.);
#1409=VECTOR('',#5845,10.);
#1410=VECTOR('',#5848,10.);
#1411=VECTOR('',#5851,10.);
#1412=VECTOR('',#5852,10.);
#1413=VECTOR('',#5853,10.);
#1414=VECTOR('',#5858,10.);
#1415=VECTOR('',#5861,10.);
#1416=VECTOR('',#5864,10.);
#1417=VECTOR('',#5865,10.);
#1418=VECTOR('',#5866,10.);
#1419=VECTOR('',#5871,10.);
#1420=VECTOR('',#5874,10.);
#1421=VECTOR('',#5877,10.);
#1422=VECTOR('',#5878,10.);
#1423=VECTOR('',#5879,10.);
#1424=VECTOR('',#5884,10.);
#1425=VECTOR('',#5887,10.);
#1426=VECTOR('',#5890,10.);
#1427=VECTOR('',#5891,10.);
#1428=VECTOR('',#5892,10.);
#1429=VECTOR('',#5897,10.);
#1430=VECTOR('',#5900,10.);
#1431=VECTOR('',#5903,10.);
#1432=VECTOR('',#5904,10.);
#1433=VECTOR('',#5905,10.);
#1434=VECTOR('',#5910,10.);
#1435=VECTOR('',#5913,10.);
#1436=VECTOR('',#5916,10.);
#1437=VECTOR('',#5917,10.);
#1438=VECTOR('',#5918,10.);
#1439=VECTOR('',#5923,10.);
#1440=VECTOR('',#5926,10.);
#1441=VECTOR('',#5929,10.);
#1442=VECTOR('',#5930,10.);
#1443=VECTOR('',#5931,10.);
#1444=VECTOR('',#5932,10.);
#1445=VECTOR('',#5939,10.);
#1446=VECTOR('',#5940,10.);
#1447=VECTOR('',#5947,10.);
#1448=VECTOR('',#5948,10.);
#1449=VECTOR('',#5955,10.);
#1450=VECTOR('',#5956,10.);
#1451=VECTOR('',#5963,10.);
#1452=VECTOR('',#5964,10.);
#1453=VECTOR('',#5971,10.);
#1454=VECTOR('',#5972,10.);
#1455=VECTOR('',#5979,10.);
#1456=VECTOR('',#5980,10.);
#1457=VECTOR('',#5987,10.);
#1458=VECTOR('',#5988,10.);
#1459=VECTOR('',#5995,10.);
#1460=VECTOR('',#5996,10.);
#1461=VECTOR('',#6003,10.);
#1462=VECTOR('',#6004,10.);
#1463=VECTOR('',#6011,10.);
#1464=VECTOR('',#6012,10.);
#1465=VECTOR('',#6019,10.);
#1466=VECTOR('',#6020,10.);
#1467=VECTOR('',#6027,10.);
#1468=VECTOR('',#6028,10.);
#1469=VECTOR('',#6035,10.);
#1470=VECTOR('',#6036,10.);
#1471=VECTOR('',#6043,10.);
#1472=VECTOR('',#6044,10.);
#1473=VECTOR('',#6051,10.);
#1474=VECTOR('',#6052,10.);
#1475=VECTOR('',#6059,10.);
#1476=VECTOR('',#6060,10.);
#1477=VECTOR('',#6067,10.);
#1478=VECTOR('',#6068,10.);
#1479=VECTOR('',#6075,10.);
#1480=VECTOR('',#6076,10.);
#1481=VECTOR('',#6083,10.);
#1482=VECTOR('',#6124,10.);
#1483=VECTOR('',#6127,10.);
#1484=VECTOR('',#6140,10.);
#1485=VECTOR('',#6143,10.);
#1486=VECTOR('',#6186,10.);
#1487=VECTOR('',#6225,10.);
#1488=VECTOR('',#6228,10.);
#1489=VECTOR('',#6231,10.);
#1490=VECTOR('',#6232,10.);
#1491=VECTOR('',#6235,10.);
#1492=VECTOR('',#6236,10.);
#1493=VECTOR('',#6239,10.);
#1609=CIRCLE('',#4913,5.);
#1610=CIRCLE('',#4914,5.);
#1611=CIRCLE('',#4916,1.);
#1612=CIRCLE('',#4917,1.);
#1613=CIRCLE('',#4920,1.);
#1614=CIRCLE('',#4921,1.);
#1615=CIRCLE('',#4924,1.);
#1616=CIRCLE('',#4925,1.);
#1617=CIRCLE('',#4928,1.);
#1618=CIRCLE('',#4929,1.);
#1619=CIRCLE('',#4932,1.);
#1620=CIRCLE('',#4933,1.);
#1621=CIRCLE('',#4936,1.);
#1622=CIRCLE('',#4937,1.);
#1623=CIRCLE('',#4940,1.);
#1624=CIRCLE('',#4941,1.);
#1625=CIRCLE('',#4944,1.);
#1626=CIRCLE('',#4945,1.);
#1627=CIRCLE('',#4948,1.);
#1628=CIRCLE('',#4949,1.);
#1629=CIRCLE('',#4952,1.);
#1630=CIRCLE('',#4953,1.);
#1631=CIRCLE('',#4956,1.);
#1632=CIRCLE('',#4957,1.);
#1633=CIRCLE('',#4960,1.);
#1634=CIRCLE('',#4961,1.);
#1635=CIRCLE('',#4964,1.);
#1636=CIRCLE('',#4965,1.);
#1637=CIRCLE('',#4968,1.);
#1638=CIRCLE('',#4969,1.);
#1639=CIRCLE('',#4972,1.);
#1640=CIRCLE('',#4973,1.);
#1641=CIRCLE('',#4976,1.);
#1642=CIRCLE('',#4977,1.);
#1643=CIRCLE('',#4980,1.);
#1644=CIRCLE('',#4981,1.);
#1645=CIRCLE('',#4984,1.);
#1646=CIRCLE('',#4985,1.);
#1647=CIRCLE('',#4988,1.);
#1648=CIRCLE('',#4989,1.);
#1649=CIRCLE('',#4992,1.);
#1650=CIRCLE('',#4993,1.);
#1651=CIRCLE('',#4996,1.);
#1652=CIRCLE('',#4997,1.);
#1653=CIRCLE('',#5000,1.);
#1654=CIRCLE('',#5001,1.);
#1655=CIRCLE('',#5004,1.);
#1656=CIRCLE('',#5005,1.);
#1657=CIRCLE('',#5008,1.);
#1658=CIRCLE('',#5009,1.);
#1659=CIRCLE('',#5012,1.);
#1660=CIRCLE('',#5013,1.);
#1661=CIRCLE('',#5016,1.);
#1662=CIRCLE('',#5017,1.);
#1663=CIRCLE('',#5020,1.);
#1664=CIRCLE('',#5021,1.);
#1665=CIRCLE('',#5024,1.);
#1666=CIRCLE('',#5025,1.);
#1667=CIRCLE('',#5028,1.);
#1668=CIRCLE('',#5029,1.);
#1669=CIRCLE('',#5032,1.);
#1670=CIRCLE('',#5033,1.);
#1671=CIRCLE('',#5036,1.);
#1672=CIRCLE('',#5037,1.);
#1673=CIRCLE('',#5040,1.);
#1674=CIRCLE('',#5041,1.);
#1675=CIRCLE('',#5044,1.);
#1676=CIRCLE('',#5045,1.);
#1677=CIRCLE('',#5048,1.);
#1678=CIRCLE('',#5049,1.);
#1679=CIRCLE('',#5052,1.);
#1680=CIRCLE('',#5053,1.);
#1681=CIRCLE('',#5056,1.);
#1682=CIRCLE('',#5057,1.);
#1683=CIRCLE('',#5060,1.);
#1684=CIRCLE('',#5061,1.);
#1685=CIRCLE('',#5064,1.);
#1686=CIRCLE('',#5065,1.);
#1687=CIRCLE('',#5068,21.9999999999943);
#1688=CIRCLE('',#5069,21.9999999999943);
#1689=CIRCLE('',#5071,21.9999999999943);
#1690=CIRCLE('',#5072,21.9999999999943);
#1691=CIRCLE('',#5074,21.9999999999943);
#1692=CIRCLE('',#5075,21.9999999999943);
#1693=CIRCLE('',#5077,21.9999999999943);
#1694=CIRCLE('',#5078,21.9999999999943);
#1695=CIRCLE('',#5080,21.9999999999943);
#1696=CIRCLE('',#5081,21.9999999999943);
#1697=CIRCLE('',#5083,21.9999999999943);
#1698=CIRCLE('',#5084,21.9999999999943);
#1699=CIRCLE('',#5086,21.9999999999943);
#1700=CIRCLE('',#5087,21.9999999999943);
#1701=CIRCLE('',#5089,21.9999999999943);
#1702=CIRCLE('',#5090,21.9999999999943);
#1703=CIRCLE('',#5092,21.9999999999943);
#1704=CIRCLE('',#5093,21.9999999999943);
#1705=CIRCLE('',#5095,21.9999999999943);
#1706=CIRCLE('',#5096,21.9999999999943);
#1707=CIRCLE('',#5098,21.9999999999943);
#1708=CIRCLE('',#5099,21.9999999999943);
#1709=CIRCLE('',#5101,21.9999999999943);
#1710=CIRCLE('',#5102,21.9999999999943);
#1711=CIRCLE('',#5104,21.9999999999943);
#1712=CIRCLE('',#5105,21.9999999999943);
#1713=CIRCLE('',#5107,21.9999999999943);
#1714=CIRCLE('',#5108,21.9999999999943);
#1715=CIRCLE('',#5110,21.9999999999943);
#1716=CIRCLE('',#5111,21.9999999999943);
#1717=CIRCLE('',#5113,21.9999999999943);
#1718=CIRCLE('',#5114,21.9999999999943);
#1719=CIRCLE('',#5116,21.9999999999943);
#1720=CIRCLE('',#5117,21.9999999999943);
#1721=CIRCLE('',#5119,21.9999999999943);
#1722=CIRCLE('',#5120,21.9999999999943);
#1723=CIRCLE('',#5122,21.9999999999943);
#1724=CIRCLE('',#5123,21.9999999999943);
#1725=CIRCLE('',#5125,17.686);
#1726=CIRCLE('',#5126,17.686);
#1727=CIRCLE('',#5127,17.686);
#1728=CIRCLE('',#5128,17.686);
#1729=CIRCLE('',#5129,17.686);
#1730=CIRCLE('',#5130,17.686);
#1731=CIRCLE('',#5131,17.686);
#1732=CIRCLE('',#5132,17.686);
#1733=CIRCLE('',#5133,17.686);
#1734=CIRCLE('',#5134,17.686);
#1735=CIRCLE('',#5135,17.686);
#1736=CIRCLE('',#5136,17.686);
#1737=CIRCLE('',#5137,17.686);
#1738=CIRCLE('',#5138,17.686);
#1739=CIRCLE('',#5139,17.686);
#1740=CIRCLE('',#5140,17.686);
#1741=CIRCLE('',#5141,17.686);
#1742=CIRCLE('',#5142,17.686);
#1743=CIRCLE('',#5143,1.);
#1744=CIRCLE('',#5144,21.9999999999943);
#1745=CIRCLE('',#5145,1.);
#1746=CIRCLE('',#5146,17.686);
#1747=CIRCLE('',#5147,17.686);
#1748=CIRCLE('',#5149,17.686);
#1749=CIRCLE('',#5150,1.);
#1750=CIRCLE('',#5151,21.9999999999943);
#1751=CIRCLE('',#5152,1.);
#1752=CIRCLE('',#5153,17.686);
#1753=CIRCLE('',#5154,17.686);
#1754=CIRCLE('',#5155,17.686);
#1755=CIRCLE('',#5156,17.686);
#1756=CIRCLE('',#5157,17.686);
#1757=CIRCLE('',#5158,17.686);
#1758=CIRCLE('',#5159,17.686);
#1759=CIRCLE('',#5160,17.686);
#1760=CIRCLE('',#5161,17.686);
#1761=CIRCLE('',#5162,17.686);
#1762=CIRCLE('',#5163,17.686);
#1763=CIRCLE('',#5164,17.686);
#1764=CIRCLE('',#5165,17.686);
#1765=CIRCLE('',#5166,17.686);
#1766=CIRCLE('',#5167,17.686);
#1767=CIRCLE('',#5168,17.686);
#1768=CIRCLE('',#5169,17.686);
#1769=CIRCLE('',#5170,17.686);
#1770=CIRCLE('',#5171,17.686);
#1875=VERTEX_POINT('',#6820);
#1876=VERTEX_POINT('',#6822);
#1877=VERTEX_POINT('',#6826);
#1878=VERTEX_POINT('',#6827);
#1879=VERTEX_POINT('',#6829);
#1880=VERTEX_POINT('',#6831);
#1881=VERTEX_POINT('',#6835);
#1882=VERTEX_POINT('',#6837);
#1883=VERTEX_POINT('',#6841);
#1884=VERTEX_POINT('',#6842);
#1885=VERTEX_POINT('',#6844);
#1886=VERTEX_POINT('',#6846);
#1887=VERTEX_POINT('',#6850);
#1888=VERTEX_POINT('',#6852);
#1889=VERTEX_POINT('',#6856);
#1890=VERTEX_POINT('',#6857);
#1891=VERTEX_POINT('',#6859);
#1892=VERTEX_POINT('',#6861);
#1893=VERTEX_POINT('',#6865);
#1894=VERTEX_POINT('',#6867);
#1895=VERTEX_POINT('',#6871);
#1896=VERTEX_POINT('',#6872);
#1897=VERTEX_POINT('',#6874);
#1898=VERTEX_POINT('',#6876);
#1899=VERTEX_POINT('',#6880);
#1900=VERTEX_POINT('',#6882);
#1901=VERTEX_POINT('',#6886);
#1902=VERTEX_POINT('',#6887);
#1903=VERTEX_POINT('',#6889);
#1904=VERTEX_POINT('',#6891);
#1905=VERTEX_POINT('',#6895);
#1906=VERTEX_POINT('',#6897);
#1907=VERTEX_POINT('',#6901);
#1908=VERTEX_POINT('',#6902);
#1909=VERTEX_POINT('',#6904);
#1910=VERTEX_POINT('',#6906);
#1911=VERTEX_POINT('',#6910);
#1912=VERTEX_POINT('',#6912);
#1913=VERTEX_POINT('',#6916);
#1914=VERTEX_POINT('',#6917);
#1915=VERTEX_POINT('',#6919);
#1916=VERTEX_POINT('',#6921);
#1917=VERTEX_POINT('',#6925);
#1918=VERTEX_POINT('',#6927);
#1919=VERTEX_POINT('',#6931);
#1920=VERTEX_POINT('',#6932);
#1921=VERTEX_POINT('',#6934);
#1922=VERTEX_POINT('',#6936);
#1923=VERTEX_POINT('',#6940);
#1924=VERTEX_POINT('',#6942);
#1925=VERTEX_POINT('',#6946);
#1926=VERTEX_POINT('',#6947);
#1927=VERTEX_POINT('',#6949);
#1928=VERTEX_POINT('',#6951);
#1929=VERTEX_POINT('',#6955);
#1930=VERTEX_POINT('',#6957);
#1931=VERTEX_POINT('',#6961);
#1932=VERTEX_POINT('',#6962);
#1933=VERTEX_POINT('',#6964);
#1934=VERTEX_POINT('',#6966);
#1935=VERTEX_POINT('',#6970);
#1936=VERTEX_POINT('',#6972);
#1937=VERTEX_POINT('',#6976);
#1938=VERTEX_POINT('',#6977);
#1939=VERTEX_POINT('',#6979);
#1940=VERTEX_POINT('',#6981);
#1941=VERTEX_POINT('',#6985);
#1942=VERTEX_POINT('',#6987);
#1943=VERTEX_POINT('',#6991);
#1944=VERTEX_POINT('',#6992);
#1945=VERTEX_POINT('',#6994);
#1946=VERTEX_POINT('',#6996);
#1947=VERTEX_POINT('',#7000);
#1948=VERTEX_POINT('',#7002);
#1949=VERTEX_POINT('',#7006);
#1950=VERTEX_POINT('',#7007);
#1951=VERTEX_POINT('',#7009);
#1952=VERTEX_POINT('',#7011);
#1953=VERTEX_POINT('',#7015);
#1954=VERTEX_POINT('',#7017);
#1955=VERTEX_POINT('',#7021);
#1956=VERTEX_POINT('',#7022);
#1957=VERTEX_POINT('',#7024);
#1958=VERTEX_POINT('',#7026);
#1959=VERTEX_POINT('',#7030);
#1960=VERTEX_POINT('',#7032);
#1961=VERTEX_POINT('',#7036);
#1962=VERTEX_POINT('',#7037);
#1963=VERTEX_POINT('',#7039);
#1964=VERTEX_POINT('',#7041);
#1965=VERTEX_POINT('',#7045);
#1966=VERTEX_POINT('',#7047);
#1967=VERTEX_POINT('',#7051);
#1968=VERTEX_POINT('',#7052);
#1969=VERTEX_POINT('',#7054);
#1970=VERTEX_POINT('',#7056);
#1971=VERTEX_POINT('',#7060);
#1972=VERTEX_POINT('',#7062);
#1973=VERTEX_POINT('',#7066);
#1974=VERTEX_POINT('',#7067);
#1975=VERTEX_POINT('',#7069);
#1976=VERTEX_POINT('',#7071);
#1977=VERTEX_POINT('',#7075);
#1978=VERTEX_POINT('',#7077);
#1979=VERTEX_POINT('',#7081);
#1980=VERTEX_POINT('',#7082);
#1981=VERTEX_POINT('',#7084);
#1982=VERTEX_POINT('',#7086);
#1983=VERTEX_POINT('',#7090);
#1984=VERTEX_POINT('',#7092);
#1985=VERTEX_POINT('',#7096);
#1986=VERTEX_POINT('',#7097);
#1987=VERTEX_POINT('',#7099);
#1988=VERTEX_POINT('',#7101);
#1989=VERTEX_POINT('',#7105);
#1990=VERTEX_POINT('',#7107);
#1991=VERTEX_POINT('',#7111);
#1992=VERTEX_POINT('',#7112);
#1993=VERTEX_POINT('',#7114);
#1994=VERTEX_POINT('',#7116);
#1995=VERTEX_POINT('',#7120);
#1996=VERTEX_POINT('',#7122);
#1997=VERTEX_POINT('',#7126);
#1998=VERTEX_POINT('',#7127);
#1999=VERTEX_POINT('',#7129);
#2000=VERTEX_POINT('',#7131);
#2001=VERTEX_POINT('',#7135);
#2002=VERTEX_POINT('',#7137);
#2003=VERTEX_POINT('',#7141);
#2004=VERTEX_POINT('',#7142);
#2005=VERTEX_POINT('',#7144);
#2006=VERTEX_POINT('',#7146);
#2007=VERTEX_POINT('',#7150);
#2008=VERTEX_POINT('',#7152);
#2009=VERTEX_POINT('',#7156);
#2010=VERTEX_POINT('',#7157);
#2011=VERTEX_POINT('',#7159);
#2012=VERTEX_POINT('',#7161);
#2013=VERTEX_POINT('',#7165);
#2014=VERTEX_POINT('',#7167);
#2015=VERTEX_POINT('',#7171);
#2016=VERTEX_POINT('',#7172);
#2017=VERTEX_POINT('',#7174);
#2018=VERTEX_POINT('',#7176);
#2019=VERTEX_POINT('',#7180);
#2020=VERTEX_POINT('',#7182);
#2021=VERTEX_POINT('',#7186);
#2022=VERTEX_POINT('',#7187);
#2023=VERTEX_POINT('',#7189);
#2024=VERTEX_POINT('',#7191);
#2025=VERTEX_POINT('',#7195);
#2026=VERTEX_POINT('',#7197);
#2027=VERTEX_POINT('',#7201);
#2028=VERTEX_POINT('',#7202);
#2029=VERTEX_POINT('',#7204);
#2030=VERTEX_POINT('',#7206);
#2031=VERTEX_POINT('',#7210);
#2032=VERTEX_POINT('',#7212);
#2033=VERTEX_POINT('',#7216);
#2034=VERTEX_POINT('',#7217);
#2035=VERTEX_POINT('',#7219);
#2036=VERTEX_POINT('',#7221);
#2037=VERTEX_POINT('',#7225);
#2038=VERTEX_POINT('',#7227);
#2039=VERTEX_POINT('',#7231);
#2040=VERTEX_POINT('',#7232);
#2041=VERTEX_POINT('',#7234);
#2042=VERTEX_POINT('',#7236);
#2043=VERTEX_POINT('',#7240);
#2044=VERTEX_POINT('',#7242);
#2045=VERTEX_POINT('',#7246);
#2046=VERTEX_POINT('',#7247);
#2047=VERTEX_POINT('',#7249);
#2048=VERTEX_POINT('',#7251);
#2049=VERTEX_POINT('',#7255);
#2050=VERTEX_POINT('',#7257);
#2051=VERTEX_POINT('',#7261);
#2052=VERTEX_POINT('',#7262);
#2053=VERTEX_POINT('',#7264);
#2054=VERTEX_POINT('',#7266);
#2055=VERTEX_POINT('',#7270);
#2056=VERTEX_POINT('',#7272);
#2057=VERTEX_POINT('',#7276);
#2058=VERTEX_POINT('',#7277);
#2059=VERTEX_POINT('',#7279);
#2060=VERTEX_POINT('',#7281);
#2061=VERTEX_POINT('',#7285);
#2062=VERTEX_POINT('',#7287);
#2063=VERTEX_POINT('',#7291);
#2064=VERTEX_POINT('',#7292);
#2065=VERTEX_POINT('',#7294);
#2066=VERTEX_POINT('',#7296);
#2067=VERTEX_POINT('',#7300);
#2068=VERTEX_POINT('',#7302);
#2069=VERTEX_POINT('',#7306);
#2070=VERTEX_POINT('',#7307);
#2071=VERTEX_POINT('',#7309);
#2072=VERTEX_POINT('',#7311);
#2073=VERTEX_POINT('',#7315);
#2074=VERTEX_POINT('',#7317);
#2075=VERTEX_POINT('',#7321);
#2076=VERTEX_POINT('',#7322);
#2077=VERTEX_POINT('',#7324);
#2078=VERTEX_POINT('',#7326);
#2079=VERTEX_POINT('',#7330);
#2080=VERTEX_POINT('',#7332);
#2081=VERTEX_POINT('',#7336);
#2082=VERTEX_POINT('',#7337);
#2083=VERTEX_POINT('',#7339);
#2084=VERTEX_POINT('',#7341);
#2085=VERTEX_POINT('',#7345);
#2086=VERTEX_POINT('',#7347);
#2087=VERTEX_POINT('',#7351);
#2088=VERTEX_POINT('',#7352);
#2089=VERTEX_POINT('',#7354);
#2090=VERTEX_POINT('',#7356);
#2091=VERTEX_POINT('',#7360);
#2092=VERTEX_POINT('',#7362);
#2093=VERTEX_POINT('',#7366);
#2094=VERTEX_POINT('',#7367);
#2095=VERTEX_POINT('',#7369);
#2096=VERTEX_POINT('',#7371);
#2097=VERTEX_POINT('',#7375);
#2098=VERTEX_POINT('',#7377);
#2099=VERTEX_POINT('',#7381);
#2100=VERTEX_POINT('',#7382);
#2101=VERTEX_POINT('',#7384);
#2102=VERTEX_POINT('',#7386);
#2103=VERTEX_POINT('',#7390);
#2104=VERTEX_POINT('',#7392);
#2105=VERTEX_POINT('',#7545);
#2106=VERTEX_POINT('',#7620);
#2107=VERTEX_POINT('',#7690);
#2108=VERTEX_POINT('',#7692);
#2109=VERTEX_POINT('',#8139);
#2110=VERTEX_POINT('',#8214);
#2111=VERTEX_POINT('',#8284);
#2112=VERTEX_POINT('',#8286);
#2113=VERTEX_POINT('',#8739);
#2114=VERTEX_POINT('',#8814);
#2115=VERTEX_POINT('',#8884);
#2116=VERTEX_POINT('',#8886);
#2117=VERTEX_POINT('',#9333);
#2118=VERTEX_POINT('',#9408);
#2119=VERTEX_POINT('',#9478);
#2120=VERTEX_POINT('',#9480);
#2121=VERTEX_POINT('',#9927);
#2122=VERTEX_POINT('',#10002);
#2123=VERTEX_POINT('',#10072);
#2124=VERTEX_POINT('',#10074);
#2125=VERTEX_POINT('',#10521);
#2126=VERTEX_POINT('',#10596);
#2127=VERTEX_POINT('',#10666);
#2128=VERTEX_POINT('',#10668);
#2129=VERTEX_POINT('',#11115);
#2130=VERTEX_POINT('',#11190);
#2131=VERTEX_POINT('',#11260);
#2132=VERTEX_POINT('',#11262);
#2133=VERTEX_POINT('',#11709);
#2134=VERTEX_POINT('',#11784);
#2135=VERTEX_POINT('',#11854);
#2136=VERTEX_POINT('',#11856);
#2137=VERTEX_POINT('',#12303);
#2138=VERTEX_POINT('',#12378);
#2139=VERTEX_POINT('',#12448);
#2140=VERTEX_POINT('',#12450);
#2141=VERTEX_POINT('',#12897);
#2142=VERTEX_POINT('',#12972);
#2143=VERTEX_POINT('',#13042);
#2144=VERTEX_POINT('',#13044);
#2145=VERTEX_POINT('',#13491);
#2146=VERTEX_POINT('',#13566);
#2147=VERTEX_POINT('',#13636);
#2148=VERTEX_POINT('',#13638);
#2149=VERTEX_POINT('',#14085);
#2150=VERTEX_POINT('',#14160);
#2151=VERTEX_POINT('',#14230);
#2152=VERTEX_POINT('',#14232);
#2153=VERTEX_POINT('',#14679);
#2154=VERTEX_POINT('',#14754);
#2155=VERTEX_POINT('',#14824);
#2156=VERTEX_POINT('',#14826);
#2157=VERTEX_POINT('',#15273);
#2158=VERTEX_POINT('',#15348);
#2159=VERTEX_POINT('',#15418);
#2160=VERTEX_POINT('',#15420);
#2161=VERTEX_POINT('',#15867);
#2162=VERTEX_POINT('',#15942);
#2163=VERTEX_POINT('',#16012);
#2164=VERTEX_POINT('',#16014);
#2165=VERTEX_POINT('',#16461);
#2166=VERTEX_POINT('',#16536);
#2167=VERTEX_POINT('',#16606);
#2168=VERTEX_POINT('',#16608);
#2169=VERTEX_POINT('',#17055);
#2170=VERTEX_POINT('',#17130);
#2171=VERTEX_POINT('',#17215);
#2172=VERTEX_POINT('',#17217);
#2173=VERTEX_POINT('',#17664);
#2174=VERTEX_POINT('',#17739);
#2175=VERTEX_POINT('',#17809);
#2176=VERTEX_POINT('',#17811);
#2177=VERTEX_POINT('',#18258);
#2178=VERTEX_POINT('',#18333);
#2179=VERTEX_POINT('',#18403);
#2180=VERTEX_POINT('',#18405);
#2181=VERTEX_POINT('',#18720);
#2182=VERTEX_POINT('',#18722);
#2183=VERTEX_POINT('',#18724);
#2184=VERTEX_POINT('',#18726);
#2185=VERTEX_POINT('',#18801);
#2186=VERTEX_POINT('',#18803);
#2187=VERTEX_POINT('',#18878);
#2188=VERTEX_POINT('',#18880);
#2189=VERTEX_POINT('',#18885);
#2190=VERTEX_POINT('',#18887);
#2191=VERTEX_POINT('',#18889);
#2192=VERTEX_POINT('',#18891);
#2193=VERTEX_POINT('',#18962);
#2194=VERTEX_POINT('',#18964);
#2195=VERTEX_POINT('',#19032);
#2196=VERTEX_POINT('',#19034);
#2325=EDGE_CURVE('',#1875,#1875,#1609,.T.);
#2326=EDGE_CURVE('',#1875,#1876,#897,.T.);
#2327=EDGE_CURVE('',#1876,#1876,#1610,.T.);
#2328=EDGE_CURVE('',#1877,#1878,#1611,.F.);
#2329=EDGE_CURVE('',#1878,#1879,#898,.T.);
#2330=EDGE_CURVE('',#1879,#1880,#1612,.T.);
#2331=EDGE_CURVE('',#1880,#1877,#899,.T.);
#2332=EDGE_CURVE('',#1881,#1878,#900,.T.);
#2333=EDGE_CURVE('',#1882,#1881,#901,.T.);
#2334=EDGE_CURVE('',#1879,#1882,#902,.T.);
#2335=EDGE_CURVE('',#1883,#1884,#1613,.T.);
#2336=EDGE_CURVE('',#1884,#1885,#903,.T.);
#2337=EDGE_CURVE('',#1885,#1886,#1614,.F.);
#2338=EDGE_CURVE('',#1886,#1883,#904,.T.);
#2339=EDGE_CURVE('',#1884,#1887,#905,.T.);
#2340=EDGE_CURVE('',#1887,#1888,#906,.T.);
#2341=EDGE_CURVE('',#1885,#1888,#907,.T.);
#2342=EDGE_CURVE('',#1889,#1890,#1615,.F.);
#2343=EDGE_CURVE('',#1890,#1891,#908,.T.);
#2344=EDGE_CURVE('',#1891,#1892,#1616,.T.);
#2345=EDGE_CURVE('',#1892,#1889,#909,.T.);
#2346=EDGE_CURVE('',#1893,#1890,#910,.T.);
#2347=EDGE_CURVE('',#1894,#1893,#911,.T.);
#2348=EDGE_CURVE('',#1891,#1894,#912,.T.);
#2349=EDGE_CURVE('',#1895,#1896,#1617,.T.);
#2350=EDGE_CURVE('',#1896,#1897,#913,.T.);
#2351=EDGE_CURVE('',#1897,#1898,#1618,.F.);
#2352=EDGE_CURVE('',#1898,#1895,#914,.T.);
#2353=EDGE_CURVE('',#1896,#1899,#915,.T.);
#2354=EDGE_CURVE('',#1899,#1900,#916,.T.);
#2355=EDGE_CURVE('',#1897,#1900,#917,.T.);
#2356=EDGE_CURVE('',#1901,#1902,#1619,.F.);
#2357=EDGE_CURVE('',#1902,#1903,#918,.T.);
#2358=EDGE_CURVE('',#1903,#1904,#1620,.T.);
#2359=EDGE_CURVE('',#1904,#1901,#919,.T.);
#2360=EDGE_CURVE('',#1905,#1902,#920,.T.);
#2361=EDGE_CURVE('',#1906,#1905,#921,.T.);
#2362=EDGE_CURVE('',#1903,#1906,#922,.T.);
#2363=EDGE_CURVE('',#1907,#1908,#1621,.T.);
#2364=EDGE_CURVE('',#1908,#1909,#923,.T.);
#2365=EDGE_CURVE('',#1909,#1910,#1622,.F.);
#2366=EDGE_CURVE('',#1910,#1907,#924,.T.);
#2367=EDGE_CURVE('',#1908,#1911,#925,.T.);
#2368=EDGE_CURVE('',#1911,#1912,#926,.T.);
#2369=EDGE_CURVE('',#1909,#1912,#927,.T.);
#2370=EDGE_CURVE('',#1913,#1914,#1623,.F.);
#2371=EDGE_CURVE('',#1914,#1915,#928,.T.);
#2372=EDGE_CURVE('',#1915,#1916,#1624,.T.);
#2373=EDGE_CURVE('',#1916,#1913,#929,.T.);
#2374=EDGE_CURVE('',#1917,#1914,#930,.T.);
#2375=EDGE_CURVE('',#1918,#1917,#931,.T.);
#2376=EDGE_CURVE('',#1915,#1918,#932,.T.);
#2377=EDGE_CURVE('',#1919,#1920,#1625,.T.);
#2378=EDGE_CURVE('',#1920,#1921,#933,.T.);
#2379=EDGE_CURVE('',#1921,#1922,#1626,.F.);
#2380=EDGE_CURVE('',#1922,#1919,#934,.T.);
#2381=EDGE_CURVE('',#1920,#1923,#935,.T.);
#2382=EDGE_CURVE('',#1923,#1924,#936,.T.);
#2383=EDGE_CURVE('',#1921,#1924,#937,.T.);
#2384=EDGE_CURVE('',#1925,#1926,#1627,.F.);
#2385=EDGE_CURVE('',#1926,#1927,#938,.T.);
#2386=EDGE_CURVE('',#1927,#1928,#1628,.T.);
#2387=EDGE_CURVE('',#1928,#1925,#939,.T.);
#2388=EDGE_CURVE('',#1929,#1926,#940,.T.);
#2389=EDGE_CURVE('',#1930,#1929,#941,.T.);
#2390=EDGE_CURVE('',#1927,#1930,#942,.T.);
#2391=EDGE_CURVE('',#1931,#1932,#1629,.T.);
#2392=EDGE_CURVE('',#1932,#1933,#943,.T.);
#2393=EDGE_CURVE('',#1933,#1934,#1630,.F.);
#2394=EDGE_CURVE('',#1934,#1931,#944,.T.);
#2395=EDGE_CURVE('',#1932,#1935,#945,.T.);
#2396=EDGE_CURVE('',#1935,#1936,#946,.T.);
#2397=EDGE_CURVE('',#1933,#1936,#947,.T.);
#2398=EDGE_CURVE('',#1937,#1938,#1631,.F.);
#2399=EDGE_CURVE('',#1938,#1939,#948,.T.);
#2400=EDGE_CURVE('',#1939,#1940,#1632,.T.);
#2401=EDGE_CURVE('',#1940,#1937,#949,.T.);
#2402=EDGE_CURVE('',#1941,#1938,#950,.T.);
#2403=EDGE_CURVE('',#1942,#1941,#951,.T.);
#2404=EDGE_CURVE('',#1939,#1942,#952,.T.);
#2405=EDGE_CURVE('',#1943,#1944,#1633,.T.);
#2406=EDGE_CURVE('',#1944,#1945,#953,.T.);
#2407=EDGE_CURVE('',#1945,#1946,#1634,.F.);
#2408=EDGE_CURVE('',#1946,#1943,#954,.T.);
#2409=EDGE_CURVE('',#1944,#1947,#955,.T.);
#2410=EDGE_CURVE('',#1947,#1948,#956,.T.);
#2411=EDGE_CURVE('',#1945,#1948,#957,.T.);
#2412=EDGE_CURVE('',#1949,#1950,#1635,.F.);
#2413=EDGE_CURVE('',#1950,#1951,#958,.T.);
#2414=EDGE_CURVE('',#1951,#1952,#1636,.T.);
#2415=EDGE_CURVE('',#1952,#1949,#959,.T.);
#2416=EDGE_CURVE('',#1953,#1950,#960,.T.);
#2417=EDGE_CURVE('',#1954,#1953,#961,.T.);
#2418=EDGE_CURVE('',#1951,#1954,#962,.T.);
#2419=EDGE_CURVE('',#1955,#1956,#1637,.T.);
#2420=EDGE_CURVE('',#1956,#1957,#963,.T.);
#2421=EDGE_CURVE('',#1957,#1958,#1638,.F.);
#2422=EDGE_CURVE('',#1958,#1955,#964,.T.);
#2423=EDGE_CURVE('',#1956,#1959,#965,.T.);
#2424=EDGE_CURVE('',#1959,#1960,#966,.T.);
#2425=EDGE_CURVE('',#1957,#1960,#967,.T.);
#2426=EDGE_CURVE('',#1961,#1962,#1639,.F.);
#2427=EDGE_CURVE('',#1962,#1963,#968,.T.);
#2428=EDGE_CURVE('',#1963,#1964,#1640,.T.);
#2429=EDGE_CURVE('',#1964,#1961,#969,.T.);
#2430=EDGE_CURVE('',#1965,#1962,#970,.T.);
#2431=EDGE_CURVE('',#1966,#1965,#971,.T.);
#2432=EDGE_CURVE('',#1963,#1966,#972,.T.);
#2433=EDGE_CURVE('',#1967,#1968,#1641,.T.);
#2434=EDGE_CURVE('',#1968,#1969,#973,.T.);
#2435=EDGE_CURVE('',#1969,#1970,#1642,.F.);
#2436=EDGE_CURVE('',#1970,#1967,#974,.T.);
#2437=EDGE_CURVE('',#1968,#1971,#975,.T.);
#2438=EDGE_CURVE('',#1971,#1972,#976,.T.);
#2439=EDGE_CURVE('',#1969,#1972,#977,.T.);
#2440=EDGE_CURVE('',#1973,#1974,#1643,.F.);
#2441=EDGE_CURVE('',#1974,#1975,#978,.T.);
#2442=EDGE_CURVE('',#1975,#1976,#1644,.T.);
#2443=EDGE_CURVE('',#1976,#1973,#979,.T.);
#2444=EDGE_CURVE('',#1977,#1974,#980,.T.);
#2445=EDGE_CURVE('',#1978,#1977,#981,.T.);
#2446=EDGE_CURVE('',#1975,#1978,#982,.T.);
#2447=EDGE_CURVE('',#1979,#1980,#1645,.T.);
#2448=EDGE_CURVE('',#1980,#1981,#983,.T.);
#2449=EDGE_CURVE('',#1981,#1982,#1646,.F.);
#2450=EDGE_CURVE('',#1982,#1979,#984,.T.);
#2451=EDGE_CURVE('',#1980,#1983,#985,.T.);
#2452=EDGE_CURVE('',#1983,#1984,#986,.T.);
#2453=EDGE_CURVE('',#1981,#1984,#987,.T.);
#2454=EDGE_CURVE('',#1985,#1986,#1647,.F.);
#2455=EDGE_CURVE('',#1986,#1987,#988,.T.);
#2456=EDGE_CURVE('',#1987,#1988,#1648,.T.);
#2457=EDGE_CURVE('',#1988,#1985,#989,.T.);
#2458=EDGE_CURVE('',#1989,#1986,#990,.T.);
#2459=EDGE_CURVE('',#1990,#1989,#991,.T.);
#2460=EDGE_CURVE('',#1987,#1990,#992,.T.);
#2461=EDGE_CURVE('',#1991,#1992,#1649,.T.);
#2462=EDGE_CURVE('',#1992,#1993,#993,.T.);
#2463=EDGE_CURVE('',#1993,#1994,#1650,.F.);
#2464=EDGE_CURVE('',#1994,#1991,#994,.T.);
#2465=EDGE_CURVE('',#1992,#1995,#995,.T.);
#2466=EDGE_CURVE('',#1995,#1996,#996,.T.);
#2467=EDGE_CURVE('',#1993,#1996,#997,.T.);
#2468=EDGE_CURVE('',#1997,#1998,#1651,.F.);
#2469=EDGE_CURVE('',#1998,#1999,#998,.T.);
#2470=EDGE_CURVE('',#1999,#2000,#1652,.T.);
#2471=EDGE_CURVE('',#2000,#1997,#999,.T.);
#2472=EDGE_CURVE('',#2001,#1998,#1000,.T.);
#2473=EDGE_CURVE('',#2002,#2001,#1001,.T.);
#2474=EDGE_CURVE('',#1999,#2002,#1002,.T.);
#2475=EDGE_CURVE('',#2003,#2004,#1653,.T.);
#2476=EDGE_CURVE('',#2004,#2005,#1003,.T.);
#2477=EDGE_CURVE('',#2005,#2006,#1654,.F.);
#2478=EDGE_CURVE('',#2006,#2003,#1004,.T.);
#2479=EDGE_CURVE('',#2004,#2007,#1005,.T.);
#2480=EDGE_CURVE('',#2007,#2008,#1006,.T.);
#2481=EDGE_CURVE('',#2005,#2008,#1007,.T.);
#2482=EDGE_CURVE('',#2009,#2010,#1655,.F.);
#2483=EDGE_CURVE('',#2010,#2011,#1008,.T.);
#2484=EDGE_CURVE('',#2011,#2012,#1656,.T.);
#2485=EDGE_CURVE('',#2012,#2009,#1009,.T.);
#2486=EDGE_CURVE('',#2013,#2010,#1010,.T.);
#2487=EDGE_CURVE('',#2014,#2013,#1011,.T.);
#2488=EDGE_CURVE('',#2011,#2014,#1012,.T.);
#2489=EDGE_CURVE('',#2015,#2016,#1657,.T.);
#2490=EDGE_CURVE('',#2016,#2017,#1013,.T.);
#2491=EDGE_CURVE('',#2017,#2018,#1658,.F.);
#2492=EDGE_CURVE('',#2018,#2015,#1014,.T.);
#2493=EDGE_CURVE('',#2016,#2019,#1015,.T.);
#2494=EDGE_CURVE('',#2019,#2020,#1016,.T.);
#2495=EDGE_CURVE('',#2017,#2020,#1017,.T.);
#2496=EDGE_CURVE('',#2021,#2022,#1659,.F.);
#2497=EDGE_CURVE('',#2022,#2023,#1018,.T.);
#2498=EDGE_CURVE('',#2023,#2024,#1660,.T.);
#2499=EDGE_CURVE('',#2024,#2021,#1019,.T.);
#2500=EDGE_CURVE('',#2025,#2022,#1020,.T.);
#2501=EDGE_CURVE('',#2026,#2025,#1021,.T.);
#2502=EDGE_CURVE('',#2023,#2026,#1022,.T.);
#2503=EDGE_CURVE('',#2027,#2028,#1661,.T.);
#2504=EDGE_CURVE('',#2028,#2029,#1023,.T.);
#2505=EDGE_CURVE('',#2029,#2030,#1662,.F.);
#2506=EDGE_CURVE('',#2030,#2027,#1024,.T.);
#2507=EDGE_CURVE('',#2028,#2031,#1025,.T.);
#2508=EDGE_CURVE('',#2031,#2032,#1026,.T.);
#2509=EDGE_CURVE('',#2029,#2032,#1027,.T.);
#2510=EDGE_CURVE('',#2033,#2034,#1663,.F.);
#2511=EDGE_CURVE('',#2034,#2035,#1028,.T.);
#2512=EDGE_CURVE('',#2035,#2036,#1664,.T.);
#2513=EDGE_CURVE('',#2036,#2033,#1029,.T.);
#2514=EDGE_CURVE('',#2037,#2034,#1030,.T.);
#2515=EDGE_CURVE('',#2038,#2037,#1031,.T.);
#2516=EDGE_CURVE('',#2035,#2038,#1032,.T.);
#2517=EDGE_CURVE('',#2039,#2040,#1665,.T.);
#2518=EDGE_CURVE('',#2040,#2041,#1033,.T.);
#2519=EDGE_CURVE('',#2041,#2042,#1666,.F.);
#2520=EDGE_CURVE('',#2042,#2039,#1034,.T.);
#2521=EDGE_CURVE('',#2040,#2043,#1035,.T.);
#2522=EDGE_CURVE('',#2043,#2044,#1036,.T.);
#2523=EDGE_CURVE('',#2041,#2044,#1037,.T.);
#2524=EDGE_CURVE('',#2045,#2046,#1667,.F.);
#2525=EDGE_CURVE('',#2046,#2047,#1038,.T.);
#2526=EDGE_CURVE('',#2047,#2048,#1668,.T.);
#2527=EDGE_CURVE('',#2048,#2045,#1039,.T.);
#2528=EDGE_CURVE('',#2049,#2046,#1040,.T.);
#2529=EDGE_CURVE('',#2050,#2049,#1041,.T.);
#2530=EDGE_CURVE('',#2047,#2050,#1042,.T.);
#2531=EDGE_CURVE('',#2051,#2052,#1669,.T.);
#2532=EDGE_CURVE('',#2052,#2053,#1043,.T.);
#2533=EDGE_CURVE('',#2053,#2054,#1670,.F.);
#2534=EDGE_CURVE('',#2054,#2051,#1044,.T.);
#2535=EDGE_CURVE('',#2052,#2055,#1045,.T.);
#2536=EDGE_CURVE('',#2055,#2056,#1046,.T.);
#2537=EDGE_CURVE('',#2053,#2056,#1047,.T.);
#2538=EDGE_CURVE('',#2057,#2058,#1671,.F.);
#2539=EDGE_CURVE('',#2058,#2059,#1048,.T.);
#2540=EDGE_CURVE('',#2059,#2060,#1672,.T.);
#2541=EDGE_CURVE('',#2060,#2057,#1049,.T.);
#2542=EDGE_CURVE('',#2061,#2058,#1050,.T.);
#2543=EDGE_CURVE('',#2062,#2061,#1051,.T.);
#2544=EDGE_CURVE('',#2059,#2062,#1052,.T.);
#2545=EDGE_CURVE('',#2063,#2064,#1673,.T.);
#2546=EDGE_CURVE('',#2064,#2065,#1053,.T.);
#2547=EDGE_CURVE('',#2065,#2066,#1674,.F.);
#2548=EDGE_CURVE('',#2066,#2063,#1054,.T.);
#2549=EDGE_CURVE('',#2064,#2067,#1055,.T.);
#2550=EDGE_CURVE('',#2067,#2068,#1056,.T.);
#2551=EDGE_CURVE('',#2065,#2068,#1057,.T.);
#2552=EDGE_CURVE('',#2069,#2070,#1675,.F.);
#2553=EDGE_CURVE('',#2070,#2071,#1058,.T.);
#2554=EDGE_CURVE('',#2071,#2072,#1676,.T.);
#2555=EDGE_CURVE('',#2072,#2069,#1059,.T.);
#2556=EDGE_CURVE('',#2073,#2070,#1060,.T.);
#2557=EDGE_CURVE('',#2074,#2073,#1061,.T.);
#2558=EDGE_CURVE('',#2071,#2074,#1062,.T.);
#2559=EDGE_CURVE('',#2075,#2076,#1677,.T.);
#2560=EDGE_CURVE('',#2076,#2077,#1063,.T.);
#2561=EDGE_CURVE('',#2077,#2078,#1678,.F.);
#2562=EDGE_CURVE('',#2078,#2075,#1064,.T.);
#2563=EDGE_CURVE('',#2076,#2079,#1065,.T.);
#2564=EDGE_CURVE('',#2079,#2080,#1066,.T.);
#2565=EDGE_CURVE('',#2077,#2080,#1067,.T.);
#2566=EDGE_CURVE('',#2081,#2082,#1679,.F.);
#2567=EDGE_CURVE('',#2082,#2083,#1068,.T.);
#2568=EDGE_CURVE('',#2083,#2084,#1680,.T.);
#2569=EDGE_CURVE('',#2084,#2081,#1069,.T.);
#2570=EDGE_CURVE('',#2085,#2082,#1070,.T.);
#2571=EDGE_CURVE('',#2086,#2085,#1071,.T.);
#2572=EDGE_CURVE('',#2083,#2086,#1072,.T.);
#2573=EDGE_CURVE('',#2087,#2088,#1681,.T.);
#2574=EDGE_CURVE('',#2088,#2089,#1073,.T.);
#2575=EDGE_CURVE('',#2089,#2090,#1682,.F.);
#2576=EDGE_CURVE('',#2090,#2087,#1074,.T.);
#2577=EDGE_CURVE('',#2088,#2091,#1075,.T.);
#2578=EDGE_CURVE('',#2091,#2092,#1076,.T.);
#2579=EDGE_CURVE('',#2089,#2092,#1077,.T.);
#2580=EDGE_CURVE('',#2093,#2094,#1683,.F.);
#2581=EDGE_CURVE('',#2094,#2095,#1078,.T.);
#2582=EDGE_CURVE('',#2095,#2096,#1684,.T.);
#2583=EDGE_CURVE('',#2096,#2093,#1079,.T.);
#2584=EDGE_CURVE('',#2097,#2094,#1080,.T.);
#2585=EDGE_CURVE('',#2098,#2097,#1081,.T.);
#2586=EDGE_CURVE('',#2095,#2098,#1082,.T.);
#2587=EDGE_CURVE('',#2099,#2100,#1685,.T.);
#2588=EDGE_CURVE('',#2100,#2101,#1083,.T.);
#2589=EDGE_CURVE('',#2101,#2102,#1686,.F.);
#2590=EDGE_CURVE('',#2102,#2099,#1084,.T.);
#2591=EDGE_CURVE('',#2100,#2103,#1085,.T.);
#2592=EDGE_CURVE('',#2103,#2104,#1086,.T.);
#2593=EDGE_CURVE('',#2101,#2104,#1087,.T.);
#2594=EDGE_CURVE('',#1882,#2105,#111,.T.);
#2595=EDGE_CURVE('',#2106,#1881,#112,.T.);
#2596=EDGE_CURVE('',#2105,#2106,#1088,.T.);
#2597=EDGE_CURVE('',#2107,#2105,#1687,.T.);
#2598=EDGE_CURVE('',#2108,#2106,#1688,.T.);
#2599=EDGE_CURVE('',#2107,#2108,#1089,.T.);
#2600=EDGE_CURVE('',#1887,#2107,#113,.T.);
#2601=EDGE_CURVE('',#1888,#2108,#114,.T.);
#2602=EDGE_CURVE('',#1894,#2109,#115,.T.);
#2603=EDGE_CURVE('',#2110,#1893,#116,.T.);
#2604=EDGE_CURVE('',#2109,#2110,#1090,.T.);
#2605=EDGE_CURVE('',#2111,#2109,#1689,.T.);
#2606=EDGE_CURVE('',#2112,#2110,#1690,.T.);
#2607=EDGE_CURVE('',#2111,#2112,#1091,.T.);
#2608=EDGE_CURVE('',#1899,#2111,#117,.T.);
#2609=EDGE_CURVE('',#1900,#2112,#118,.T.);
#2610=EDGE_CURVE('',#1906,#2113,#119,.T.);
#2611=EDGE_CURVE('',#2114,#1905,#120,.T.);
#2612=EDGE_CURVE('',#2113,#2114,#1092,.T.);
#2613=EDGE_CURVE('',#2115,#2113,#1691,.T.);
#2614=EDGE_CURVE('',#2116,#2114,#1692,.T.);
#2615=EDGE_CURVE('',#2115,#2116,#1093,.T.);
#2616=EDGE_CURVE('',#1911,#2115,#121,.T.);
#2617=EDGE_CURVE('',#1912,#2116,#122,.T.);
#2618=EDGE_CURVE('',#1918,#2117,#123,.T.);
#2619=EDGE_CURVE('',#2118,#1917,#124,.T.);
#2620=EDGE_CURVE('',#2117,#2118,#1094,.T.);
#2621=EDGE_CURVE('',#2119,#2117,#1693,.T.);
#2622=EDGE_CURVE('',#2120,#2118,#1694,.T.);
#2623=EDGE_CURVE('',#2119,#2120,#1095,.T.);
#2624=EDGE_CURVE('',#1923,#2119,#125,.T.);
#2625=EDGE_CURVE('',#1924,#2120,#126,.T.);
#2626=EDGE_CURVE('',#1930,#2121,#127,.T.);
#2627=EDGE_CURVE('',#2122,#1929,#128,.T.);
#2628=EDGE_CURVE('',#2121,#2122,#1096,.T.);
#2629=EDGE_CURVE('',#2123,#2121,#1695,.T.);
#2630=EDGE_CURVE('',#2124,#2122,#1696,.T.);
#2631=EDGE_CURVE('',#2123,#2124,#1097,.T.);
#2632=EDGE_CURVE('',#1935,#2123,#129,.T.);
#2633=EDGE_CURVE('',#1936,#2124,#130,.T.);
#2634=EDGE_CURVE('',#1942,#2125,#131,.T.);
#2635=EDGE_CURVE('',#2126,#1941,#132,.T.);
#2636=EDGE_CURVE('',#2125,#2126,#1098,.T.);
#2637=EDGE_CURVE('',#2127,#2125,#1697,.T.);
#2638=EDGE_CURVE('',#2128,#2126,#1698,.T.);
#2639=EDGE_CURVE('',#2127,#2128,#1099,.T.);
#2640=EDGE_CURVE('',#1947,#2127,#133,.T.);
#2641=EDGE_CURVE('',#1948,#2128,#134,.T.);
#2642=EDGE_CURVE('',#1954,#2129,#135,.T.);
#2643=EDGE_CURVE('',#2130,#1953,#136,.T.);
#2644=EDGE_CURVE('',#2129,#2130,#1100,.T.);
#2645=EDGE_CURVE('',#2131,#2129,#1699,.T.);
#2646=EDGE_CURVE('',#2132,#2130,#1700,.T.);
#2647=EDGE_CURVE('',#2131,#2132,#1101,.T.);
#2648=EDGE_CURVE('',#1959,#2131,#137,.T.);
#2649=EDGE_CURVE('',#1960,#2132,#138,.T.);
#2650=EDGE_CURVE('',#1966,#2133,#139,.T.);
#2651=EDGE_CURVE('',#2134,#1965,#140,.T.);
#2652=EDGE_CURVE('',#2133,#2134,#1102,.T.);
#2653=EDGE_CURVE('',#2135,#2133,#1701,.T.);
#2654=EDGE_CURVE('',#2136,#2134,#1702,.T.);
#2655=EDGE_CURVE('',#2135,#2136,#1103,.T.);
#2656=EDGE_CURVE('',#1971,#2135,#141,.T.);
#2657=EDGE_CURVE('',#1972,#2136,#142,.T.);
#2658=EDGE_CURVE('',#1978,#2137,#143,.T.);
#2659=EDGE_CURVE('',#2138,#1977,#144,.T.);
#2660=EDGE_CURVE('',#2137,#2138,#1104,.T.);
#2661=EDGE_CURVE('',#2139,#2137,#1703,.T.);
#2662=EDGE_CURVE('',#2140,#2138,#1704,.T.);
#2663=EDGE_CURVE('',#2139,#2140,#1105,.T.);
#2664=EDGE_CURVE('',#1983,#2139,#145,.T.);
#2665=EDGE_CURVE('',#1984,#2140,#146,.T.);
#2666=EDGE_CURVE('',#1990,#2141,#147,.T.);
#2667=EDGE_CURVE('',#2142,#1989,#148,.T.);
#2668=EDGE_CURVE('',#2141,#2142,#1106,.T.);
#2669=EDGE_CURVE('',#2143,#2141,#1705,.T.);
#2670=EDGE_CURVE('',#2144,#2142,#1706,.T.);
#2671=EDGE_CURVE('',#2143,#2144,#1107,.T.);
#2672=EDGE_CURVE('',#1995,#2143,#149,.T.);
#2673=EDGE_CURVE('',#1996,#2144,#150,.T.);
#2674=EDGE_CURVE('',#2002,#2145,#151,.T.);
#2675=EDGE_CURVE('',#2146,#2001,#152,.T.);
#2676=EDGE_CURVE('',#2145,#2146,#1108,.T.);
#2677=EDGE_CURVE('',#2147,#2145,#1707,.T.);
#2678=EDGE_CURVE('',#2148,#2146,#1708,.T.);
#2679=EDGE_CURVE('',#2147,#2148,#1109,.T.);
#2680=EDGE_CURVE('',#2007,#2147,#153,.T.);
#2681=EDGE_CURVE('',#2008,#2148,#154,.T.);
#2682=EDGE_CURVE('',#2014,#2149,#155,.T.);
#2683=EDGE_CURVE('',#2150,#2013,#156,.T.);
#2684=EDGE_CURVE('',#2149,#2150,#1110,.T.);
#2685=EDGE_CURVE('',#2151,#2149,#1709,.T.);
#2686=EDGE_CURVE('',#2152,#2150,#1710,.T.);
#2687=EDGE_CURVE('',#2151,#2152,#1111,.T.);
#2688=EDGE_CURVE('',#2019,#2151,#157,.T.);
#2689=EDGE_CURVE('',#2020,#2152,#158,.T.);
#2690=EDGE_CURVE('',#2026,#2153,#159,.T.);
#2691=EDGE_CURVE('',#2154,#2025,#160,.T.);
#2692=EDGE_CURVE('',#2153,#2154,#1112,.T.);
#2693=EDGE_CURVE('',#2155,#2153,#1711,.T.);
#2694=EDGE_CURVE('',#2156,#2154,#1712,.T.);
#2695=EDGE_CURVE('',#2155,#2156,#1113,.T.);
#2696=EDGE_CURVE('',#2031,#2155,#161,.T.);
#2697=EDGE_CURVE('',#2032,#2156,#162,.T.);
#2698=EDGE_CURVE('',#2038,#2157,#163,.T.);
#2699=EDGE_CURVE('',#2158,#2037,#164,.T.);
#2700=EDGE_CURVE('',#2157,#2158,#1114,.T.);
#2701=EDGE_CURVE('',#2159,#2157,#1713,.T.);
#2702=EDGE_CURVE('',#2160,#2158,#1714,.T.);
#2703=EDGE_CURVE('',#2159,#2160,#1115,.T.);
#2704=EDGE_CURVE('',#2043,#2159,#165,.T.);
#2705=EDGE_CURVE('',#2044,#2160,#166,.T.);
#2706=EDGE_CURVE('',#2050,#2161,#167,.T.);
#2707=EDGE_CURVE('',#2162,#2049,#168,.T.);
#2708=EDGE_CURVE('',#2161,#2162,#1116,.T.);
#2709=EDGE_CURVE('',#2163,#2161,#1715,.T.);
#2710=EDGE_CURVE('',#2164,#2162,#1716,.T.);
#2711=EDGE_CURVE('',#2163,#2164,#1117,.T.);
#2712=EDGE_CURVE('',#2055,#2163,#169,.T.);
#2713=EDGE_CURVE('',#2056,#2164,#170,.T.);
#2714=EDGE_CURVE('',#2062,#2165,#171,.T.);
#2715=EDGE_CURVE('',#2166,#2061,#172,.T.);
#2716=EDGE_CURVE('',#2165,#2166,#1118,.T.);
#2717=EDGE_CURVE('',#2167,#2165,#1717,.T.);
#2718=EDGE_CURVE('',#2168,#2166,#1718,.T.);
#2719=EDGE_CURVE('',#2167,#2168,#1119,.T.);
#2720=EDGE_CURVE('',#2067,#2167,#173,.T.);
#2721=EDGE_CURVE('',#2068,#2168,#174,.T.);
#2722=EDGE_CURVE('',#2074,#2169,#175,.T.);
#2723=EDGE_CURVE('',#2170,#2073,#176,.T.);
#2724=EDGE_CURVE('',#2169,#2170,#1120,.T.);
#2725=EDGE_CURVE('',#2171,#2169,#1719,.T.);
#2726=EDGE_CURVE('',#2172,#2170,#1720,.T.);
#2727=EDGE_CURVE('',#2171,#2172,#1121,.T.);
#2728=EDGE_CURVE('',#2079,#2171,#177,.T.);
#2729=EDGE_CURVE('',#2080,#2172,#178,.T.);
#2730=EDGE_CURVE('',#2086,#2173,#179,.T.);
#2731=EDGE_CURVE('',#2174,#2085,#180,.T.);
#2732=EDGE_CURVE('',#2173,#2174,#1122,.T.);
#2733=EDGE_CURVE('',#2175,#2173,#1721,.T.);
#2734=EDGE_CURVE('',#2176,#2174,#1722,.T.);
#2735=EDGE_CURVE('',#2175,#2176,#1123,.T.);
#2736=EDGE_CURVE('',#2091,#2175,#181,.T.);
#2737=EDGE_CURVE('',#2092,#2176,#182,.T.);
#2738=EDGE_CURVE('',#2098,#2177,#183,.T.);
#2739=EDGE_CURVE('',#2178,#2097,#184,.T.);
#2740=EDGE_CURVE('',#2177,#2178,#1124,.T.);
#2741=EDGE_CURVE('',#2179,#2177,#1723,.T.);
#2742=EDGE_CURVE('',#2180,#2178,#1724,.T.);
#2743=EDGE_CURVE('',#2179,#2180,#1125,.T.);
#2744=EDGE_CURVE('',#2103,#2179,#185,.T.);
#2745=EDGE_CURVE('',#2104,#2180,#186,.T.);
#2746=EDGE_CURVE('',#1904,#1895,#1725,.T.);
#2747=EDGE_CURVE('',#1916,#1907,#1726,.T.);
#2748=EDGE_CURVE('',#1928,#1919,#1727,.T.);
#2749=EDGE_CURVE('',#1940,#1931,#1728,.T.);
#2750=EDGE_CURVE('',#1952,#1943,#1729,.T.);
#2751=EDGE_CURVE('',#1964,#1955,#1730,.T.);
#2752=EDGE_CURVE('',#1976,#1967,#1731,.T.);
#2753=EDGE_CURVE('',#1988,#1979,#1732,.T.);
#2754=EDGE_CURVE('',#2000,#1991,#1733,.T.);
#2755=EDGE_CURVE('',#2012,#2003,#1734,.T.);
#2756=EDGE_CURVE('',#2024,#2015,#1735,.T.);
#2757=EDGE_CURVE('',#2036,#2027,#1736,.T.);
#2758=EDGE_CURVE('',#2048,#2039,#1737,.T.);
#2759=EDGE_CURVE('',#2060,#2051,#1738,.T.);
#2760=EDGE_CURVE('',#2072,#2063,#1739,.T.);
#2761=EDGE_CURVE('',#2084,#2075,#1740,.T.);
#2762=EDGE_CURVE('',#2096,#2087,#1741,.T.);
#2763=EDGE_CURVE('',#2181,#2099,#1742,.T.);
#2764=EDGE_CURVE('',#2182,#2181,#1743,.T.);
#2765=EDGE_CURVE('',#2182,#2183,#1126,.T.);
#2766=EDGE_CURVE('',#2183,#2184,#187,.T.);
#2767=EDGE_CURVE('',#2185,#2184,#1744,.T.);
#2768=EDGE_CURVE('',#2186,#2185,#188,.T.);
#2769=EDGE_CURVE('',#2187,#2186,#1127,.T.);
#2770=EDGE_CURVE('',#2188,#2187,#1745,.T.);
#2771=EDGE_CURVE('',#1880,#2188,#1746,.T.);
#2772=EDGE_CURVE('',#1892,#1883,#1747,.T.);
#2773=EDGE_CURVE('',#1877,#2189,#1748,.T.);
#2774=EDGE_CURVE('',#2190,#2189,#1749,.F.);
#2775=EDGE_CURVE('',#2190,#2191,#1128,.T.);
#2776=EDGE_CURVE('',#2191,#2192,#189,.T.);
#2777=EDGE_CURVE('',#2192,#2193,#1750,.T.);
#2778=EDGE_CURVE('',#2193,#2194,#190,.T.);
#2779=EDGE_CURVE('',#2194,#2195,#1129,.T.);
#2780=EDGE_CURVE('',#2196,#2195,#1751,.F.);
#2781=EDGE_CURVE('',#2196,#2102,#1752,.T.);
#2782=EDGE_CURVE('',#2093,#2090,#1753,.T.);
#2783=EDGE_CURVE('',#2081,#2078,#1754,.T.);
#2784=EDGE_CURVE('',#2069,#2066,#1755,.T.);
#2785=EDGE_CURVE('',#2057,#2054,#1756,.T.);
#2786=EDGE_CURVE('',#2045,#2042,#1757,.T.);
#2787=EDGE_CURVE('',#2033,#2030,#1758,.T.);
#2788=EDGE_CURVE('',#2021,#2018,#1759,.T.);
#2789=EDGE_CURVE('',#2009,#2006,#1760,.T.);
#2790=EDGE_CURVE('',#1997,#1994,#1761,.T.);
#2791=EDGE_CURVE('',#1985,#1982,#1762,.T.);
#2792=EDGE_CURVE('',#1973,#1970,#1763,.T.);
#2793=EDGE_CURVE('',#1961,#1958,#1764,.T.);
#2794=EDGE_CURVE('',#1949,#1946,#1765,.T.);
#2795=EDGE_CURVE('',#1937,#1934,#1766,.T.);
#2796=EDGE_CURVE('',#1925,#1922,#1767,.T.);
#2797=EDGE_CURVE('',#1913,#1910,#1768,.T.);
#2798=EDGE_CURVE('',#1901,#1898,#1769,.T.);
#2799=EDGE_CURVE('',#1889,#1886,#1770,.T.);
#2800=EDGE_CURVE('',#2181,#2196,#1130,.T.);
#2801=EDGE_CURVE('',#2195,#2182,#1131,.T.);
#2802=EDGE_CURVE('',#2183,#2194,#1132,.T.);
#2803=EDGE_CURVE('',#2187,#2190,#1133,.T.);
#2804=EDGE_CURVE('',#2189,#2188,#1134,.T.);
#2805=EDGE_CURVE('',#2186,#2191,#1135,.T.);
#2806=EDGE_CURVE('',#2184,#2193,#1136,.T.);
#2807=EDGE_CURVE('',#2185,#2192,#1137,.T.);
#3027=ORIENTED_EDGE('',*,*,#2325,.F.);
#3028=ORIENTED_EDGE('',*,*,#2326,.T.);
#3029=ORIENTED_EDGE('',*,*,#2327,.F.);
#3030=ORIENTED_EDGE('',*,*,#2326,.F.);
#3031=ORIENTED_EDGE('',*,*,#2328,.T.);
#3032=ORIENTED_EDGE('',*,*,#2329,.T.);
#3033=ORIENTED_EDGE('',*,*,#2330,.T.);
#3034=ORIENTED_EDGE('',*,*,#2331,.T.);
#3035=ORIENTED_EDGE('',*,*,#2329,.F.);
#3036=ORIENTED_EDGE('',*,*,#2332,.F.);
#3037=ORIENTED_EDGE('',*,*,#2333,.F.);
#3038=ORIENTED_EDGE('',*,*,#2334,.F.);
#3039=ORIENTED_EDGE('',*,*,#2335,.T.);
#3040=ORIENTED_EDGE('',*,*,#2336,.T.);
#3041=ORIENTED_EDGE('',*,*,#2337,.T.);
#3042=ORIENTED_EDGE('',*,*,#2338,.T.);
#3043=ORIENTED_EDGE('',*,*,#2336,.F.);
#3044=ORIENTED_EDGE('',*,*,#2339,.T.);
#3045=ORIENTED_EDGE('',*,*,#2340,.T.);
#3046=ORIENTED_EDGE('',*,*,#2341,.F.);
#3047=ORIENTED_EDGE('',*,*,#2342,.T.);
#3048=ORIENTED_EDGE('',*,*,#2343,.T.);
#3049=ORIENTED_EDGE('',*,*,#2344,.T.);
#3050=ORIENTED_EDGE('',*,*,#2345,.T.);
#3051=ORIENTED_EDGE('',*,*,#2343,.F.);
#3052=ORIENTED_EDGE('',*,*,#2346,.F.);
#3053=ORIENTED_EDGE('',*,*,#2347,.F.);
#3054=ORIENTED_EDGE('',*,*,#2348,.F.);
#3055=ORIENTED_EDGE('',*,*,#2349,.T.);
#3056=ORIENTED_EDGE('',*,*,#2350,.T.);
#3057=ORIENTED_EDGE('',*,*,#2351,.T.);
#3058=ORIENTED_EDGE('',*,*,#2352,.T.);
#3059=ORIENTED_EDGE('',*,*,#2350,.F.);
#3060=ORIENTED_EDGE('',*,*,#2353,.T.);
#3061=ORIENTED_EDGE('',*,*,#2354,.T.);
#3062=ORIENTED_EDGE('',*,*,#2355,.F.);
#3063=ORIENTED_EDGE('',*,*,#2356,.T.);
#3064=ORIENTED_EDGE('',*,*,#2357,.T.);
#3065=ORIENTED_EDGE('',*,*,#2358,.T.);
#3066=ORIENTED_EDGE('',*,*,#2359,.T.);
#3067=ORIENTED_EDGE('',*,*,#2357,.F.);
#3068=ORIENTED_EDGE('',*,*,#2360,.F.);
#3069=ORIENTED_EDGE('',*,*,#2361,.F.);
#3070=ORIENTED_EDGE('',*,*,#2362,.F.);
#3071=ORIENTED_EDGE('',*,*,#2363,.T.);
#3072=ORIENTED_EDGE('',*,*,#2364,.T.);
#3073=ORIENTED_EDGE('',*,*,#2365,.T.);
#3074=ORIENTED_EDGE('',*,*,#2366,.T.);
#3075=ORIENTED_EDGE('',*,*,#2364,.F.);
#3076=ORIENTED_EDGE('',*,*,#2367,.T.);
#3077=ORIENTED_EDGE('',*,*,#2368,.T.);
#3078=ORIENTED_EDGE('',*,*,#2369,.F.);
#3079=ORIENTED_EDGE('',*,*,#2370,.T.);
#3080=ORIENTED_EDGE('',*,*,#2371,.T.);
#3081=ORIENTED_EDGE('',*,*,#2372,.T.);
#3082=ORIENTED_EDGE('',*,*,#2373,.T.);
#3083=ORIENTED_EDGE('',*,*,#2371,.F.);
#3084=ORIENTED_EDGE('',*,*,#2374,.F.);
#3085=ORIENTED_EDGE('',*,*,#2375,.F.);
#3086=ORIENTED_EDGE('',*,*,#2376,.F.);
#3087=ORIENTED_EDGE('',*,*,#2377,.T.);
#3088=ORIENTED_EDGE('',*,*,#2378,.T.);
#3089=ORIENTED_EDGE('',*,*,#2379,.T.);
#3090=ORIENTED_EDGE('',*,*,#2380,.T.);
#3091=ORIENTED_EDGE('',*,*,#2378,.F.);
#3092=ORIENTED_EDGE('',*,*,#2381,.T.);
#3093=ORIENTED_EDGE('',*,*,#2382,.T.);
#3094=ORIENTED_EDGE('',*,*,#2383,.F.);
#3095=ORIENTED_EDGE('',*,*,#2384,.T.);
#3096=ORIENTED_EDGE('',*,*,#2385,.T.);
#3097=ORIENTED_EDGE('',*,*,#2386,.T.);
#3098=ORIENTED_EDGE('',*,*,#2387,.T.);
#3099=ORIENTED_EDGE('',*,*,#2385,.F.);
#3100=ORIENTED_EDGE('',*,*,#2388,.F.);
#3101=ORIENTED_EDGE('',*,*,#2389,.F.);
#3102=ORIENTED_EDGE('',*,*,#2390,.F.);
#3103=ORIENTED_EDGE('',*,*,#2391,.T.);
#3104=ORIENTED_EDGE('',*,*,#2392,.T.);
#3105=ORIENTED_EDGE('',*,*,#2393,.T.);
#3106=ORIENTED_EDGE('',*,*,#2394,.T.);
#3107=ORIENTED_EDGE('',*,*,#2392,.F.);
#3108=ORIENTED_EDGE('',*,*,#2395,.T.);
#3109=ORIENTED_EDGE('',*,*,#2396,.T.);
#3110=ORIENTED_EDGE('',*,*,#2397,.F.);
#3111=ORIENTED_EDGE('',*,*,#2398,.T.);
#3112=ORIENTED_EDGE('',*,*,#2399,.T.);
#3113=ORIENTED_EDGE('',*,*,#2400,.T.);
#3114=ORIENTED_EDGE('',*,*,#2401,.T.);
#3115=ORIENTED_EDGE('',*,*,#2399,.F.);
#3116=ORIENTED_EDGE('',*,*,#2402,.F.);
#3117=ORIENTED_EDGE('',*,*,#2403,.F.);
#3118=ORIENTED_EDGE('',*,*,#2404,.F.);
#3119=ORIENTED_EDGE('',*,*,#2405,.T.);
#3120=ORIENTED_EDGE('',*,*,#2406,.T.);
#3121=ORIENTED_EDGE('',*,*,#2407,.T.);
#3122=ORIENTED_EDGE('',*,*,#2408,.T.);
#3123=ORIENTED_EDGE('',*,*,#2406,.F.);
#3124=ORIENTED_EDGE('',*,*,#2409,.T.);
#3125=ORIENTED_EDGE('',*,*,#2410,.T.);
#3126=ORIENTED_EDGE('',*,*,#2411,.F.);
#3127=ORIENTED_EDGE('',*,*,#2412,.T.);
#3128=ORIENTED_EDGE('',*,*,#2413,.T.);
#3129=ORIENTED_EDGE('',*,*,#2414,.T.);
#3130=ORIENTED_EDGE('',*,*,#2415,.T.);
#3131=ORIENTED_EDGE('',*,*,#2413,.F.);
#3132=ORIENTED_EDGE('',*,*,#2416,.F.);
#3133=ORIENTED_EDGE('',*,*,#2417,.F.);
#3134=ORIENTED_EDGE('',*,*,#2418,.F.);
#3135=ORIENTED_EDGE('',*,*,#2419,.T.);
#3136=ORIENTED_EDGE('',*,*,#2420,.T.);
#3137=ORIENTED_EDGE('',*,*,#2421,.T.);
#3138=ORIENTED_EDGE('',*,*,#2422,.T.);
#3139=ORIENTED_EDGE('',*,*,#2420,.F.);
#3140=ORIENTED_EDGE('',*,*,#2423,.T.);
#3141=ORIENTED_EDGE('',*,*,#2424,.T.);
#3142=ORIENTED_EDGE('',*,*,#2425,.F.);
#3143=ORIENTED_EDGE('',*,*,#2426,.T.);
#3144=ORIENTED_EDGE('',*,*,#2427,.T.);
#3145=ORIENTED_EDGE('',*,*,#2428,.T.);
#3146=ORIENTED_EDGE('',*,*,#2429,.T.);
#3147=ORIENTED_EDGE('',*,*,#2427,.F.);
#3148=ORIENTED_EDGE('',*,*,#2430,.F.);
#3149=ORIENTED_EDGE('',*,*,#2431,.F.);
#3150=ORIENTED_EDGE('',*,*,#2432,.F.);
#3151=ORIENTED_EDGE('',*,*,#2433,.T.);
#3152=ORIENTED_EDGE('',*,*,#2434,.T.);
#3153=ORIENTED_EDGE('',*,*,#2435,.T.);
#3154=ORIENTED_EDGE('',*,*,#2436,.T.);
#3155=ORIENTED_EDGE('',*,*,#2434,.F.);
#3156=ORIENTED_EDGE('',*,*,#2437,.T.);
#3157=ORIENTED_EDGE('',*,*,#2438,.T.);
#3158=ORIENTED_EDGE('',*,*,#2439,.F.);
#3159=ORIENTED_EDGE('',*,*,#2440,.T.);
#3160=ORIENTED_EDGE('',*,*,#2441,.T.);
#3161=ORIENTED_EDGE('',*,*,#2442,.T.);
#3162=ORIENTED_EDGE('',*,*,#2443,.T.);
#3163=ORIENTED_EDGE('',*,*,#2441,.F.);
#3164=ORIENTED_EDGE('',*,*,#2444,.F.);
#3165=ORIENTED_EDGE('',*,*,#2445,.F.);
#3166=ORIENTED_EDGE('',*,*,#2446,.F.);
#3167=ORIENTED_EDGE('',*,*,#2447,.T.);
#3168=ORIENTED_EDGE('',*,*,#2448,.T.);
#3169=ORIENTED_EDGE('',*,*,#2449,.T.);
#3170=ORIENTED_EDGE('',*,*,#2450,.T.);
#3171=ORIENTED_EDGE('',*,*,#2448,.F.);
#3172=ORIENTED_EDGE('',*,*,#2451,.T.);
#3173=ORIENTED_EDGE('',*,*,#2452,.T.);
#3174=ORIENTED_EDGE('',*,*,#2453,.F.);
#3175=ORIENTED_EDGE('',*,*,#2454,.T.);
#3176=ORIENTED_EDGE('',*,*,#2455,.T.);
#3177=ORIENTED_EDGE('',*,*,#2456,.T.);
#3178=ORIENTED_EDGE('',*,*,#2457,.T.);
#3179=ORIENTED_EDGE('',*,*,#2455,.F.);
#3180=ORIENTED_EDGE('',*,*,#2458,.F.);
#3181=ORIENTED_EDGE('',*,*,#2459,.F.);
#3182=ORIENTED_EDGE('',*,*,#2460,.F.);
#3183=ORIENTED_EDGE('',*,*,#2461,.T.);
#3184=ORIENTED_EDGE('',*,*,#2462,.T.);
#3185=ORIENTED_EDGE('',*,*,#2463,.T.);
#3186=ORIENTED_EDGE('',*,*,#2464,.T.);
#3187=ORIENTED_EDGE('',*,*,#2462,.F.);
#3188=ORIENTED_EDGE('',*,*,#2465,.T.);
#3189=ORIENTED_EDGE('',*,*,#2466,.T.);
#3190=ORIENTED_EDGE('',*,*,#2467,.F.);
#3191=ORIENTED_EDGE('',*,*,#2468,.T.);
#3192=ORIENTED_EDGE('',*,*,#2469,.T.);
#3193=ORIENTED_EDGE('',*,*,#2470,.T.);
#3194=ORIENTED_EDGE('',*,*,#2471,.T.);
#3195=ORIENTED_EDGE('',*,*,#2469,.F.);
#3196=ORIENTED_EDGE('',*,*,#2472,.F.);
#3197=ORIENTED_EDGE('',*,*,#2473,.F.);
#3198=ORIENTED_EDGE('',*,*,#2474,.F.);
#3199=ORIENTED_EDGE('',*,*,#2475,.T.);
#3200=ORIENTED_EDGE('',*,*,#2476,.T.);
#3201=ORIENTED_EDGE('',*,*,#2477,.T.);
#3202=ORIENTED_EDGE('',*,*,#2478,.T.);
#3203=ORIENTED_EDGE('',*,*,#2476,.F.);
#3204=ORIENTED_EDGE('',*,*,#2479,.T.);
#3205=ORIENTED_EDGE('',*,*,#2480,.T.);
#3206=ORIENTED_EDGE('',*,*,#2481,.F.);
#3207=ORIENTED_EDGE('',*,*,#2482,.T.);
#3208=ORIENTED_EDGE('',*,*,#2483,.T.);
#3209=ORIENTED_EDGE('',*,*,#2484,.T.);
#3210=ORIENTED_EDGE('',*,*,#2485,.T.);
#3211=ORIENTED_EDGE('',*,*,#2483,.F.);
#3212=ORIENTED_EDGE('',*,*,#2486,.F.);
#3213=ORIENTED_EDGE('',*,*,#2487,.F.);
#3214=ORIENTED_EDGE('',*,*,#2488,.F.);
#3215=ORIENTED_EDGE('',*,*,#2489,.T.);
#3216=ORIENTED_EDGE('',*,*,#2490,.T.);
#3217=ORIENTED_EDGE('',*,*,#2491,.T.);
#3218=ORIENTED_EDGE('',*,*,#2492,.T.);
#3219=ORIENTED_EDGE('',*,*,#2490,.F.);
#3220=ORIENTED_EDGE('',*,*,#2493,.T.);
#3221=ORIENTED_EDGE('',*,*,#2494,.T.);
#3222=ORIENTED_EDGE('',*,*,#2495,.F.);
#3223=ORIENTED_EDGE('',*,*,#2496,.T.);
#3224=ORIENTED_EDGE('',*,*,#2497,.T.);
#3225=ORIENTED_EDGE('',*,*,#2498,.T.);
#3226=ORIENTED_EDGE('',*,*,#2499,.T.);
#3227=ORIENTED_EDGE('',*,*,#2497,.F.);
#3228=ORIENTED_EDGE('',*,*,#2500,.F.);
#3229=ORIENTED_EDGE('',*,*,#2501,.F.);
#3230=ORIENTED_EDGE('',*,*,#2502,.F.);
#3231=ORIENTED_EDGE('',*,*,#2503,.T.);
#3232=ORIENTED_EDGE('',*,*,#2504,.T.);
#3233=ORIENTED_EDGE('',*,*,#2505,.T.);
#3234=ORIENTED_EDGE('',*,*,#2506,.T.);
#3235=ORIENTED_EDGE('',*,*,#2504,.F.);
#3236=ORIENTED_EDGE('',*,*,#2507,.T.);
#3237=ORIENTED_EDGE('',*,*,#2508,.T.);
#3238=ORIENTED_EDGE('',*,*,#2509,.F.);
#3239=ORIENTED_EDGE('',*,*,#2510,.T.);
#3240=ORIENTED_EDGE('',*,*,#2511,.T.);
#3241=ORIENTED_EDGE('',*,*,#2512,.T.);
#3242=ORIENTED_EDGE('',*,*,#2513,.T.);
#3243=ORIENTED_EDGE('',*,*,#2511,.F.);
#3244=ORIENTED_EDGE('',*,*,#2514,.F.);
#3245=ORIENTED_EDGE('',*,*,#2515,.F.);
#3246=ORIENTED_EDGE('',*,*,#2516,.F.);
#3247=ORIENTED_EDGE('',*,*,#2517,.T.);
#3248=ORIENTED_EDGE('',*,*,#2518,.T.);
#3249=ORIENTED_EDGE('',*,*,#2519,.T.);
#3250=ORIENTED_EDGE('',*,*,#2520,.T.);
#3251=ORIENTED_EDGE('',*,*,#2518,.F.);
#3252=ORIENTED_EDGE('',*,*,#2521,.T.);
#3253=ORIENTED_EDGE('',*,*,#2522,.T.);
#3254=ORIENTED_EDGE('',*,*,#2523,.F.);
#3255=ORIENTED_EDGE('',*,*,#2524,.T.);
#3256=ORIENTED_EDGE('',*,*,#2525,.T.);
#3257=ORIENTED_EDGE('',*,*,#2526,.T.);
#3258=ORIENTED_EDGE('',*,*,#2527,.T.);
#3259=ORIENTED_EDGE('',*,*,#2525,.F.);
#3260=ORIENTED_EDGE('',*,*,#2528,.F.);
#3261=ORIENTED_EDGE('',*,*,#2529,.F.);
#3262=ORIENTED_EDGE('',*,*,#2530,.F.);
#3263=ORIENTED_EDGE('',*,*,#2531,.T.);
#3264=ORIENTED_EDGE('',*,*,#2532,.T.);
#3265=ORIENTED_EDGE('',*,*,#2533,.T.);
#3266=ORIENTED_EDGE('',*,*,#2534,.T.);
#3267=ORIENTED_EDGE('',*,*,#2532,.F.);
#3268=ORIENTED_EDGE('',*,*,#2535,.T.);
#3269=ORIENTED_EDGE('',*,*,#2536,.T.);
#3270=ORIENTED_EDGE('',*,*,#2537,.F.);
#3271=ORIENTED_EDGE('',*,*,#2538,.T.);
#3272=ORIENTED_EDGE('',*,*,#2539,.T.);
#3273=ORIENTED_EDGE('',*,*,#2540,.T.);
#3274=ORIENTED_EDGE('',*,*,#2541,.T.);
#3275=ORIENTED_EDGE('',*,*,#2539,.F.);
#3276=ORIENTED_EDGE('',*,*,#2542,.F.);
#3277=ORIENTED_EDGE('',*,*,#2543,.F.);
#3278=ORIENTED_EDGE('',*,*,#2544,.F.);
#3279=ORIENTED_EDGE('',*,*,#2545,.T.);
#3280=ORIENTED_EDGE('',*,*,#2546,.T.);
#3281=ORIENTED_EDGE('',*,*,#2547,.T.);
#3282=ORIENTED_EDGE('',*,*,#2548,.T.);
#3283=ORIENTED_EDGE('',*,*,#2546,.F.);
#3284=ORIENTED_EDGE('',*,*,#2549,.T.);
#3285=ORIENTED_EDGE('',*,*,#2550,.T.);
#3286=ORIENTED_EDGE('',*,*,#2551,.F.);
#3287=ORIENTED_EDGE('',*,*,#2552,.T.);
#3288=ORIENTED_EDGE('',*,*,#2553,.T.);
#3289=ORIENTED_EDGE('',*,*,#2554,.T.);
#3290=ORIENTED_EDGE('',*,*,#2555,.T.);
#3291=ORIENTED_EDGE('',*,*,#2553,.F.);
#3292=ORIENTED_EDGE('',*,*,#2556,.F.);
#3293=ORIENTED_EDGE('',*,*,#2557,.F.);
#3294=ORIENTED_EDGE('',*,*,#2558,.F.);
#3295=ORIENTED_EDGE('',*,*,#2559,.T.);
#3296=ORIENTED_EDGE('',*,*,#2560,.T.);
#3297=ORIENTED_EDGE('',*,*,#2561,.T.);
#3298=ORIENTED_EDGE('',*,*,#2562,.T.);
#3299=ORIENTED_EDGE('',*,*,#2560,.F.);
#3300=ORIENTED_EDGE('',*,*,#2563,.T.);
#3301=ORIENTED_EDGE('',*,*,#2564,.T.);
#3302=ORIENTED_EDGE('',*,*,#2565,.F.);
#3303=ORIENTED_EDGE('',*,*,#2566,.T.);
#3304=ORIENTED_EDGE('',*,*,#2567,.T.);
#3305=ORIENTED_EDGE('',*,*,#2568,.T.);
#3306=ORIENTED_EDGE('',*,*,#2569,.T.);
#3307=ORIENTED_EDGE('',*,*,#2567,.F.);
#3308=ORIENTED_EDGE('',*,*,#2570,.F.);
#3309=ORIENTED_EDGE('',*,*,#2571,.F.);
#3310=ORIENTED_EDGE('',*,*,#2572,.F.);
#3311=ORIENTED_EDGE('',*,*,#2573,.T.);
#3312=ORIENTED_EDGE('',*,*,#2574,.T.);
#3313=ORIENTED_EDGE('',*,*,#2575,.T.);
#3314=ORIENTED_EDGE('',*,*,#2576,.T.);
#3315=ORIENTED_EDGE('',*,*,#2574,.F.);
#3316=ORIENTED_EDGE('',*,*,#2577,.T.);
#3317=ORIENTED_EDGE('',*,*,#2578,.T.);
#3318=ORIENTED_EDGE('',*,*,#2579,.F.);
#3319=ORIENTED_EDGE('',*,*,#2580,.T.);
#3320=ORIENTED_EDGE('',*,*,#2581,.T.);
#3321=ORIENTED_EDGE('',*,*,#2582,.T.);
#3322=ORIENTED_EDGE('',*,*,#2583,.T.);
#3323=ORIENTED_EDGE('',*,*,#2581,.F.);
#3324=ORIENTED_EDGE('',*,*,#2584,.F.);
#3325=ORIENTED_EDGE('',*,*,#2585,.F.);
#3326=ORIENTED_EDGE('',*,*,#2586,.F.);
#3327=ORIENTED_EDGE('',*,*,#2587,.T.);
#3328=ORIENTED_EDGE('',*,*,#2588,.T.);
#3329=ORIENTED_EDGE('',*,*,#2589,.T.);
#3330=ORIENTED_EDGE('',*,*,#2590,.T.);
#3331=ORIENTED_EDGE('',*,*,#2588,.F.);
#3332=ORIENTED_EDGE('',*,*,#2591,.T.);
#3333=ORIENTED_EDGE('',*,*,#2592,.T.);
#3334=ORIENTED_EDGE('',*,*,#2593,.F.);
#3335=ORIENTED_EDGE('',*,*,#2594,.F.);
#3336=ORIENTED_EDGE('',*,*,#2333,.T.);
#3337=ORIENTED_EDGE('',*,*,#2595,.F.);
#3338=ORIENTED_EDGE('',*,*,#2596,.F.);
#3339=ORIENTED_EDGE('',*,*,#2597,.T.);
#3340=ORIENTED_EDGE('',*,*,#2596,.T.);
#3341=ORIENTED_EDGE('',*,*,#2598,.F.);
#3342=ORIENTED_EDGE('',*,*,#2599,.F.);
#3343=ORIENTED_EDGE('',*,*,#2600,.T.);
#3344=ORIENTED_EDGE('',*,*,#2599,.T.);
#3345=ORIENTED_EDGE('',*,*,#2601,.F.);
#3346=ORIENTED_EDGE('',*,*,#2340,.F.);
#3347=ORIENTED_EDGE('',*,*,#2602,.F.);
#3348=ORIENTED_EDGE('',*,*,#2347,.T.);
#3349=ORIENTED_EDGE('',*,*,#2603,.F.);
#3350=ORIENTED_EDGE('',*,*,#2604,.F.);
#3351=ORIENTED_EDGE('',*,*,#2605,.T.);
#3352=ORIENTED_EDGE('',*,*,#2604,.T.);
#3353=ORIENTED_EDGE('',*,*,#2606,.F.);
#3354=ORIENTED_EDGE('',*,*,#2607,.F.);
#3355=ORIENTED_EDGE('',*,*,#2608,.T.);
#3356=ORIENTED_EDGE('',*,*,#2607,.T.);
#3357=ORIENTED_EDGE('',*,*,#2609,.F.);
#3358=ORIENTED_EDGE('',*,*,#2354,.F.);
#3359=ORIENTED_EDGE('',*,*,#2610,.F.);
#3360=ORIENTED_EDGE('',*,*,#2361,.T.);
#3361=ORIENTED_EDGE('',*,*,#2611,.F.);
#3362=ORIENTED_EDGE('',*,*,#2612,.F.);
#3363=ORIENTED_EDGE('',*,*,#2613,.T.);
#3364=ORIENTED_EDGE('',*,*,#2612,.T.);
#3365=ORIENTED_EDGE('',*,*,#2614,.F.);
#3366=ORIENTED_EDGE('',*,*,#2615,.F.);
#3367=ORIENTED_EDGE('',*,*,#2616,.T.);
#3368=ORIENTED_EDGE('',*,*,#2615,.T.);
#3369=ORIENTED_EDGE('',*,*,#2617,.F.);
#3370=ORIENTED_EDGE('',*,*,#2368,.F.);
#3371=ORIENTED_EDGE('',*,*,#2618,.F.);
#3372=ORIENTED_EDGE('',*,*,#2375,.T.);
#3373=ORIENTED_EDGE('',*,*,#2619,.F.);
#3374=ORIENTED_EDGE('',*,*,#2620,.F.);
#3375=ORIENTED_EDGE('',*,*,#2621,.T.);
#3376=ORIENTED_EDGE('',*,*,#2620,.T.);
#3377=ORIENTED_EDGE('',*,*,#2622,.F.);
#3378=ORIENTED_EDGE('',*,*,#2623,.F.);
#3379=ORIENTED_EDGE('',*,*,#2624,.T.);
#3380=ORIENTED_EDGE('',*,*,#2623,.T.);
#3381=ORIENTED_EDGE('',*,*,#2625,.F.);
#3382=ORIENTED_EDGE('',*,*,#2382,.F.);
#3383=ORIENTED_EDGE('',*,*,#2626,.F.);
#3384=ORIENTED_EDGE('',*,*,#2389,.T.);
#3385=ORIENTED_EDGE('',*,*,#2627,.F.);
#3386=ORIENTED_EDGE('',*,*,#2628,.F.);
#3387=ORIENTED_EDGE('',*,*,#2629,.T.);
#3388=ORIENTED_EDGE('',*,*,#2628,.T.);
#3389=ORIENTED_EDGE('',*,*,#2630,.F.);
#3390=ORIENTED_EDGE('',*,*,#2631,.F.);
#3391=ORIENTED_EDGE('',*,*,#2632,.T.);
#3392=ORIENTED_EDGE('',*,*,#2631,.T.);
#3393=ORIENTED_EDGE('',*,*,#2633,.F.);
#3394=ORIENTED_EDGE('',*,*,#2396,.F.);
#3395=ORIENTED_EDGE('',*,*,#2634,.F.);
#3396=ORIENTED_EDGE('',*,*,#2403,.T.);
#3397=ORIENTED_EDGE('',*,*,#2635,.F.);
#3398=ORIENTED_EDGE('',*,*,#2636,.F.);
#3399=ORIENTED_EDGE('',*,*,#2637,.T.);
#3400=ORIENTED_EDGE('',*,*,#2636,.T.);
#3401=ORIENTED_EDGE('',*,*,#2638,.F.);
#3402=ORIENTED_EDGE('',*,*,#2639,.F.);
#3403=ORIENTED_EDGE('',*,*,#2640,.T.);
#3404=ORIENTED_EDGE('',*,*,#2639,.T.);
#3405=ORIENTED_EDGE('',*,*,#2641,.F.);
#3406=ORIENTED_EDGE('',*,*,#2410,.F.);
#3407=ORIENTED_EDGE('',*,*,#2642,.F.);
#3408=ORIENTED_EDGE('',*,*,#2417,.T.);
#3409=ORIENTED_EDGE('',*,*,#2643,.F.);
#3410=ORIENTED_EDGE('',*,*,#2644,.F.);
#3411=ORIENTED_EDGE('',*,*,#2645,.T.);
#3412=ORIENTED_EDGE('',*,*,#2644,.T.);
#3413=ORIENTED_EDGE('',*,*,#2646,.F.);
#3414=ORIENTED_EDGE('',*,*,#2647,.F.);
#3415=ORIENTED_EDGE('',*,*,#2648,.T.);
#3416=ORIENTED_EDGE('',*,*,#2647,.T.);
#3417=ORIENTED_EDGE('',*,*,#2649,.F.);
#3418=ORIENTED_EDGE('',*,*,#2424,.F.);
#3419=ORIENTED_EDGE('',*,*,#2650,.F.);
#3420=ORIENTED_EDGE('',*,*,#2431,.T.);
#3421=ORIENTED_EDGE('',*,*,#2651,.F.);
#3422=ORIENTED_EDGE('',*,*,#2652,.F.);
#3423=ORIENTED_EDGE('',*,*,#2653,.T.);
#3424=ORIENTED_EDGE('',*,*,#2652,.T.);
#3425=ORIENTED_EDGE('',*,*,#2654,.F.);
#3426=ORIENTED_EDGE('',*,*,#2655,.F.);
#3427=ORIENTED_EDGE('',*,*,#2656,.T.);
#3428=ORIENTED_EDGE('',*,*,#2655,.T.);
#3429=ORIENTED_EDGE('',*,*,#2657,.F.);
#3430=ORIENTED_EDGE('',*,*,#2438,.F.);
#3431=ORIENTED_EDGE('',*,*,#2658,.F.);
#3432=ORIENTED_EDGE('',*,*,#2445,.T.);
#3433=ORIENTED_EDGE('',*,*,#2659,.F.);
#3434=ORIENTED_EDGE('',*,*,#2660,.F.);
#3435=ORIENTED_EDGE('',*,*,#2661,.T.);
#3436=ORIENTED_EDGE('',*,*,#2660,.T.);
#3437=ORIENTED_EDGE('',*,*,#2662,.F.);
#3438=ORIENTED_EDGE('',*,*,#2663,.F.);
#3439=ORIENTED_EDGE('',*,*,#2664,.T.);
#3440=ORIENTED_EDGE('',*,*,#2663,.T.);
#3441=ORIENTED_EDGE('',*,*,#2665,.F.);
#3442=ORIENTED_EDGE('',*,*,#2452,.F.);
#3443=ORIENTED_EDGE('',*,*,#2666,.F.);
#3444=ORIENTED_EDGE('',*,*,#2459,.T.);
#3445=ORIENTED_EDGE('',*,*,#2667,.F.);
#3446=ORIENTED_EDGE('',*,*,#2668,.F.);
#3447=ORIENTED_EDGE('',*,*,#2669,.T.);
#3448=ORIENTED_EDGE('',*,*,#2668,.T.);
#3449=ORIENTED_EDGE('',*,*,#2670,.F.);
#3450=ORIENTED_EDGE('',*,*,#2671,.F.);
#3451=ORIENTED_EDGE('',*,*,#2672,.T.);
#3452=ORIENTED_EDGE('',*,*,#2671,.T.);
#3453=ORIENTED_EDGE('',*,*,#2673,.F.);
#3454=ORIENTED_EDGE('',*,*,#2466,.F.);
#3455=ORIENTED_EDGE('',*,*,#2674,.F.);
#3456=ORIENTED_EDGE('',*,*,#2473,.T.);
#3457=ORIENTED_EDGE('',*,*,#2675,.F.);
#3458=ORIENTED_EDGE('',*,*,#2676,.F.);
#3459=ORIENTED_EDGE('',*,*,#2677,.T.);
#3460=ORIENTED_EDGE('',*,*,#2676,.T.);
#3461=ORIENTED_EDGE('',*,*,#2678,.F.);
#3462=ORIENTED_EDGE('',*,*,#2679,.F.);
#3463=ORIENTED_EDGE('',*,*,#2680,.T.);
#3464=ORIENTED_EDGE('',*,*,#2679,.T.);
#3465=ORIENTED_EDGE('',*,*,#2681,.F.);
#3466=ORIENTED_EDGE('',*,*,#2480,.F.);
#3467=ORIENTED_EDGE('',*,*,#2682,.F.);
#3468=ORIENTED_EDGE('',*,*,#2487,.T.);
#3469=ORIENTED_EDGE('',*,*,#2683,.F.);
#3470=ORIENTED_EDGE('',*,*,#2684,.F.);
#3471=ORIENTED_EDGE('',*,*,#2685,.T.);
#3472=ORIENTED_EDGE('',*,*,#2684,.T.);
#3473=ORIENTED_EDGE('',*,*,#2686,.F.);
#3474=ORIENTED_EDGE('',*,*,#2687,.F.);
#3475=ORIENTED_EDGE('',*,*,#2688,.T.);
#3476=ORIENTED_EDGE('',*,*,#2687,.T.);
#3477=ORIENTED_EDGE('',*,*,#2689,.F.);
#3478=ORIENTED_EDGE('',*,*,#2494,.F.);
#3479=ORIENTED_EDGE('',*,*,#2690,.F.);
#3480=ORIENTED_EDGE('',*,*,#2501,.T.);
#3481=ORIENTED_EDGE('',*,*,#2691,.F.);
#3482=ORIENTED_EDGE('',*,*,#2692,.F.);
#3483=ORIENTED_EDGE('',*,*,#2693,.T.);
#3484=ORIENTED_EDGE('',*,*,#2692,.T.);
#3485=ORIENTED_EDGE('',*,*,#2694,.F.);
#3486=ORIENTED_EDGE('',*,*,#2695,.F.);
#3487=ORIENTED_EDGE('',*,*,#2696,.T.);
#3488=ORIENTED_EDGE('',*,*,#2695,.T.);
#3489=ORIENTED_EDGE('',*,*,#2697,.F.);
#3490=ORIENTED_EDGE('',*,*,#2508,.F.);
#3491=ORIENTED_EDGE('',*,*,#2698,.F.);
#3492=ORIENTED_EDGE('',*,*,#2515,.T.);
#3493=ORIENTED_EDGE('',*,*,#2699,.F.);
#3494=ORIENTED_EDGE('',*,*,#2700,.F.);
#3495=ORIENTED_EDGE('',*,*,#2701,.T.);
#3496=ORIENTED_EDGE('',*,*,#2700,.T.);
#3497=ORIENTED_EDGE('',*,*,#2702,.F.);
#3498=ORIENTED_EDGE('',*,*,#2703,.F.);
#3499=ORIENTED_EDGE('',*,*,#2704,.T.);
#3500=ORIENTED_EDGE('',*,*,#2703,.T.);
#3501=ORIENTED_EDGE('',*,*,#2705,.F.);
#3502=ORIENTED_EDGE('',*,*,#2522,.F.);
#3503=ORIENTED_EDGE('',*,*,#2706,.F.);
#3504=ORIENTED_EDGE('',*,*,#2529,.T.);
#3505=ORIENTED_EDGE('',*,*,#2707,.F.);
#3506=ORIENTED_EDGE('',*,*,#2708,.F.);
#3507=ORIENTED_EDGE('',*,*,#2709,.T.);
#3508=ORIENTED_EDGE('',*,*,#2708,.T.);
#3509=ORIENTED_EDGE('',*,*,#2710,.F.);
#3510=ORIENTED_EDGE('',*,*,#2711,.F.);
#3511=ORIENTED_EDGE('',*,*,#2712,.T.);
#3512=ORIENTED_EDGE('',*,*,#2711,.T.);
#3513=ORIENTED_EDGE('',*,*,#2713,.F.);
#3514=ORIENTED_EDGE('',*,*,#2536,.F.);
#3515=ORIENTED_EDGE('',*,*,#2714,.F.);
#3516=ORIENTED_EDGE('',*,*,#2543,.T.);
#3517=ORIENTED_EDGE('',*,*,#2715,.F.);
#3518=ORIENTED_EDGE('',*,*,#2716,.F.);
#3519=ORIENTED_EDGE('',*,*,#2717,.T.);
#3520=ORIENTED_EDGE('',*,*,#2716,.T.);
#3521=ORIENTED_EDGE('',*,*,#2718,.F.);
#3522=ORIENTED_EDGE('',*,*,#2719,.F.);
#3523=ORIENTED_EDGE('',*,*,#2720,.T.);
#3524=ORIENTED_EDGE('',*,*,#2719,.T.);
#3525=ORIENTED_EDGE('',*,*,#2721,.F.);
#3526=ORIENTED_EDGE('',*,*,#2550,.F.);
#3527=ORIENTED_EDGE('',*,*,#2722,.F.);
#3528=ORIENTED_EDGE('',*,*,#2557,.T.);
#3529=ORIENTED_EDGE('',*,*,#2723,.F.);
#3530=ORIENTED_EDGE('',*,*,#2724,.F.);
#3531=ORIENTED_EDGE('',*,*,#2725,.T.);
#3532=ORIENTED_EDGE('',*,*,#2724,.T.);
#3533=ORIENTED_EDGE('',*,*,#2726,.F.);
#3534=ORIENTED_EDGE('',*,*,#2727,.F.);
#3535=ORIENTED_EDGE('',*,*,#2728,.T.);
#3536=ORIENTED_EDGE('',*,*,#2727,.T.);
#3537=ORIENTED_EDGE('',*,*,#2729,.F.);
#3538=ORIENTED_EDGE('',*,*,#2564,.F.);
#3539=ORIENTED_EDGE('',*,*,#2730,.F.);
#3540=ORIENTED_EDGE('',*,*,#2571,.T.);
#3541=ORIENTED_EDGE('',*,*,#2731,.F.);
#3542=ORIENTED_EDGE('',*,*,#2732,.F.);
#3543=ORIENTED_EDGE('',*,*,#2733,.T.);
#3544=ORIENTED_EDGE('',*,*,#2732,.T.);
#3545=ORIENTED_EDGE('',*,*,#2734,.F.);
#3546=ORIENTED_EDGE('',*,*,#2735,.F.);
#3547=ORIENTED_EDGE('',*,*,#2736,.T.);
#3548=ORIENTED_EDGE('',*,*,#2735,.T.);
#3549=ORIENTED_EDGE('',*,*,#2737,.F.);
#3550=ORIENTED_EDGE('',*,*,#2578,.F.);
#3551=ORIENTED_EDGE('',*,*,#2738,.F.);
#3552=ORIENTED_EDGE('',*,*,#2585,.T.);
#3553=ORIENTED_EDGE('',*,*,#2739,.F.);
#3554=ORIENTED_EDGE('',*,*,#2740,.F.);
#3555=ORIENTED_EDGE('',*,*,#2741,.T.);
#3556=ORIENTED_EDGE('',*,*,#2740,.T.);
#3557=ORIENTED_EDGE('',*,*,#2742,.F.);
#3558=ORIENTED_EDGE('',*,*,#2743,.F.);
#3559=ORIENTED_EDGE('',*,*,#2744,.T.);
#3560=ORIENTED_EDGE('',*,*,#2743,.T.);
#3561=ORIENTED_EDGE('',*,*,#2745,.F.);
#3562=ORIENTED_EDGE('',*,*,#2592,.F.);
#3563=ORIENTED_EDGE('',*,*,#2344,.F.);
#3564=ORIENTED_EDGE('',*,*,#2348,.T.);
#3565=ORIENTED_EDGE('',*,*,#2602,.T.);
#3566=ORIENTED_EDGE('',*,*,#2605,.F.);
#3567=ORIENTED_EDGE('',*,*,#2608,.F.);
#3568=ORIENTED_EDGE('',*,*,#2353,.F.);
#3569=ORIENTED_EDGE('',*,*,#2349,.F.);
#3570=ORIENTED_EDGE('',*,*,#2746,.F.);
#3571=ORIENTED_EDGE('',*,*,#2358,.F.);
#3572=ORIENTED_EDGE('',*,*,#2362,.T.);
#3573=ORIENTED_EDGE('',*,*,#2610,.T.);
#3574=ORIENTED_EDGE('',*,*,#2613,.F.);
#3575=ORIENTED_EDGE('',*,*,#2616,.F.);
#3576=ORIENTED_EDGE('',*,*,#2367,.F.);
#3577=ORIENTED_EDGE('',*,*,#2363,.F.);
#3578=ORIENTED_EDGE('',*,*,#2747,.F.);
#3579=ORIENTED_EDGE('',*,*,#2372,.F.);
#3580=ORIENTED_EDGE('',*,*,#2376,.T.);
#3581=ORIENTED_EDGE('',*,*,#2618,.T.);
#3582=ORIENTED_EDGE('',*,*,#2621,.F.);
#3583=ORIENTED_EDGE('',*,*,#2624,.F.);
#3584=ORIENTED_EDGE('',*,*,#2381,.F.);
#3585=ORIENTED_EDGE('',*,*,#2377,.F.);
#3586=ORIENTED_EDGE('',*,*,#2748,.F.);
#3587=ORIENTED_EDGE('',*,*,#2386,.F.);
#3588=ORIENTED_EDGE('',*,*,#2390,.T.);
#3589=ORIENTED_EDGE('',*,*,#2626,.T.);
#3590=ORIENTED_EDGE('',*,*,#2629,.F.);
#3591=ORIENTED_EDGE('',*,*,#2632,.F.);
#3592=ORIENTED_EDGE('',*,*,#2395,.F.);
#3593=ORIENTED_EDGE('',*,*,#2391,.F.);
#3594=ORIENTED_EDGE('',*,*,#2749,.F.);
#3595=ORIENTED_EDGE('',*,*,#2400,.F.);
#3596=ORIENTED_EDGE('',*,*,#2404,.T.);
#3597=ORIENTED_EDGE('',*,*,#2634,.T.);
#3598=ORIENTED_EDGE('',*,*,#2637,.F.);
#3599=ORIENTED_EDGE('',*,*,#2640,.F.);
#3600=ORIENTED_EDGE('',*,*,#2409,.F.);
#3601=ORIENTED_EDGE('',*,*,#2405,.F.);
#3602=ORIENTED_EDGE('',*,*,#2750,.F.);
#3603=ORIENTED_EDGE('',*,*,#2414,.F.);
#3604=ORIENTED_EDGE('',*,*,#2418,.T.);
#3605=ORIENTED_EDGE('',*,*,#2642,.T.);
#3606=ORIENTED_EDGE('',*,*,#2645,.F.);
#3607=ORIENTED_EDGE('',*,*,#2648,.F.);
#3608=ORIENTED_EDGE('',*,*,#2423,.F.);
#3609=ORIENTED_EDGE('',*,*,#2419,.F.);
#3610=ORIENTED_EDGE('',*,*,#2751,.F.);
#3611=ORIENTED_EDGE('',*,*,#2428,.F.);
#3612=ORIENTED_EDGE('',*,*,#2432,.T.);
#3613=ORIENTED_EDGE('',*,*,#2650,.T.);
#3614=ORIENTED_EDGE('',*,*,#2653,.F.);
#3615=ORIENTED_EDGE('',*,*,#2656,.F.);
#3616=ORIENTED_EDGE('',*,*,#2437,.F.);
#3617=ORIENTED_EDGE('',*,*,#2433,.F.);
#3618=ORIENTED_EDGE('',*,*,#2752,.F.);
#3619=ORIENTED_EDGE('',*,*,#2442,.F.);
#3620=ORIENTED_EDGE('',*,*,#2446,.T.);
#3621=ORIENTED_EDGE('',*,*,#2658,.T.);
#3622=ORIENTED_EDGE('',*,*,#2661,.F.);
#3623=ORIENTED_EDGE('',*,*,#2664,.F.);
#3624=ORIENTED_EDGE('',*,*,#2451,.F.);
#3625=ORIENTED_EDGE('',*,*,#2447,.F.);
#3626=ORIENTED_EDGE('',*,*,#2753,.F.);
#3627=ORIENTED_EDGE('',*,*,#2456,.F.);
#3628=ORIENTED_EDGE('',*,*,#2460,.T.);
#3629=ORIENTED_EDGE('',*,*,#2666,.T.);
#3630=ORIENTED_EDGE('',*,*,#2669,.F.);
#3631=ORIENTED_EDGE('',*,*,#2672,.F.);
#3632=ORIENTED_EDGE('',*,*,#2465,.F.);
#3633=ORIENTED_EDGE('',*,*,#2461,.F.);
#3634=ORIENTED_EDGE('',*,*,#2754,.F.);
#3635=ORIENTED_EDGE('',*,*,#2470,.F.);
#3636=ORIENTED_EDGE('',*,*,#2474,.T.);
#3637=ORIENTED_EDGE('',*,*,#2674,.T.);
#3638=ORIENTED_EDGE('',*,*,#2677,.F.);
#3639=ORIENTED_EDGE('',*,*,#2680,.F.);
#3640=ORIENTED_EDGE('',*,*,#2479,.F.);
#3641=ORIENTED_EDGE('',*,*,#2475,.F.);
#3642=ORIENTED_EDGE('',*,*,#2755,.F.);
#3643=ORIENTED_EDGE('',*,*,#2484,.F.);
#3644=ORIENTED_EDGE('',*,*,#2488,.T.);
#3645=ORIENTED_EDGE('',*,*,#2682,.T.);
#3646=ORIENTED_EDGE('',*,*,#2685,.F.);
#3647=ORIENTED_EDGE('',*,*,#2688,.F.);
#3648=ORIENTED_EDGE('',*,*,#2493,.F.);
#3649=ORIENTED_EDGE('',*,*,#2489,.F.);
#3650=ORIENTED_EDGE('',*,*,#2756,.F.);
#3651=ORIENTED_EDGE('',*,*,#2498,.F.);
#3652=ORIENTED_EDGE('',*,*,#2502,.T.);
#3653=ORIENTED_EDGE('',*,*,#2690,.T.);
#3654=ORIENTED_EDGE('',*,*,#2693,.F.);
#3655=ORIENTED_EDGE('',*,*,#2696,.F.);
#3656=ORIENTED_EDGE('',*,*,#2507,.F.);
#3657=ORIENTED_EDGE('',*,*,#2503,.F.);
#3658=ORIENTED_EDGE('',*,*,#2757,.F.);
#3659=ORIENTED_EDGE('',*,*,#2512,.F.);
#3660=ORIENTED_EDGE('',*,*,#2516,.T.);
#3661=ORIENTED_EDGE('',*,*,#2698,.T.);
#3662=ORIENTED_EDGE('',*,*,#2701,.F.);
#3663=ORIENTED_EDGE('',*,*,#2704,.F.);
#3664=ORIENTED_EDGE('',*,*,#2521,.F.);
#3665=ORIENTED_EDGE('',*,*,#2517,.F.);
#3666=ORIENTED_EDGE('',*,*,#2758,.F.);
#3667=ORIENTED_EDGE('',*,*,#2526,.F.);
#3668=ORIENTED_EDGE('',*,*,#2530,.T.);
#3669=ORIENTED_EDGE('',*,*,#2706,.T.);
#3670=ORIENTED_EDGE('',*,*,#2709,.F.);
#3671=ORIENTED_EDGE('',*,*,#2712,.F.);
#3672=ORIENTED_EDGE('',*,*,#2535,.F.);
#3673=ORIENTED_EDGE('',*,*,#2531,.F.);
#3674=ORIENTED_EDGE('',*,*,#2759,.F.);
#3675=ORIENTED_EDGE('',*,*,#2540,.F.);
#3676=ORIENTED_EDGE('',*,*,#2544,.T.);
#3677=ORIENTED_EDGE('',*,*,#2714,.T.);
#3678=ORIENTED_EDGE('',*,*,#2717,.F.);
#3679=ORIENTED_EDGE('',*,*,#2720,.F.);
#3680=ORIENTED_EDGE('',*,*,#2549,.F.);
#3681=ORIENTED_EDGE('',*,*,#2545,.F.);
#3682=ORIENTED_EDGE('',*,*,#2760,.F.);
#3683=ORIENTED_EDGE('',*,*,#2554,.F.);
#3684=ORIENTED_EDGE('',*,*,#2558,.T.);
#3685=ORIENTED_EDGE('',*,*,#2722,.T.);
#3686=ORIENTED_EDGE('',*,*,#2725,.F.);
#3687=ORIENTED_EDGE('',*,*,#2728,.F.);
#3688=ORIENTED_EDGE('',*,*,#2563,.F.);
#3689=ORIENTED_EDGE('',*,*,#2559,.F.);
#3690=ORIENTED_EDGE('',*,*,#2761,.F.);
#3691=ORIENTED_EDGE('',*,*,#2568,.F.);
#3692=ORIENTED_EDGE('',*,*,#2572,.T.);
#3693=ORIENTED_EDGE('',*,*,#2730,.T.);
#3694=ORIENTED_EDGE('',*,*,#2733,.F.);
#3695=ORIENTED_EDGE('',*,*,#2736,.F.);
#3696=ORIENTED_EDGE('',*,*,#2577,.F.);
#3697=ORIENTED_EDGE('',*,*,#2573,.F.);
#3698=ORIENTED_EDGE('',*,*,#2762,.F.);
#3699=ORIENTED_EDGE('',*,*,#2582,.F.);
#3700=ORIENTED_EDGE('',*,*,#2586,.T.);
#3701=ORIENTED_EDGE('',*,*,#2738,.T.);
#3702=ORIENTED_EDGE('',*,*,#2741,.F.);
#3703=ORIENTED_EDGE('',*,*,#2744,.F.);
#3704=ORIENTED_EDGE('',*,*,#2591,.F.);
#3705=ORIENTED_EDGE('',*,*,#2587,.F.);
#3706=ORIENTED_EDGE('',*,*,#2763,.F.);
#3707=ORIENTED_EDGE('',*,*,#2764,.F.);
#3708=ORIENTED_EDGE('',*,*,#2765,.T.);
#3709=ORIENTED_EDGE('',*,*,#2766,.T.);
#3710=ORIENTED_EDGE('',*,*,#2767,.F.);
#3711=ORIENTED_EDGE('',*,*,#2768,.F.);
#3712=ORIENTED_EDGE('',*,*,#2769,.F.);
#3713=ORIENTED_EDGE('',*,*,#2770,.F.);
#3714=ORIENTED_EDGE('',*,*,#2771,.F.);
#3715=ORIENTED_EDGE('',*,*,#2330,.F.);
#3716=ORIENTED_EDGE('',*,*,#2334,.T.);
#3717=ORIENTED_EDGE('',*,*,#2594,.T.);
#3718=ORIENTED_EDGE('',*,*,#2597,.F.);
#3719=ORIENTED_EDGE('',*,*,#2600,.F.);
#3720=ORIENTED_EDGE('',*,*,#2339,.F.);
#3721=ORIENTED_EDGE('',*,*,#2335,.F.);
#3722=ORIENTED_EDGE('',*,*,#2772,.F.);
#3723=ORIENTED_EDGE('',*,*,#2327,.T.);
#3724=ORIENTED_EDGE('',*,*,#2773,.T.);
#3725=ORIENTED_EDGE('',*,*,#2774,.F.);
#3726=ORIENTED_EDGE('',*,*,#2775,.T.);
#3727=ORIENTED_EDGE('',*,*,#2776,.T.);
#3728=ORIENTED_EDGE('',*,*,#2777,.T.);
#3729=ORIENTED_EDGE('',*,*,#2778,.T.);
#3730=ORIENTED_EDGE('',*,*,#2779,.T.);
#3731=ORIENTED_EDGE('',*,*,#2780,.F.);
#3732=ORIENTED_EDGE('',*,*,#2781,.T.);
#3733=ORIENTED_EDGE('',*,*,#2589,.F.);
#3734=ORIENTED_EDGE('',*,*,#2593,.T.);
#3735=ORIENTED_EDGE('',*,*,#2745,.T.);
#3736=ORIENTED_EDGE('',*,*,#2742,.T.);
#3737=ORIENTED_EDGE('',*,*,#2739,.T.);
#3738=ORIENTED_EDGE('',*,*,#2584,.T.);
#3739=ORIENTED_EDGE('',*,*,#2580,.F.);
#3740=ORIENTED_EDGE('',*,*,#2782,.T.);
#3741=ORIENTED_EDGE('',*,*,#2575,.F.);
#3742=ORIENTED_EDGE('',*,*,#2579,.T.);
#3743=ORIENTED_EDGE('',*,*,#2737,.T.);
#3744=ORIENTED_EDGE('',*,*,#2734,.T.);
#3745=ORIENTED_EDGE('',*,*,#2731,.T.);
#3746=ORIENTED_EDGE('',*,*,#2570,.T.);
#3747=ORIENTED_EDGE('',*,*,#2566,.F.);
#3748=ORIENTED_EDGE('',*,*,#2783,.T.);
#3749=ORIENTED_EDGE('',*,*,#2561,.F.);
#3750=ORIENTED_EDGE('',*,*,#2565,.T.);
#3751=ORIENTED_EDGE('',*,*,#2729,.T.);
#3752=ORIENTED_EDGE('',*,*,#2726,.T.);
#3753=ORIENTED_EDGE('',*,*,#2723,.T.);
#3754=ORIENTED_EDGE('',*,*,#2556,.T.);
#3755=ORIENTED_EDGE('',*,*,#2552,.F.);
#3756=ORIENTED_EDGE('',*,*,#2784,.T.);
#3757=ORIENTED_EDGE('',*,*,#2547,.F.);
#3758=ORIENTED_EDGE('',*,*,#2551,.T.);
#3759=ORIENTED_EDGE('',*,*,#2721,.T.);
#3760=ORIENTED_EDGE('',*,*,#2718,.T.);
#3761=ORIENTED_EDGE('',*,*,#2715,.T.);
#3762=ORIENTED_EDGE('',*,*,#2542,.T.);
#3763=ORIENTED_EDGE('',*,*,#2538,.F.);
#3764=ORIENTED_EDGE('',*,*,#2785,.T.);
#3765=ORIENTED_EDGE('',*,*,#2533,.F.);
#3766=ORIENTED_EDGE('',*,*,#2537,.T.);
#3767=ORIENTED_EDGE('',*,*,#2713,.T.);
#3768=ORIENTED_EDGE('',*,*,#2710,.T.);
#3769=ORIENTED_EDGE('',*,*,#2707,.T.);
#3770=ORIENTED_EDGE('',*,*,#2528,.T.);
#3771=ORIENTED_EDGE('',*,*,#2524,.F.);
#3772=ORIENTED_EDGE('',*,*,#2786,.T.);
#3773=ORIENTED_EDGE('',*,*,#2519,.F.);
#3774=ORIENTED_EDGE('',*,*,#2523,.T.);
#3775=ORIENTED_EDGE('',*,*,#2705,.T.);
#3776=ORIENTED_EDGE('',*,*,#2702,.T.);
#3777=ORIENTED_EDGE('',*,*,#2699,.T.);
#3778=ORIENTED_EDGE('',*,*,#2514,.T.);
#3779=ORIENTED_EDGE('',*,*,#2510,.F.);
#3780=ORIENTED_EDGE('',*,*,#2787,.T.);
#3781=ORIENTED_EDGE('',*,*,#2505,.F.);
#3782=ORIENTED_EDGE('',*,*,#2509,.T.);
#3783=ORIENTED_EDGE('',*,*,#2697,.T.);
#3784=ORIENTED_EDGE('',*,*,#2694,.T.);
#3785=ORIENTED_EDGE('',*,*,#2691,.T.);
#3786=ORIENTED_EDGE('',*,*,#2500,.T.);
#3787=ORIENTED_EDGE('',*,*,#2496,.F.);
#3788=ORIENTED_EDGE('',*,*,#2788,.T.);
#3789=ORIENTED_EDGE('',*,*,#2491,.F.);
#3790=ORIENTED_EDGE('',*,*,#2495,.T.);
#3791=ORIENTED_EDGE('',*,*,#2689,.T.);
#3792=ORIENTED_EDGE('',*,*,#2686,.T.);
#3793=ORIENTED_EDGE('',*,*,#2683,.T.);
#3794=ORIENTED_EDGE('',*,*,#2486,.T.);
#3795=ORIENTED_EDGE('',*,*,#2482,.F.);
#3796=ORIENTED_EDGE('',*,*,#2789,.T.);
#3797=ORIENTED_EDGE('',*,*,#2477,.F.);
#3798=ORIENTED_EDGE('',*,*,#2481,.T.);
#3799=ORIENTED_EDGE('',*,*,#2681,.T.);
#3800=ORIENTED_EDGE('',*,*,#2678,.T.);
#3801=ORIENTED_EDGE('',*,*,#2675,.T.);
#3802=ORIENTED_EDGE('',*,*,#2472,.T.);
#3803=ORIENTED_EDGE('',*,*,#2468,.F.);
#3804=ORIENTED_EDGE('',*,*,#2790,.T.);
#3805=ORIENTED_EDGE('',*,*,#2463,.F.);
#3806=ORIENTED_EDGE('',*,*,#2467,.T.);
#3807=ORIENTED_EDGE('',*,*,#2673,.T.);
#3808=ORIENTED_EDGE('',*,*,#2670,.T.);
#3809=ORIENTED_EDGE('',*,*,#2667,.T.);
#3810=ORIENTED_EDGE('',*,*,#2458,.T.);
#3811=ORIENTED_EDGE('',*,*,#2454,.F.);
#3812=ORIENTED_EDGE('',*,*,#2791,.T.);
#3813=ORIENTED_EDGE('',*,*,#2449,.F.);
#3814=ORIENTED_EDGE('',*,*,#2453,.T.);
#3815=ORIENTED_EDGE('',*,*,#2665,.T.);
#3816=ORIENTED_EDGE('',*,*,#2662,.T.);
#3817=ORIENTED_EDGE('',*,*,#2659,.T.);
#3818=ORIENTED_EDGE('',*,*,#2444,.T.);
#3819=ORIENTED_EDGE('',*,*,#2440,.F.);
#3820=ORIENTED_EDGE('',*,*,#2792,.T.);
#3821=ORIENTED_EDGE('',*,*,#2435,.F.);
#3822=ORIENTED_EDGE('',*,*,#2439,.T.);
#3823=ORIENTED_EDGE('',*,*,#2657,.T.);
#3824=ORIENTED_EDGE('',*,*,#2654,.T.);
#3825=ORIENTED_EDGE('',*,*,#2651,.T.);
#3826=ORIENTED_EDGE('',*,*,#2430,.T.);
#3827=ORIENTED_EDGE('',*,*,#2426,.F.);
#3828=ORIENTED_EDGE('',*,*,#2793,.T.);
#3829=ORIENTED_EDGE('',*,*,#2421,.F.);
#3830=ORIENTED_EDGE('',*,*,#2425,.T.);
#3831=ORIENTED_EDGE('',*,*,#2649,.T.);
#3832=ORIENTED_EDGE('',*,*,#2646,.T.);
#3833=ORIENTED_EDGE('',*,*,#2643,.T.);
#3834=ORIENTED_EDGE('',*,*,#2416,.T.);
#3835=ORIENTED_EDGE('',*,*,#2412,.F.);
#3836=ORIENTED_EDGE('',*,*,#2794,.T.);
#3837=ORIENTED_EDGE('',*,*,#2407,.F.);
#3838=ORIENTED_EDGE('',*,*,#2411,.T.);
#3839=ORIENTED_EDGE('',*,*,#2641,.T.);
#3840=ORIENTED_EDGE('',*,*,#2638,.T.);
#3841=ORIENTED_EDGE('',*,*,#2635,.T.);
#3842=ORIENTED_EDGE('',*,*,#2402,.T.);
#3843=ORIENTED_EDGE('',*,*,#2398,.F.);
#3844=ORIENTED_EDGE('',*,*,#2795,.T.);
#3845=ORIENTED_EDGE('',*,*,#2393,.F.);
#3846=ORIENTED_EDGE('',*,*,#2397,.T.);
#3847=ORIENTED_EDGE('',*,*,#2633,.T.);
#3848=ORIENTED_EDGE('',*,*,#2630,.T.);
#3849=ORIENTED_EDGE('',*,*,#2627,.T.);
#3850=ORIENTED_EDGE('',*,*,#2388,.T.);
#3851=ORIENTED_EDGE('',*,*,#2384,.F.);
#3852=ORIENTED_EDGE('',*,*,#2796,.T.);
#3853=ORIENTED_EDGE('',*,*,#2379,.F.);
#3854=ORIENTED_EDGE('',*,*,#2383,.T.);
#3855=ORIENTED_EDGE('',*,*,#2625,.T.);
#3856=ORIENTED_EDGE('',*,*,#2622,.T.);
#3857=ORIENTED_EDGE('',*,*,#2619,.T.);
#3858=ORIENTED_EDGE('',*,*,#2374,.T.);
#3859=ORIENTED_EDGE('',*,*,#2370,.F.);
#3860=ORIENTED_EDGE('',*,*,#2797,.T.);
#3861=ORIENTED_EDGE('',*,*,#2365,.F.);
#3862=ORIENTED_EDGE('',*,*,#2369,.T.);
#3863=ORIENTED_EDGE('',*,*,#2617,.T.);
#3864=ORIENTED_EDGE('',*,*,#2614,.T.);
#3865=ORIENTED_EDGE('',*,*,#2611,.T.);
#3866=ORIENTED_EDGE('',*,*,#2360,.T.);
#3867=ORIENTED_EDGE('',*,*,#2356,.F.);
#3868=ORIENTED_EDGE('',*,*,#2798,.T.);
#3869=ORIENTED_EDGE('',*,*,#2351,.F.);
#3870=ORIENTED_EDGE('',*,*,#2355,.T.);
#3871=ORIENTED_EDGE('',*,*,#2609,.T.);
#3872=ORIENTED_EDGE('',*,*,#2606,.T.);
#3873=ORIENTED_EDGE('',*,*,#2603,.T.);
#3874=ORIENTED_EDGE('',*,*,#2346,.T.);
#3875=ORIENTED_EDGE('',*,*,#2342,.F.);
#3876=ORIENTED_EDGE('',*,*,#2799,.T.);
#3877=ORIENTED_EDGE('',*,*,#2337,.F.);
#3878=ORIENTED_EDGE('',*,*,#2341,.T.);
#3879=ORIENTED_EDGE('',*,*,#2601,.T.);
#3880=ORIENTED_EDGE('',*,*,#2598,.T.);
#3881=ORIENTED_EDGE('',*,*,#2595,.T.);
#3882=ORIENTED_EDGE('',*,*,#2332,.T.);
#3883=ORIENTED_EDGE('',*,*,#2328,.F.);
#3884=ORIENTED_EDGE('',*,*,#2325,.T.);
#3885=ORIENTED_EDGE('',*,*,#2590,.F.);
#3886=ORIENTED_EDGE('',*,*,#2781,.F.);
#3887=ORIENTED_EDGE('',*,*,#2800,.F.);
#3888=ORIENTED_EDGE('',*,*,#2763,.T.);
#3889=ORIENTED_EDGE('',*,*,#2576,.F.);
#3890=ORIENTED_EDGE('',*,*,#2782,.F.);
#3891=ORIENTED_EDGE('',*,*,#2583,.F.);
#3892=ORIENTED_EDGE('',*,*,#2762,.T.);
#3893=ORIENTED_EDGE('',*,*,#2562,.F.);
#3894=ORIENTED_EDGE('',*,*,#2783,.F.);
#3895=ORIENTED_EDGE('',*,*,#2569,.F.);
#3896=ORIENTED_EDGE('',*,*,#2761,.T.);
#3897=ORIENTED_EDGE('',*,*,#2548,.F.);
#3898=ORIENTED_EDGE('',*,*,#2784,.F.);
#3899=ORIENTED_EDGE('',*,*,#2555,.F.);
#3900=ORIENTED_EDGE('',*,*,#2760,.T.);
#3901=ORIENTED_EDGE('',*,*,#2534,.F.);
#3902=ORIENTED_EDGE('',*,*,#2785,.F.);
#3903=ORIENTED_EDGE('',*,*,#2541,.F.);
#3904=ORIENTED_EDGE('',*,*,#2759,.T.);
#3905=ORIENTED_EDGE('',*,*,#2520,.F.);
#3906=ORIENTED_EDGE('',*,*,#2786,.F.);
#3907=ORIENTED_EDGE('',*,*,#2527,.F.);
#3908=ORIENTED_EDGE('',*,*,#2758,.T.);
#3909=ORIENTED_EDGE('',*,*,#2506,.F.);
#3910=ORIENTED_EDGE('',*,*,#2787,.F.);
#3911=ORIENTED_EDGE('',*,*,#2513,.F.);
#3912=ORIENTED_EDGE('',*,*,#2757,.T.);
#3913=ORIENTED_EDGE('',*,*,#2492,.F.);
#3914=ORIENTED_EDGE('',*,*,#2788,.F.);
#3915=ORIENTED_EDGE('',*,*,#2499,.F.);
#3916=ORIENTED_EDGE('',*,*,#2756,.T.);
#3917=ORIENTED_EDGE('',*,*,#2478,.F.);
#3918=ORIENTED_EDGE('',*,*,#2789,.F.);
#3919=ORIENTED_EDGE('',*,*,#2485,.F.);
#3920=ORIENTED_EDGE('',*,*,#2755,.T.);
#3921=ORIENTED_EDGE('',*,*,#2464,.F.);
#3922=ORIENTED_EDGE('',*,*,#2790,.F.);
#3923=ORIENTED_EDGE('',*,*,#2471,.F.);
#3924=ORIENTED_EDGE('',*,*,#2754,.T.);
#3925=ORIENTED_EDGE('',*,*,#2450,.F.);
#3926=ORIENTED_EDGE('',*,*,#2791,.F.);
#3927=ORIENTED_EDGE('',*,*,#2457,.F.);
#3928=ORIENTED_EDGE('',*,*,#2753,.T.);
#3929=ORIENTED_EDGE('',*,*,#2436,.F.);
#3930=ORIENTED_EDGE('',*,*,#2792,.F.);
#3931=ORIENTED_EDGE('',*,*,#2443,.F.);
#3932=ORIENTED_EDGE('',*,*,#2752,.T.);
#3933=ORIENTED_EDGE('',*,*,#2422,.F.);
#3934=ORIENTED_EDGE('',*,*,#2793,.F.);
#3935=ORIENTED_EDGE('',*,*,#2429,.F.);
#3936=ORIENTED_EDGE('',*,*,#2751,.T.);
#3937=ORIENTED_EDGE('',*,*,#2408,.F.);
#3938=ORIENTED_EDGE('',*,*,#2794,.F.);
#3939=ORIENTED_EDGE('',*,*,#2415,.F.);
#3940=ORIENTED_EDGE('',*,*,#2750,.T.);
#3941=ORIENTED_EDGE('',*,*,#2394,.F.);
#3942=ORIENTED_EDGE('',*,*,#2795,.F.);
#3943=ORIENTED_EDGE('',*,*,#2401,.F.);
#3944=ORIENTED_EDGE('',*,*,#2749,.T.);
#3945=ORIENTED_EDGE('',*,*,#2380,.F.);
#3946=ORIENTED_EDGE('',*,*,#2796,.F.);
#3947=ORIENTED_EDGE('',*,*,#2387,.F.);
#3948=ORIENTED_EDGE('',*,*,#2748,.T.);
#3949=ORIENTED_EDGE('',*,*,#2366,.F.);
#3950=ORIENTED_EDGE('',*,*,#2797,.F.);
#3951=ORIENTED_EDGE('',*,*,#2373,.F.);
#3952=ORIENTED_EDGE('',*,*,#2747,.T.);
#3953=ORIENTED_EDGE('',*,*,#2352,.F.);
#3954=ORIENTED_EDGE('',*,*,#2798,.F.);
#3955=ORIENTED_EDGE('',*,*,#2359,.F.);
#3956=ORIENTED_EDGE('',*,*,#2746,.T.);
#3957=ORIENTED_EDGE('',*,*,#2338,.F.);
#3958=ORIENTED_EDGE('',*,*,#2799,.F.);
#3959=ORIENTED_EDGE('',*,*,#2345,.F.);
#3960=ORIENTED_EDGE('',*,*,#2772,.T.);
#3961=ORIENTED_EDGE('',*,*,#2780,.T.);
#3962=ORIENTED_EDGE('',*,*,#2801,.T.);
#3963=ORIENTED_EDGE('',*,*,#2764,.T.);
#3964=ORIENTED_EDGE('',*,*,#2800,.T.);
#3965=ORIENTED_EDGE('',*,*,#2801,.F.);
#3966=ORIENTED_EDGE('',*,*,#2779,.F.);
#3967=ORIENTED_EDGE('',*,*,#2802,.F.);
#3968=ORIENTED_EDGE('',*,*,#2765,.F.);
#3969=ORIENTED_EDGE('',*,*,#2770,.T.);
#3970=ORIENTED_EDGE('',*,*,#2803,.T.);
#3971=ORIENTED_EDGE('',*,*,#2774,.T.);
#3972=ORIENTED_EDGE('',*,*,#2804,.T.);
#3973=ORIENTED_EDGE('',*,*,#2803,.F.);
#3974=ORIENTED_EDGE('',*,*,#2769,.T.);
#3975=ORIENTED_EDGE('',*,*,#2805,.T.);
#3976=ORIENTED_EDGE('',*,*,#2775,.F.);
#3977=ORIENTED_EDGE('',*,*,#2766,.F.);
#3978=ORIENTED_EDGE('',*,*,#2802,.T.);
#3979=ORIENTED_EDGE('',*,*,#2778,.F.);
#3980=ORIENTED_EDGE('',*,*,#2806,.F.);
#3981=ORIENTED_EDGE('',*,*,#2767,.T.);
#3982=ORIENTED_EDGE('',*,*,#2806,.T.);
#3983=ORIENTED_EDGE('',*,*,#2777,.F.);
#3984=ORIENTED_EDGE('',*,*,#2807,.F.);
#3985=ORIENTED_EDGE('',*,*,#2768,.T.);
#3986=ORIENTED_EDGE('',*,*,#2807,.T.);
#3987=ORIENTED_EDGE('',*,*,#2776,.F.);
#3988=ORIENTED_EDGE('',*,*,#2805,.F.);
#3989=ORIENTED_EDGE('',*,*,#2331,.F.);
#3990=ORIENTED_EDGE('',*,*,#2771,.T.);
#3991=ORIENTED_EDGE('',*,*,#2804,.F.);
#3992=ORIENTED_EDGE('',*,*,#2773,.F.);
#4431=CYLINDRICAL_SURFACE('',#4912,5.);
#4432=CYLINDRICAL_SURFACE('',#4915,1.);
#4433=CYLINDRICAL_SURFACE('',#4919,1.);
#4434=CYLINDRICAL_SURFACE('',#4923,1.);
#4435=CYLINDRICAL_SURFACE('',#4927,1.);
#4436=CYLINDRICAL_SURFACE('',#4931,1.);
#4437=CYLINDRICAL_SURFACE('',#4935,1.);
#4438=CYLINDRICAL_SURFACE('',#4939,1.);
#4439=CYLINDRICAL_SURFACE('',#4943,1.);
#4440=CYLINDRICAL_SURFACE('',#4947,1.);
#4441=CYLINDRICAL_SURFACE('',#4951,1.);
#4442=CYLINDRICAL_SURFACE('',#4955,1.);
#4443=CYLINDRICAL_SURFACE('',#4959,1.);
#4444=CYLINDRICAL_SURFACE('',#4963,1.);
#4445=CYLINDRICAL_SURFACE('',#4967,1.);
#4446=CYLINDRICAL_SURFACE('',#4971,1.);
#4447=CYLINDRICAL_SURFACE('',#4975,1.);
#4448=CYLINDRICAL_SURFACE('',#4979,1.);
#4449=CYLINDRICAL_SURFACE('',#4983,1.);
#4450=CYLINDRICAL_SURFACE('',#4987,1.);
#4451=CYLINDRICAL_SURFACE('',#4991,1.);
#4452=CYLINDRICAL_SURFACE('',#4995,1.);
#4453=CYLINDRICAL_SURFACE('',#4999,1.);
#4454=CYLINDRICAL_SURFACE('',#5003,1.);
#4455=CYLINDRICAL_SURFACE('',#5007,1.);
#4456=CYLINDRICAL_SURFACE('',#5011,1.);
#4457=CYLINDRICAL_SURFACE('',#5015,1.);
#4458=CYLINDRICAL_SURFACE('',#5019,1.);
#4459=CYLINDRICAL_SURFACE('',#5023,1.);
#4460=CYLINDRICAL_SURFACE('',#5027,1.);
#4461=CYLINDRICAL_SURFACE('',#5031,1.);
#4462=CYLINDRICAL_SURFACE('',#5035,1.);
#4463=CYLINDRICAL_SURFACE('',#5039,1.);
#4464=CYLINDRICAL_SURFACE('',#5043,1.);
#4465=CYLINDRICAL_SURFACE('',#5047,1.);
#4466=CYLINDRICAL_SURFACE('',#5051,1.);
#4467=CYLINDRICAL_SURFACE('',#5055,1.);
#4468=CYLINDRICAL_SURFACE('',#5059,1.);
#4469=CYLINDRICAL_SURFACE('',#5063,1.);
#4470=CYLINDRICAL_SURFACE('',#5067,21.9999999999943);
#4471=CYLINDRICAL_SURFACE('',#5070,21.9999999999943);
#4472=CYLINDRICAL_SURFACE('',#5073,21.9999999999943);
#4473=CYLINDRICAL_SURFACE('',#5076,21.9999999999943);
#4474=CYLINDRICAL_SURFACE('',#5079,21.9999999999943);
#4475=CYLINDRICAL_SURFACE('',#5082,21.9999999999943);
#4476=CYLINDRICAL_SURFACE('',#5085,21.9999999999943);
#4477=CYLINDRICAL_SURFACE('',#5088,21.9999999999943);
#4478=CYLINDRICAL_SURFACE('',#5091,21.9999999999943);
#4479=CYLINDRICAL_SURFACE('',#5094,21.9999999999943);
#4480=CYLINDRICAL_SURFACE('',#5097,21.9999999999943);
#4481=CYLINDRICAL_SURFACE('',#5100,21.9999999999943);
#4482=CYLINDRICAL_SURFACE('',#5103,21.9999999999943);
#4483=CYLINDRICAL_SURFACE('',#5106,21.9999999999943);
#4484=CYLINDRICAL_SURFACE('',#5109,21.9999999999943);
#4485=CYLINDRICAL_SURFACE('',#5112,21.9999999999943);
#4486=CYLINDRICAL_SURFACE('',#5115,21.9999999999943);
#4487=CYLINDRICAL_SURFACE('',#5118,21.9999999999943);
#4488=CYLINDRICAL_SURFACE('',#5121,21.9999999999943);
#4489=CYLINDRICAL_SURFACE('',#5172,17.686);
#4490=CYLINDRICAL_SURFACE('',#5173,17.686);
#4491=CYLINDRICAL_SURFACE('',#5174,17.686);
#4492=CYLINDRICAL_SURFACE('',#5175,17.686);
#4493=CYLINDRICAL_SURFACE('',#5176,17.686);
#4494=CYLINDRICAL_SURFACE('',#5177,17.686);
#4495=CYLINDRICAL_SURFACE('',#5178,17.686);
#4496=CYLINDRICAL_SURFACE('',#5179,17.686);
#4497=CYLINDRICAL_SURFACE('',#5180,17.686);
#4498=CYLINDRICAL_SURFACE('',#5181,17.686);
#4499=CYLINDRICAL_SURFACE('',#5182,17.686);
#4500=CYLINDRICAL_SURFACE('',#5183,17.686);
#4501=CYLINDRICAL_SURFACE('',#5184,17.686);
#4502=CYLINDRICAL_SURFACE('',#5185,17.686);
#4503=CYLINDRICAL_SURFACE('',#5186,17.686);
#4504=CYLINDRICAL_SURFACE('',#5187,17.686);
#4505=CYLINDRICAL_SURFACE('',#5188,17.686);
#4506=CYLINDRICAL_SURFACE('',#5189,17.686);
#4507=CYLINDRICAL_SURFACE('',#5190,17.686);
#4508=CYLINDRICAL_SURFACE('',#5191,1.);
#4509=CYLINDRICAL_SURFACE('',#5193,1.);
#4510=CYLINDRICAL_SURFACE('',#5195,21.9999999999943);
#4511=CYLINDRICAL_SURFACE('',#5196,17.686);
#4549=ADVANCED_FACE('',(#325),#4431,.F.);
#4550=ADVANCED_FACE('',(#326),#4432,.F.);
#4551=ADVANCED_FACE('',(#327),#231,.T.);
#4552=ADVANCED_FACE('',(#328),#4433,.F.);
#4553=ADVANCED_FACE('',(#329),#232,.T.);
#4554=ADVANCED_FACE('',(#330),#4434,.F.);
#4555=ADVANCED_FACE('',(#331),#233,.T.);
#4556=ADVANCED_FACE('',(#332),#4435,.F.);
#4557=ADVANCED_FACE('',(#333),#234,.T.);
#4558=ADVANCED_FACE('',(#334),#4436,.F.);
#4559=ADVANCED_FACE('',(#335),#235,.T.);
#4560=ADVANCED_FACE('',(#336),#4437,.F.);
#4561=ADVANCED_FACE('',(#337),#236,.T.);
#4562=ADVANCED_FACE('',(#338),#4438,.F.);
#4563=ADVANCED_FACE('',(#339),#237,.T.);
#4564=ADVANCED_FACE('',(#340),#4439,.F.);
#4565=ADVANCED_FACE('',(#341),#238,.T.);
#4566=ADVANCED_FACE('',(#342),#4440,.F.);
#4567=ADVANCED_FACE('',(#343),#239,.T.);
#4568=ADVANCED_FACE('',(#344),#4441,.F.);
#4569=ADVANCED_FACE('',(#345),#240,.T.);
#4570=ADVANCED_FACE('',(#346),#4442,.F.);
#4571=ADVANCED_FACE('',(#347),#241,.T.);
#4572=ADVANCED_FACE('',(#348),#4443,.F.);
#4573=ADVANCED_FACE('',(#349),#242,.T.);
#4574=ADVANCED_FACE('',(#350),#4444,.F.);
#4575=ADVANCED_FACE('',(#351),#243,.T.);
#4576=ADVANCED_FACE('',(#352),#4445,.F.);
#4577=ADVANCED_FACE('',(#353),#244,.T.);
#4578=ADVANCED_FACE('',(#354),#4446,.F.);
#4579=ADVANCED_FACE('',(#355),#245,.T.);
#4580=ADVANCED_FACE('',(#356),#4447,.F.);
#4581=ADVANCED_FACE('',(#357),#246,.T.);
#4582=ADVANCED_FACE('',(#358),#4448,.F.);
#4583=ADVANCED_FACE('',(#359),#247,.T.);
#4584=ADVANCED_FACE('',(#360),#4449,.F.);
#4585=ADVANCED_FACE('',(#361),#248,.T.);
#4586=ADVANCED_FACE('',(#362),#4450,.F.);
#4587=ADVANCED_FACE('',(#363),#249,.T.);
#4588=ADVANCED_FACE('',(#364),#4451,.F.);
#4589=ADVANCED_FACE('',(#365),#250,.T.);
#4590=ADVANCED_FACE('',(#366),#4452,.F.);
#4591=ADVANCED_FACE('',(#367),#251,.T.);
#4592=ADVANCED_FACE('',(#368),#4453,.F.);
#4593=ADVANCED_FACE('',(#369),#252,.T.);
#4594=ADVANCED_FACE('',(#370),#4454,.F.);
#4595=ADVANCED_FACE('',(#371),#253,.T.);
#4596=ADVANCED_FACE('',(#372),#4455,.F.);
#4597=ADVANCED_FACE('',(#373),#254,.T.);
#4598=ADVANCED_FACE('',(#374),#4456,.F.);
#4599=ADVANCED_FACE('',(#375),#255,.T.);
#4600=ADVANCED_FACE('',(#376),#4457,.F.);
#4601=ADVANCED_FACE('',(#377),#256,.T.);
#4602=ADVANCED_FACE('',(#378),#4458,.F.);
#4603=ADVANCED_FACE('',(#379),#257,.T.);
#4604=ADVANCED_FACE('',(#380),#4459,.F.);
#4605=ADVANCED_FACE('',(#381),#258,.T.);
#4606=ADVANCED_FACE('',(#382),#4460,.F.);
#4607=ADVANCED_FACE('',(#383),#259,.T.);
#4608=ADVANCED_FACE('',(#384),#4461,.F.);
#4609=ADVANCED_FACE('',(#385),#260,.T.);
#4610=ADVANCED_FACE('',(#386),#4462,.F.);
#4611=ADVANCED_FACE('',(#387),#261,.T.);
#4612=ADVANCED_FACE('',(#388),#4463,.F.);
#4613=ADVANCED_FACE('',(#389),#262,.T.);
#4614=ADVANCED_FACE('',(#390),#4464,.F.);
#4615=ADVANCED_FACE('',(#391),#263,.T.);
#4616=ADVANCED_FACE('',(#392),#4465,.F.);
#4617=ADVANCED_FACE('',(#393),#264,.T.);
#4618=ADVANCED_FACE('',(#394),#4466,.F.);
#4619=ADVANCED_FACE('',(#395),#265,.T.);
#4620=ADVANCED_FACE('',(#396),#4467,.F.);
#4621=ADVANCED_FACE('',(#397),#266,.T.);
#4622=ADVANCED_FACE('',(#398),#4468,.F.);
#4623=ADVANCED_FACE('',(#399),#267,.T.);
#4624=ADVANCED_FACE('',(#400),#4469,.F.);
#4625=ADVANCED_FACE('',(#401),#268,.T.);
#4626=ADVANCED_FACE('',(#402),#191,.T.);
#4627=ADVANCED_FACE('',(#403),#4470,.T.);
#4628=ADVANCED_FACE('',(#404),#192,.T.);
#4629=ADVANCED_FACE('',(#405),#193,.T.);
#4630=ADVANCED_FACE('',(#406),#4471,.T.);
#4631=ADVANCED_FACE('',(#407),#194,.T.);
#4632=ADVANCED_FACE('',(#408),#195,.T.);
#4633=ADVANCED_FACE('',(#409),#4472,.T.);
#4634=ADVANCED_FACE('',(#410),#196,.T.);
#4635=ADVANCED_FACE('',(#411),#197,.T.);
#4636=ADVANCED_FACE('',(#412),#4473,.T.);
#4637=ADVANCED_FACE('',(#413),#198,.T.);
#4638=ADVANCED_FACE('',(#414),#199,.T.);
#4639=ADVANCED_FACE('',(#415),#4474,.T.);
#4640=ADVANCED_FACE('',(#416),#200,.T.);
#4641=ADVANCED_FACE('',(#417),#201,.T.);
#4642=ADVANCED_FACE('',(#418),#4475,.T.);
#4643=ADVANCED_FACE('',(#419),#202,.T.);
#4644=ADVANCED_FACE('',(#420),#203,.T.);
#4645=ADVANCED_FACE('',(#421),#4476,.T.);
#4646=ADVANCED_FACE('',(#422),#204,.T.);
#4647=ADVANCED_FACE('',(#423),#205,.T.);
#4648=ADVANCED_FACE('',(#424),#4477,.T.);
#4649=ADVANCED_FACE('',(#425),#206,.T.);
#4650=ADVANCED_FACE('',(#426),#207,.T.);
#4651=ADVANCED_FACE('',(#427),#4478,.T.);
#4652=ADVANCED_FACE('',(#428),#208,.T.);
#4653=ADVANCED_FACE('',(#429),#209,.T.);
#4654=ADVANCED_FACE('',(#430),#4479,.T.);
#4655=ADVANCED_FACE('',(#431),#210,.T.);
#4656=ADVANCED_FACE('',(#432),#211,.T.);
#4657=ADVANCED_FACE('',(#433),#4480,.T.);
#4658=ADVANCED_FACE('',(#434),#212,.T.);
#4659=ADVANCED_FACE('',(#435),#213,.T.);
#4660=ADVANCED_FACE('',(#436),#4481,.T.);
#4661=ADVANCED_FACE('',(#437),#214,.T.);
#4662=ADVANCED_FACE('',(#438),#215,.T.);
#4663=ADVANCED_FACE('',(#439),#4482,.T.);
#4664=ADVANCED_FACE('',(#440),#216,.T.);
#4665=ADVANCED_FACE('',(#441),#217,.T.);
#4666=ADVANCED_FACE('',(#442),#4483,.T.);
#4667=ADVANCED_FACE('',(#443),#218,.T.);
#4668=ADVANCED_FACE('',(#444),#219,.T.);
#4669=ADVANCED_FACE('',(#445),#4484,.T.);
#4670=ADVANCED_FACE('',(#446),#220,.T.);
#4671=ADVANCED_FACE('',(#447),#221,.T.);
#4672=ADVANCED_FACE('',(#448),#4485,.T.);
#4673=ADVANCED_FACE('',(#449),#222,.T.);
#4674=ADVANCED_FACE('',(#450),#223,.T.);
#4675=ADVANCED_FACE('',(#451),#4486,.T.);
#4676=ADVANCED_FACE('',(#452),#224,.T.);
#4677=ADVANCED_FACE('',(#453),#225,.T.);
#4678=ADVANCED_FACE('',(#454),#4487,.T.);
#4679=ADVANCED_FACE('',(#455),#226,.T.);
#4680=ADVANCED_FACE('',(#456),#227,.T.);
#4681=ADVANCED_FACE('',(#457),#4488,.T.);
#4682=ADVANCED_FACE('',(#458),#228,.T.);
#4683=ADVANCED_FACE('',(#459,#91),#269,.F.);
#4684=ADVANCED_FACE('',(#460,#92),#270,.T.);
#4685=ADVANCED_FACE('',(#461),#4489,.T.);
#4686=ADVANCED_FACE('',(#462),#4490,.T.);
#4687=ADVANCED_FACE('',(#463),#4491,.T.);
#4688=ADVANCED_FACE('',(#464),#4492,.T.);
#4689=ADVANCED_FACE('',(#465),#4493,.T.);
#4690=ADVANCED_FACE('',(#466),#4494,.T.);
#4691=ADVANCED_FACE('',(#467),#4495,.T.);
#4692=ADVANCED_FACE('',(#468),#4496,.T.);
#4693=ADVANCED_FACE('',(#469),#4497,.T.);
#4694=ADVANCED_FACE('',(#470),#4498,.T.);
#4695=ADVANCED_FACE('',(#471),#4499,.T.);
#4696=ADVANCED_FACE('',(#472),#4500,.T.);
#4697=ADVANCED_FACE('',(#473),#4501,.T.);
#4698=ADVANCED_FACE('',(#474),#4502,.T.);
#4699=ADVANCED_FACE('',(#475),#4503,.T.);
#4700=ADVANCED_FACE('',(#476),#4504,.T.);
#4701=ADVANCED_FACE('',(#477),#4505,.T.);
#4702=ADVANCED_FACE('',(#478),#4506,.T.);
#4703=ADVANCED_FACE('',(#479),#4507,.T.);
#4704=ADVANCED_FACE('',(#480),#4508,.F.);
#4705=ADVANCED_FACE('',(#481),#271,.T.);
#4706=ADVANCED_FACE('',(#482),#4509,.F.);
#4707=ADVANCED_FACE('',(#483),#272,.T.);
#4708=ADVANCED_FACE('',(#484),#229,.T.);
#4709=ADVANCED_FACE('',(#485),#4510,.T.);
#4710=ADVANCED_FACE('',(#486),#230,.T.);
#4711=ADVANCED_FACE('',(#487),#4511,.T.);
#4825=CLOSED_SHELL('',(#4549,#4550,#4551,#4552,#4553,#4554,#4555,#4556,
#4557,#4558,#4559,#4560,#4561,#4562,#4563,#4564,#4565,#4566,#4567,#4568,
#4569,#4570,#4571,#4572,#4573,#4574,#4575,#4576,#4577,#4578,#4579,#4580,
#4581,#4582,#4583,#4584,#4585,#4586,#4587,#4588,#4589,#4590,#4591,#4592,
#4593,#4594,#4595,#4596,#4597,#4598,#4599,#4600,#4601,#4602,#4603,#4604,
#4605,#4606,#4607,#4608,#4609,#4610,#4611,#4612,#4613,#4614,#4615,#4616,
#4617,#4618,#4619,#4620,#4621,#4622,#4623,#4624,#4625,#4626,#4627,#4628,
#4629,#4630,#4631,#4632,#4633,#4634,#4635,#4636,#4637,#4638,#4639,#4640,
#4641,#4642,#4643,#4644,#4645,#4646,#4647,#4648,#4649,#4650,#4651,#4652,
#4653,#4654,#4655,#4656,#4657,#4658,#4659,#4660,#4661,#4662,#4663,#4664,
#4665,#4666,#4667,#4668,#4669,#4670,#4671,#4672,#4673,#4674,#4675,#4676,
#4677,#4678,#4679,#4680,#4681,#4682,#4683,#4684,#4685,#4686,#4687,#4688,
#4689,#4690,#4691,#4692,#4693,#4694,#4695,#4696,#4697,#4698,#4699,#4700,
#4701,#4702,#4703,#4704,#4705,#4706,#4707,#4708,#4709,#4710,#4711));
#4911=AXIS2_PLACEMENT_3D('',#6818,#5429,#5430);
#4912=AXIS2_PLACEMENT_3D('',#6819,#5431,#5432);
#4913=AXIS2_PLACEMENT_3D('',#6821,#5433,#5434);
#4914=AXIS2_PLACEMENT_3D('',#6824,#5436,#5437);
#4915=AXIS2_PLACEMENT_3D('',#6825,#5438,#5439);
#4916=AXIS2_PLACEMENT_3D('',#6828,#5440,#5441);
#4917=AXIS2_PLACEMENT_3D('',#6832,#5443,#5444);
#4918=AXIS2_PLACEMENT_3D('',#6834,#5446,#5447);
#4919=AXIS2_PLACEMENT_3D('',#6840,#5451,#5452);
#4920=AXIS2_PLACEMENT_3D('',#6843,#5453,#5454);
#4921=AXIS2_PLACEMENT_3D('',#6847,#5456,#5457);
#4922=AXIS2_PLACEMENT_3D('',#6849,#5459,#5460);
#4923=AXIS2_PLACEMENT_3D('',#6855,#5464,#5465);
#4924=AXIS2_PLACEMENT_3D('',#6858,#5466,#5467);
#4925=AXIS2_PLACEMENT_3D('',#6862,#5469,#5470);
#4926=AXIS2_PLACEMENT_3D('',#6864,#5472,#5473);
#4927=AXIS2_PLACEMENT_3D('',#6870,#5477,#5478);
#4928=AXIS2_PLACEMENT_3D('',#6873,#5479,#5480);
#4929=AXIS2_PLACEMENT_3D('',#6877,#5482,#5483);
#4930=AXIS2_PLACEMENT_3D('',#6879,#5485,#5486);
#4931=AXIS2_PLACEMENT_3D('',#6885,#5490,#5491);
#4932=AXIS2_PLACEMENT_3D('',#6888,#5492,#5493);
#4933=AXIS2_PLACEMENT_3D('',#6892,#5495,#5496);
#4934=AXIS2_PLACEMENT_3D('',#6894,#5498,#5499);
#4935=AXIS2_PLACEMENT_3D('',#6900,#5503,#5504);
#4936=AXIS2_PLACEMENT_3D('',#6903,#5505,#5506);
#4937=AXIS2_PLACEMENT_3D('',#6907,#5508,#5509);
#4938=AXIS2_PLACEMENT_3D('',#6909,#5511,#5512);
#4939=AXIS2_PLACEMENT_3D('',#6915,#5516,#5517);
#4940=AXIS2_PLACEMENT_3D('',#6918,#5518,#5519);
#4941=AXIS2_PLACEMENT_3D('',#6922,#5521,#5522);
#4942=AXIS2_PLACEMENT_3D('',#6924,#5524,#5525);
#4943=AXIS2_PLACEMENT_3D('',#6930,#5529,#5530);
#4944=AXIS2_PLACEMENT_3D('',#6933,#5531,#5532);
#4945=AXIS2_PLACEMENT_3D('',#6937,#5534,#5535);
#4946=AXIS2_PLACEMENT_3D('',#6939,#5537,#5538);
#4947=AXIS2_PLACEMENT_3D('',#6945,#5542,#5543);
#4948=AXIS2_PLACEMENT_3D('',#6948,#5544,#5545);
#4949=AXIS2_PLACEMENT_3D('',#6952,#5547,#5548);
#4950=AXIS2_PLACEMENT_3D('',#6954,#5550,#5551);
#4951=AXIS2_PLACEMENT_3D('',#6960,#5555,#5556);
#4952=AXIS2_PLACEMENT_3D('',#6963,#5557,#5558);
#4953=AXIS2_PLACEMENT_3D('',#6967,#5560,#5561);
#4954=AXIS2_PLACEMENT_3D('',#6969,#5563,#5564);
#4955=AXIS2_PLACEMENT_3D('',#6975,#5568,#5569);
#4956=AXIS2_PLACEMENT_3D('',#6978,#5570,#5571);
#4957=AXIS2_PLACEMENT_3D('',#6982,#5573,#5574);
#4958=AXIS2_PLACEMENT_3D('',#6984,#5576,#5577);
#4959=AXIS2_PLACEMENT_3D('',#6990,#5581,#5582);
#4960=AXIS2_PLACEMENT_3D('',#6993,#5583,#5584);
#4961=AXIS2_PLACEMENT_3D('',#6997,#5586,#5587);
#4962=AXIS2_PLACEMENT_3D('',#6999,#5589,#5590);
#4963=AXIS2_PLACEMENT_3D('',#7005,#5594,#5595);
#4964=AXIS2_PLACEMENT_3D('',#7008,#5596,#5597);
#4965=AXIS2_PLACEMENT_3D('',#7012,#5599,#5600);
#4966=AXIS2_PLACEMENT_3D('',#7014,#5602,#5603);
#4967=AXIS2_PLACEMENT_3D('',#7020,#5607,#5608);
#4968=AXIS2_PLACEMENT_3D('',#7023,#5609,#5610);
#4969=AXIS2_PLACEMENT_3D('',#7027,#5612,#5613);
#4970=AXIS2_PLACEMENT_3D('',#7029,#5615,#5616);
#4971=AXIS2_PLACEMENT_3D('',#7035,#5620,#5621);
#4972=AXIS2_PLACEMENT_3D('',#7038,#5622,#5623);
#4973=AXIS2_PLACEMENT_3D('',#7042,#5625,#5626);
#4974=AXIS2_PLACEMENT_3D('',#7044,#5628,#5629);
#4975=AXIS2_PLACEMENT_3D('',#7050,#5633,#5634);
#4976=AXIS2_PLACEMENT_3D('',#7053,#5635,#5636);
#4977=AXIS2_PLACEMENT_3D('',#7057,#5638,#5639);
#4978=AXIS2_PLACEMENT_3D('',#7059,#5641,#5642);
#4979=AXIS2_PLACEMENT_3D('',#7065,#5646,#5647);
#4980=AXIS2_PLACEMENT_3D('',#7068,#5648,#5649);
#4981=AXIS2_PLACEMENT_3D('',#7072,#5651,#5652);
#4982=AXIS2_PLACEMENT_3D('',#7074,#5654,#5655);
#4983=AXIS2_PLACEMENT_3D('',#7080,#5659,#5660);
#4984=AXIS2_PLACEMENT_3D('',#7083,#5661,#5662);
#4985=AXIS2_PLACEMENT_3D('',#7087,#5664,#5665);
#4986=AXIS2_PLACEMENT_3D('',#7089,#5667,#5668);
#4987=AXIS2_PLACEMENT_3D('',#7095,#5672,#5673);
#4988=AXIS2_PLACEMENT_3D('',#7098,#5674,#5675);
#4989=AXIS2_PLACEMENT_3D('',#7102,#5677,#5678);
#4990=AXIS2_PLACEMENT_3D('',#7104,#5680,#5681);
#4991=AXIS2_PLACEMENT_3D('',#7110,#5685,#5686);
#4992=AXIS2_PLACEMENT_3D('',#7113,#5687,#5688);
#4993=AXIS2_PLACEMENT_3D('',#7117,#5690,#5691);
#4994=AXIS2_PLACEMENT_3D('',#7119,#5693,#5694);
#4995=AXIS2_PLACEMENT_3D('',#7125,#5698,#5699);
#4996=AXIS2_PLACEMENT_3D('',#7128,#5700,#5701);
#4997=AXIS2_PLACEMENT_3D('',#7132,#5703,#5704);
#4998=AXIS2_PLACEMENT_3D('',#7134,#5706,#5707);
#4999=AXIS2_PLACEMENT_3D('',#7140,#5711,#5712);
#5000=AXIS2_PLACEMENT_3D('',#7143,#5713,#5714);
#5001=AXIS2_PLACEMENT_3D('',#7147,#5716,#5717);
#5002=AXIS2_PLACEMENT_3D('',#7149,#5719,#5720);
#5003=AXIS2_PLACEMENT_3D('',#7155,#5724,#5725);
#5004=AXIS2_PLACEMENT_3D('',#7158,#5726,#5727);
#5005=AXIS2_PLACEMENT_3D('',#7162,#5729,#5730);
#5006=AXIS2_PLACEMENT_3D('',#7164,#5732,#5733);
#5007=AXIS2_PLACEMENT_3D('',#7170,#5737,#5738);
#5008=AXIS2_PLACEMENT_3D('',#7173,#5739,#5740);
#5009=AXIS2_PLACEMENT_3D('',#7177,#5742,#5743);
#5010=AXIS2_PLACEMENT_3D('',#7179,#5745,#5746);
#5011=AXIS2_PLACEMENT_3D('',#7185,#5750,#5751);
#5012=AXIS2_PLACEMENT_3D('',#7188,#5752,#5753);
#5013=AXIS2_PLACEMENT_3D('',#7192,#5755,#5756);
#5014=AXIS2_PLACEMENT_3D('',#7194,#5758,#5759);
#5015=AXIS2_PLACEMENT_3D('',#7200,#5763,#5764);
#5016=AXIS2_PLACEMENT_3D('',#7203,#5765,#5766);
#5017=AXIS2_PLACEMENT_3D('',#7207,#5768,#5769);
#5018=AXIS2_PLACEMENT_3D('',#7209,#5771,#5772);
#5019=AXIS2_PLACEMENT_3D('',#7215,#5776,#5777);
#5020=AXIS2_PLACEMENT_3D('',#7218,#5778,#5779);
#5021=AXIS2_PLACEMENT_3D('',#7222,#5781,#5782);
#5022=AXIS2_PLACEMENT_3D('',#7224,#5784,#5785);
#5023=AXIS2_PLACEMENT_3D('',#7230,#5789,#5790);
#5024=AXIS2_PLACEMENT_3D('',#7233,#5791,#5792);
#5025=AXIS2_PLACEMENT_3D('',#7237,#5794,#5795);
#5026=AXIS2_PLACEMENT_3D('',#7239,#5797,#5798);
#5027=AXIS2_PLACEMENT_3D('',#7245,#5802,#5803);
#5028=AXIS2_PLACEMENT_3D('',#7248,#5804,#5805);
#5029=AXIS2_PLACEMENT_3D('',#7252,#5807,#5808);
#5030=AXIS2_PLACEMENT_3D('',#7254,#5810,#5811);
#5031=AXIS2_PLACEMENT_3D('',#7260,#5815,#5816);
#5032=AXIS2_PLACEMENT_3D('',#7263,#5817,#5818);
#5033=AXIS2_PLACEMENT_3D('',#7267,#5820,#5821);
#5034=AXIS2_PLACEMENT_3D('',#7269,#5823,#5824);
#5035=AXIS2_PLACEMENT_3D('',#7275,#5828,#5829);
#5036=AXIS2_PLACEMENT_3D('',#7278,#5830,#5831);
#5037=AXIS2_PLACEMENT_3D('',#7282,#5833,#5834);
#5038=AXIS2_PLACEMENT_3D('',#7284,#5836,#5837);
#5039=AXIS2_PLACEMENT_3D('',#7290,#5841,#5842);
#5040=AXIS2_PLACEMENT_3D('',#7293,#5843,#5844);
#5041=AXIS2_PLACEMENT_3D('',#7297,#5846,#5847);
#5042=AXIS2_PLACEMENT_3D('',#7299,#5849,#5850);
#5043=AXIS2_PLACEMENT_3D('',#7305,#5854,#5855);
#5044=AXIS2_PLACEMENT_3D('',#7308,#5856,#5857);
#5045=AXIS2_PLACEMENT_3D('',#7312,#5859,#5860);
#5046=AXIS2_PLACEMENT_3D('',#7314,#5862,#5863);
#5047=AXIS2_PLACEMENT_3D('',#7320,#5867,#5868);
#5048=AXIS2_PLACEMENT_3D('',#7323,#5869,#5870);
#5049=AXIS2_PLACEMENT_3D('',#7327,#5872,#5873);
#5050=AXIS2_PLACEMENT_3D('',#7329,#5875,#5876);
#5051=AXIS2_PLACEMENT_3D('',#7335,#5880,#5881);
#5052=AXIS2_PLACEMENT_3D('',#7338,#5882,#5883);
#5053=AXIS2_PLACEMENT_3D('',#7342,#5885,#5886);
#5054=AXIS2_PLACEMENT_3D('',#7344,#5888,#5889);
#5055=AXIS2_PLACEMENT_3D('',#7350,#5893,#5894);
#5056=AXIS2_PLACEMENT_3D('',#7353,#5895,#5896);
#5057=AXIS2_PLACEMENT_3D('',#7357,#5898,#5899);
#5058=AXIS2_PLACEMENT_3D('',#7359,#5901,#5902);
#5059=AXIS2_PLACEMENT_3D('',#7365,#5906,#5907);
#5060=AXIS2_PLACEMENT_3D('',#7368,#5908,#5909);
#5061=AXIS2_PLACEMENT_3D('',#7372,#5911,#5912);
#5062=AXIS2_PLACEMENT_3D('',#7374,#5914,#5915);
#5063=AXIS2_PLACEMENT_3D('',#7380,#5919,#5920);
#5064=AXIS2_PLACEMENT_3D('',#7383,#5921,#5922);
#5065=AXIS2_PLACEMENT_3D('',#7387,#5924,#5925);
#5066=AXIS2_PLACEMENT_3D('',#7389,#5927,#5928);
#5067=AXIS2_PLACEMENT_3D('',#7689,#5933,#5934);
#5068=AXIS2_PLACEMENT_3D('',#7691,#5935,#5936);
#5069=AXIS2_PLACEMENT_3D('',#7693,#5937,#5938);
#5070=AXIS2_PLACEMENT_3D('',#8283,#5941,#5942);
#5071=AXIS2_PLACEMENT_3D('',#8285,#5943,#5944);
#5072=AXIS2_PLACEMENT_3D('',#8287,#5945,#5946);
#5073=AXIS2_PLACEMENT_3D('',#8883,#5949,#5950);
#5074=AXIS2_PLACEMENT_3D('',#8885,#5951,#5952);
#5075=AXIS2_PLACEMENT_3D('',#8887,#5953,#5954);
#5076=AXIS2_PLACEMENT_3D('',#9477,#5957,#5958);
#5077=AXIS2_PLACEMENT_3D('',#9479,#5959,#5960);
#5078=AXIS2_PLACEMENT_3D('',#9481,#5961,#5962);
#5079=AXIS2_PLACEMENT_3D('',#10071,#5965,#5966);
#5080=AXIS2_PLACEMENT_3D('',#10073,#5967,#5968);
#5081=AXIS2_PLACEMENT_3D('',#10075,#5969,#5970);
#5082=AXIS2_PLACEMENT_3D('',#10665,#5973,#5974);
#5083=AXIS2_PLACEMENT_3D('',#10667,#5975,#5976);
#5084=AXIS2_PLACEMENT_3D('',#10669,#5977,#5978);
#5085=AXIS2_PLACEMENT_3D('',#11259,#5981,#5982);
#5086=AXIS2_PLACEMENT_3D('',#11261,#5983,#5984);
#5087=AXIS2_PLACEMENT_3D('',#11263,#5985,#5986);
#5088=AXIS2_PLACEMENT_3D('',#11853,#5989,#5990);
#5089=AXIS2_PLACEMENT_3D('',#11855,#5991,#5992);
#5090=AXIS2_PLACEMENT_3D('',#11857,#5993,#5994);
#5091=AXIS2_PLACEMENT_3D('',#12447,#5997,#5998);
#5092=AXIS2_PLACEMENT_3D('',#12449,#5999,#6000);
#5093=AXIS2_PLACEMENT_3D('',#12451,#6001,#6002);
#5094=AXIS2_PLACEMENT_3D('',#13041,#6005,#6006);
#5095=AXIS2_PLACEMENT_3D('',#13043,#6007,#6008);
#5096=AXIS2_PLACEMENT_3D('',#13045,#6009,#6010);
#5097=AXIS2_PLACEMENT_3D('',#13635,#6013,#6014);
#5098=AXIS2_PLACEMENT_3D('',#13637,#6015,#6016);
#5099=AXIS2_PLACEMENT_3D('',#13639,#6017,#6018);
#5100=AXIS2_PLACEMENT_3D('',#14229,#6021,#6022);
#5101=AXIS2_PLACEMENT_3D('',#14231,#6023,#6024);
#5102=AXIS2_PLACEMENT_3D('',#14233,#6025,#6026);
#5103=AXIS2_PLACEMENT_3D('',#14823,#6029,#6030);
#5104=AXIS2_PLACEMENT_3D('',#14825,#6031,#6032);
#5105=AXIS2_PLACEMENT_3D('',#14827,#6033,#6034);
#5106=AXIS2_PLACEMENT_3D('',#15417,#6037,#6038);
#5107=AXIS2_PLACEMENT_3D('',#15419,#6039,#6040);
#5108=AXIS2_PLACEMENT_3D('',#15421,#6041,#6042);
#5109=AXIS2_PLACEMENT_3D('',#16011,#6045,#6046);
#5110=AXIS2_PLACEMENT_3D('',#16013,#6047,#6048);
#5111=AXIS2_PLACEMENT_3D('',#16015,#6049,#6050);
#5112=AXIS2_PLACEMENT_3D('',#16605,#6053,#6054);
#5113=AXIS2_PLACEMENT_3D('',#16607,#6055,#6056);
#5114=AXIS2_PLACEMENT_3D('',#16609,#6057,#6058);
#5115=AXIS2_PLACEMENT_3D('',#17214,#6061,#6062);
#5116=AXIS2_PLACEMENT_3D('',#17216,#6063,#6064);
#5117=AXIS2_PLACEMENT_3D('',#17218,#6065,#6066);
#5118=AXIS2_PLACEMENT_3D('',#17808,#6069,#6070);
#5119=AXIS2_PLACEMENT_3D('',#17810,#6071,#6072);
#5120=AXIS2_PLACEMENT_3D('',#17812,#6073,#6074);
#5121=AXIS2_PLACEMENT_3D('',#18402,#6077,#6078);
#5122=AXIS2_PLACEMENT_3D('',#18404,#6079,#6080);
#5123=AXIS2_PLACEMENT_3D('',#18406,#6081,#6082);
#5124=AXIS2_PLACEMENT_3D('',#18702,#6084,#6085);
#5125=AXIS2_PLACEMENT_3D('',#18703,#6086,#6087);
#5126=AXIS2_PLACEMENT_3D('',#18704,#6088,#6089);
#5127=AXIS2_PLACEMENT_3D('',#18705,#6090,#6091);
#5128=AXIS2_PLACEMENT_3D('',#18706,#6092,#6093);
#5129=AXIS2_PLACEMENT_3D('',#18707,#6094,#6095);
#5130=AXIS2_PLACEMENT_3D('',#18708,#6096,#6097);
#5131=AXIS2_PLACEMENT_3D('',#18709,#6098,#6099);
#5132=AXIS2_PLACEMENT_3D('',#18710,#6100,#6101);
#5133=AXIS2_PLACEMENT_3D('',#18711,#6102,#6103);
#5134=AXIS2_PLACEMENT_3D('',#18712,#6104,#6105);
#5135=AXIS2_PLACEMENT_3D('',#18713,#6106,#6107);
#5136=AXIS2_PLACEMENT_3D('',#18714,#6108,#6109);
#5137=AXIS2_PLACEMENT_3D('',#18715,#6110,#6111);
#5138=AXIS2_PLACEMENT_3D('',#18716,#6112,#6113);
#5139=AXIS2_PLACEMENT_3D('',#18717,#6114,#6115);
#5140=AXIS2_PLACEMENT_3D('',#18718,#6116,#6117);
#5141=AXIS2_PLACEMENT_3D('',#18719,#6118,#6119);
#5142=AXIS2_PLACEMENT_3D('',#18721,#6120,#6121);
#5143=AXIS2_PLACEMENT_3D('',#18723,#6122,#6123);
#5144=AXIS2_PLACEMENT_3D('',#18802,#6125,#6126);
#5145=AXIS2_PLACEMENT_3D('',#18881,#6128,#6129);
#5146=AXIS2_PLACEMENT_3D('',#18882,#6130,#6131);
#5147=AXIS2_PLACEMENT_3D('',#18883,#6132,#6133);
#5148=AXIS2_PLACEMENT_3D('',#18884,#6134,#6135);
#5149=AXIS2_PLACEMENT_3D('',#18886,#6136,#6137);
#5150=AXIS2_PLACEMENT_3D('',#18888,#6138,#6139);
#5151=AXIS2_PLACEMENT_3D('',#18963,#6141,#6142);
#5152=AXIS2_PLACEMENT_3D('',#19035,#6144,#6145);
#5153=AXIS2_PLACEMENT_3D('',#19036,#6146,#6147);
#5154=AXIS2_PLACEMENT_3D('',#19037,#6148,#6149);
#5155=AXIS2_PLACEMENT_3D('',#19038,#6150,#6151);
#5156=AXIS2_PLACEMENT_3D('',#19039,#6152,#6153);
#5157=AXIS2_PLACEMENT_3D('',#19040,#6154,#6155);
#5158=AXIS2_PLACEMENT_3D('',#19041,#6156,#6157);
#5159=AXIS2_PLACEMENT_3D('',#19042,#6158,#6159);
#5160=AXIS2_PLACEMENT_3D('',#19043,#6160,#6161);
#5161=AXIS2_PLACEMENT_3D('',#19044,#6162,#6163);
#5162=AXIS2_PLACEMENT_3D('',#19045,#6164,#6165);
#5163=AXIS2_PLACEMENT_3D('',#19046,#6166,#6167);
#5164=AXIS2_PLACEMENT_3D('',#19047,#6168,#6169);
#5165=AXIS2_PLACEMENT_3D('',#19048,#6170,#6171);
#5166=AXIS2_PLACEMENT_3D('',#19049,#6172,#6173);
#5167=AXIS2_PLACEMENT_3D('',#19050,#6174,#6175);
#5168=AXIS2_PLACEMENT_3D('',#19051,#6176,#6177);
#5169=AXIS2_PLACEMENT_3D('',#19052,#6178,#6179);
#5170=AXIS2_PLACEMENT_3D('',#19053,#6180,#6181);
#5171=AXIS2_PLACEMENT_3D('',#19054,#6182,#6183);
#5172=AXIS2_PLACEMENT_3D('',#19055,#6184,#6185);
#5173=AXIS2_PLACEMENT_3D('',#19057,#6187,#6188);
#5174=AXIS2_PLACEMENT_3D('',#19058,#6189,#6190);
#5175=AXIS2_PLACEMENT_3D('',#19059,#6191,#6192);
#5176=AXIS2_PLACEMENT_3D('',#19060,#6193,#6194);
#5177=AXIS2_PLACEMENT_3D('',#19061,#6195,#6196);
#5178=AXIS2_PLACEMENT_3D('',#19062,#6197,#6198);
#5179=AXIS2_PLACEMENT_3D('',#19063,#6199,#6200);
#5180=AXIS2_PLACEMENT_3D('',#19064,#6201,#6202);
#5181=AXIS2_PLACEMENT_3D('',#19065,#6203,#6204);
#5182=AXIS2_PLACEMENT_3D('',#19066,#6205,#6206);
#5183=AXIS2_PLACEMENT_3D('',#19067,#6207,#6208);
#5184=AXIS2_PLACEMENT_3D('',#19068,#6209,#6210);
#5185=AXIS2_PLACEMENT_3D('',#19069,#6211,#6212);
#5186=AXIS2_PLACEMENT_3D('',#19070,#6213,#6214);
#5187=AXIS2_PLACEMENT_3D('',#19071,#6215,#6216);
#5188=AXIS2_PLACEMENT_3D('',#19072,#6217,#6218);
#5189=AXIS2_PLACEMENT_3D('',#19073,#6219,#6220);
#5190=AXIS2_PLACEMENT_3D('',#19074,#6221,#6222);
#5191=AXIS2_PLACEMENT_3D('',#19075,#6223,#6224);
#5192=AXIS2_PLACEMENT_3D('',#19077,#6226,#6227);
#5193=AXIS2_PLACEMENT_3D('',#19079,#6229,#6230);
#5194=AXIS2_PLACEMENT_3D('',#19082,#6233,#6234);
#5195=AXIS2_PLACEMENT_3D('',#19235,#6237,#6238);
#5196=AXIS2_PLACEMENT_3D('',#19387,#6240,#6241);
#5429=DIRECTION('axis',(0.,0.,1.));
#5430=DIRECTION('refdir',(1.,0.,0.));
#5431=DIRECTION('center_axis',(0.,0.,-1.));
#5432=DIRECTION('ref_axis',(-1.,0.,0.));
#5433=DIRECTION('center_axis',(0.,0.,-1.));
#5434=DIRECTION('ref_axis',(-1.,0.,0.));
#5435=DIRECTION('',(0.,0.,-1.));
#5436=DIRECTION('center_axis',(0.,0.,1.));
#5437=DIRECTION('ref_axis',(-1.,0.,0.));
#5438=DIRECTION('center_axis',(0.,0.,-1.));
#5439=DIRECTION('ref_axis',(-0.830130914723544,-0.557568528900486,0.));
#5440=DIRECTION('center_axis',(0.,0.,-1.));
#5441=DIRECTION('ref_axis',(-0.830130914723544,-0.557568528900486,0.));
#5442=DIRECTION('',(0.,0.,-1.));
#5443=DIRECTION('center_axis',(0.,0.,-1.));
#5444=DIRECTION('ref_axis',(-0.830130914723544,-0.557568528900486,0.));
#5445=DIRECTION('',(0.,0.,1.));
#5446=DIRECTION('center_axis',(0.21892739748686,0.975741151448288,0.));
#5447=DIRECTION('ref_axis',(-0.975741151448288,0.21892739748686,0.));
#5448=DIRECTION('',(-0.975741151448288,0.21892739748686,0.));
#5449=DIRECTION('',(0.,0.,1.));
#5450=DIRECTION('',(0.975741151448288,-0.21892739748686,0.));
#5451=DIRECTION('center_axis',(0.,0.,1.));
#5452=DIRECTION('ref_axis',(-0.343859459137252,0.939021124555692,0.));
#5453=DIRECTION('center_axis',(0.,0.,-1.));
#5454=DIRECTION('ref_axis',(-0.343859459137252,0.939021124555692,0.));
#5455=DIRECTION('',(0.,0.,1.));
#5456=DIRECTION('center_axis',(0.,0.,-1.));
#5457=DIRECTION('ref_axis',(-0.343859459137252,0.939021124555692,0.));
#5458=DIRECTION('',(0.,0.,-1.));
#5459=DIRECTION('center_axis',(-0.396410273775032,-0.918073469198192,0.));
#5460=DIRECTION('ref_axis',(0.918073469198192,-0.396410273775032,0.));
#5461=DIRECTION('',(0.918073469198192,-0.396410273775032,0.));
#5462=DIRECTION('',(0.,0.,1.));
#5463=DIRECTION('',(0.918073469198192,-0.396410273775032,0.));
#5464=DIRECTION('center_axis',(0.,0.,-1.));
#5465=DIRECTION('ref_axis',(-0.961799566784773,-0.273754622486313,0.));
#5466=DIRECTION('center_axis',(0.,0.,-1.));
#5467=DIRECTION('ref_axis',(-0.961799566784773,-0.273754622486313,0.));
#5468=DIRECTION('',(0.,0.,-1.));
#5469=DIRECTION('center_axis',(0.,0.,-1.));
#5470=DIRECTION('ref_axis',(-0.961799566784773,-0.273754622486313,0.));
#5471=DIRECTION('',(0.,0.,1.));
#5472=DIRECTION('center_axis',(0.509732925883917,0.860332693944512,0.));
#5473=DIRECTION('ref_axis',(-0.860332693944512,0.509732925883917,0.));
#5474=DIRECTION('',(-0.860332693944512,0.509732925883917,0.));
#5475=DIRECTION('',(0.,0.,1.));
#5476=DIRECTION('',(0.860332693944512,-0.509732925883917,0.));
#5477=DIRECTION('center_axis',(0.,0.,1.));
#5478=DIRECTION('ref_axis',(-0.0368562937374252,0.999320575997483,0.));
#5479=DIRECTION('center_axis',(0.,0.,-1.));
#5480=DIRECTION('ref_axis',(-0.0368562937374252,0.999320575997483,0.));
#5481=DIRECTION('',(0.,0.,1.));
#5482=DIRECTION('center_axis',(0.,0.,-1.));
#5483=DIRECTION('ref_axis',(-0.0368562937374252,0.999320575997483,0.));
#5484=DIRECTION('',(0.,0.,-1.));
#5485=DIRECTION('center_axis',(-0.660708878067096,-0.750642243977328,0.));
#5486=DIRECTION('ref_axis',(0.750642243977328,-0.660708878067096,0.));
#5487=DIRECTION('',(0.750642243977328,-0.660708878067096,0.));
#5488=DIRECTION('',(0.,0.,1.));
#5489=DIRECTION('',(0.750642243977328,-0.660708878067096,0.));
#5490=DIRECTION('center_axis',(0.,0.,-1.));
#5491=DIRECTION('ref_axis',(-0.999320575997483,0.0368562937374283,0.));
#5492=DIRECTION('center_axis',(0.,0.,-1.));
#5493=DIRECTION('ref_axis',(-0.999320575997483,0.0368562937374283,0.));
#5494=DIRECTION('',(0.,0.,-1.));
#5495=DIRECTION('center_axis',(0.,0.,-1.));
#5496=DIRECTION('ref_axis',(-0.999320575997483,0.0368562937374283,0.));
#5497=DIRECTION('',(0.,0.,1.));
#5498=DIRECTION('center_axis',(0.750642243977329,0.660708878067096,0.));
#5499=DIRECTION('ref_axis',(-0.660708878067096,0.750642243977329,0.));
#5500=DIRECTION('',(-0.660708878067096,0.750642243977329,0.));
#5501=DIRECTION('',(0.,0.,1.));
#5502=DIRECTION('',(0.660708878067096,-0.750642243977329,0.));
#5503=DIRECTION('center_axis',(0.,0.,1.));
#5504=DIRECTION('ref_axis',(0.273754622486313,0.961799566784773,0.));
#5505=DIRECTION('center_axis',(0.,0.,-1.));
#5506=DIRECTION('ref_axis',(0.273754622486313,0.961799566784773,0.));
#5507=DIRECTION('',(0.,0.,1.));
#5508=DIRECTION('center_axis',(0.,0.,-1.));
#5509=DIRECTION('ref_axis',(0.273754622486313,0.961799566784773,0.));
#5510=DIRECTION('',(0.,0.,-1.));
#5511=DIRECTION('center_axis',(-0.860332693944512,-0.509732925883917,0.));
#5512=DIRECTION('ref_axis',(0.509732925883917,-0.860332693944512,0.));
#5513=DIRECTION('',(0.509732925883917,-0.860332693944512,0.));
#5514=DIRECTION('',(0.,0.,1.));
#5515=DIRECTION('',(0.509732925883917,-0.860332693944512,0.));
#5516=DIRECTION('center_axis',(0.,0.,-1.));
#5517=DIRECTION('ref_axis',(-0.939021124555692,0.343859459137252,0.));
#5518=DIRECTION('center_axis',(0.,0.,-1.));
#5519=DIRECTION('ref_axis',(-0.939021124555692,0.343859459137252,0.));
#5520=DIRECTION('',(0.,0.,-1.));
#5521=DIRECTION('center_axis',(0.,0.,-1.));
#5522=DIRECTION('ref_axis',(-0.939021124555692,0.343859459137252,0.));
#5523=DIRECTION('',(0.,0.,1.));
#5524=DIRECTION('center_axis',(0.918073469198192,0.396410273775032,0.));
#5525=DIRECTION('ref_axis',(-0.396410273775032,0.918073469198192,0.));
#5526=DIRECTION('',(-0.396410273775032,0.918073469198192,0.));
#5527=DIRECTION('',(0.,0.,1.));
#5528=DIRECTION('',(0.396410273775032,-0.918073469198192,0.));
#5529=DIRECTION('center_axis',(0.,0.,1.));
#5530=DIRECTION('ref_axis',(0.557568528900487,0.830130914723543,0.));
#5531=DIRECTION('center_axis',(0.,0.,-1.));
#5532=DIRECTION('ref_axis',(0.557568528900487,0.830130914723543,0.));
#5533=DIRECTION('',(0.,0.,1.));
#5534=DIRECTION('center_axis',(0.,0.,-1.));
#5535=DIRECTION('ref_axis',(0.557568528900487,0.830130914723543,0.));
#5536=DIRECTION('',(0.,0.,-1.));
#5537=DIRECTION('center_axis',(-0.975741151448288,-0.218927397486859,0.));
#5538=DIRECTION('ref_axis',(0.218927397486859,-0.975741151448288,0.));
#5539=DIRECTION('',(0.218927397486859,-0.975741151448288,0.));
#5540=DIRECTION('',(0.,0.,1.));
#5541=DIRECTION('',(0.218927397486859,-0.975741151448288,0.));
#5542=DIRECTION('center_axis',(0.,0.,-1.));
#5543=DIRECTION('ref_axis',(-0.786803742897506,0.617203264866993,0.));
#5544=DIRECTION('center_axis',(0.,0.,-1.));
#5545=DIRECTION('ref_axis',(-0.786803742897506,0.617203264866993,0.));
#5546=DIRECTION('',(0.,0.,-1.));
#5547=DIRECTION('center_axis',(0.,0.,-1.));
#5548=DIRECTION('ref_axis',(-0.786803742897506,0.617203264866993,0.));
#5549=DIRECTION('',(0.,0.,1.));
#5550=DIRECTION('center_axis',(0.995637266659949,0.0933082699330834,0.));
#5551=DIRECTION('ref_axis',(-0.0933082699330834,0.995637266659949,0.));
#5552=DIRECTION('',(-0.0933082699330834,0.995637266659949,0.));
#5553=DIRECTION('',(0.,0.,1.));
#5554=DIRECTION('',(0.0933082699330834,-0.995637266659949,0.));
#5555=DIRECTION('center_axis',(0.,0.,1.));
#5556=DIRECTION('ref_axis',(0.786803742897505,0.617203264866994,0.));
#5557=DIRECTION('center_axis',(0.,0.,-1.));
#5558=DIRECTION('ref_axis',(0.786803742897505,0.617203264866994,0.));
#5559=DIRECTION('',(0.,0.,1.));
#5560=DIRECTION('center_axis',(0.,0.,-1.));
#5561=DIRECTION('ref_axis',(0.786803742897505,0.617203264866994,0.));
#5562=DIRECTION('',(0.,0.,-1.));
#5563=DIRECTION('center_axis',(-0.995637266659949,0.0933082699330838,0.));
#5564=DIRECTION('ref_axis',(-0.0933082699330838,-0.995637266659949,0.));
#5565=DIRECTION('',(-0.0933082699330838,-0.995637266659949,0.));
#5566=DIRECTION('',(0.,0.,1.));
#5567=DIRECTION('',(-0.0933082699330838,-0.995637266659949,0.));
#5568=DIRECTION('center_axis',(0.,0.,-1.));
#5569=DIRECTION('ref_axis',(-0.557568528900486,0.830130914723544,0.));
#5570=DIRECTION('center_axis',(0.,0.,-1.));
#5571=DIRECTION('ref_axis',(-0.557568528900486,0.830130914723544,0.));
#5572=DIRECTION('',(0.,0.,-1.));
#5573=DIRECTION('center_axis',(0.,0.,-1.));
#5574=DIRECTION('ref_axis',(-0.557568528900486,0.830130914723544,0.));
#5575=DIRECTION('',(0.,0.,1.));
#5576=DIRECTION('center_axis',(0.975741151448288,-0.21892739748686,0.));
#5577=DIRECTION('ref_axis',(0.21892739748686,0.975741151448288,0.));
#5578=DIRECTION('',(0.21892739748686,0.975741151448288,0.));
#5579=DIRECTION('',(0.,0.,1.));
#5580=DIRECTION('',(-0.21892739748686,-0.975741151448288,0.));
#5581=DIRECTION('center_axis',(0.,0.,1.));
#5582=DIRECTION('ref_axis',(0.939021124555691,0.343859459137256,0.));
#5583=DIRECTION('center_axis',(0.,0.,-1.));
#5584=DIRECTION('ref_axis',(0.939021124555691,0.343859459137256,0.));
#5585=DIRECTION('',(0.,0.,1.));
#5586=DIRECTION('center_axis',(0.,0.,-1.));
#5587=DIRECTION('ref_axis',(0.939021124555691,0.343859459137256,0.));
#5588=DIRECTION('',(0.,0.,-1.));
#5589=DIRECTION('center_axis',(-0.918073469198192,0.396410273775032,0.));
#5590=DIRECTION('ref_axis',(-0.396410273775032,-0.918073469198192,0.));
#5591=DIRECTION('',(-0.396410273775032,-0.918073469198192,0.));
#5592=DIRECTION('',(0.,0.,1.));
#5593=DIRECTION('',(-0.396410273775032,-0.918073469198192,0.));
#5594=DIRECTION('center_axis',(0.,0.,-1.));
#5595=DIRECTION('ref_axis',(-0.273754622486312,0.961799566784773,0.));
#5596=DIRECTION('center_axis',(0.,0.,-1.));
#5597=DIRECTION('ref_axis',(-0.273754622486312,0.961799566784773,0.));
#5598=DIRECTION('',(0.,0.,-1.));
#5599=DIRECTION('center_axis',(0.,0.,-1.));
#5600=DIRECTION('ref_axis',(-0.273754622486312,0.961799566784773,0.));
#5601=DIRECTION('',(0.,0.,1.));
#5602=DIRECTION('center_axis',(0.860332693944512,-0.509732925883917,0.));
#5603=DIRECTION('ref_axis',(0.509732925883917,0.860332693944512,0.));
#5604=DIRECTION('',(0.509732925883917,0.860332693944512,0.));
#5605=DIRECTION('',(0.,0.,1.));
#5606=DIRECTION('',(-0.509732925883917,-0.860332693944512,0.));
#5607=DIRECTION('center_axis',(0.,0.,1.));
#5608=DIRECTION('ref_axis',(0.999320575997482,0.0368562937374314,0.));
#5609=DIRECTION('center_axis',(0.,0.,-1.));
#5610=DIRECTION('ref_axis',(0.999320575997482,0.0368562937374314,0.));
#5611=DIRECTION('',(0.,0.,1.));
#5612=DIRECTION('center_axis',(0.,0.,-1.));
#5613=DIRECTION('ref_axis',(0.999320575997482,0.0368562937374314,0.));
#5614=DIRECTION('',(0.,0.,-1.));
#5615=DIRECTION('center_axis',(-0.750642243977328,0.660708878067096,0.));
#5616=DIRECTION('ref_axis',(-0.660708878067096,-0.750642243977328,0.));
#5617=DIRECTION('',(-0.660708878067096,-0.750642243977328,0.));
#5618=DIRECTION('',(0.,0.,1.));
#5619=DIRECTION('',(-0.660708878067096,-0.750642243977328,0.));
#5620=DIRECTION('center_axis',(0.,0.,-1.));
#5621=DIRECTION('ref_axis',(0.0368562937374315,0.999320575997482,0.));
#5622=DIRECTION('center_axis',(0.,0.,-1.));
#5623=DIRECTION('ref_axis',(0.0368562937374315,0.999320575997482,0.));
#5624=DIRECTION('',(0.,0.,-1.));
#5625=DIRECTION('center_axis',(0.,0.,-1.));
#5626=DIRECTION('ref_axis',(0.0368562937374315,0.999320575997482,0.));
#5627=DIRECTION('',(0.,0.,1.));
#5628=DIRECTION('center_axis',(0.660708878067096,-0.750642243977329,0.));
#5629=DIRECTION('ref_axis',(0.750642243977329,0.660708878067096,0.));
#5630=DIRECTION('',(0.750642243977329,0.660708878067096,0.));
#5631=DIRECTION('',(0.,0.,1.));
#5632=DIRECTION('',(-0.750642243977328,-0.660708878067096,0.));
#5633=DIRECTION('center_axis',(0.,0.,1.));
#5634=DIRECTION('ref_axis',(0.961799566784773,-0.273754622486311,0.));
#5635=DIRECTION('center_axis',(0.,0.,-1.));
#5636=DIRECTION('ref_axis',(0.961799566784773,-0.273754622486311,0.));
#5637=DIRECTION('',(0.,0.,1.));
#5638=DIRECTION('center_axis',(0.,0.,-1.));
#5639=DIRECTION('ref_axis',(0.961799566784773,-0.273754622486311,0.));
#5640=DIRECTION('',(0.,0.,-1.));
#5641=DIRECTION('center_axis',(-0.509732925883917,0.860332693944512,0.));
#5642=DIRECTION('ref_axis',(-0.860332693944512,-0.509732925883917,0.));
#5643=DIRECTION('',(-0.860332693944512,-0.509732925883917,0.));
#5644=DIRECTION('',(0.,0.,1.));
#5645=DIRECTION('',(-0.860332693944512,-0.509732925883917,0.));
#5646=DIRECTION('center_axis',(0.,0.,-1.));
#5647=DIRECTION('ref_axis',(0.343859459137253,0.939021124555692,0.));
#5648=DIRECTION('center_axis',(0.,0.,-1.));
#5649=DIRECTION('ref_axis',(0.343859459137253,0.939021124555692,0.));
#5650=DIRECTION('',(0.,0.,-1.));
#5651=DIRECTION('center_axis',(0.,0.,-1.));
#5652=DIRECTION('ref_axis',(0.343859459137253,0.939021124555692,0.));
#5653=DIRECTION('',(0.,0.,1.));
#5654=DIRECTION('center_axis',(0.396410273775032,-0.918073469198192,0.));
#5655=DIRECTION('ref_axis',(0.918073469198192,0.396410273775032,0.));
#5656=DIRECTION('',(0.918073469198192,0.396410273775032,0.));
#5657=DIRECTION('',(0.,0.,1.));
#5658=DIRECTION('',(-0.918073469198192,-0.396410273775032,0.));
#5659=DIRECTION('center_axis',(0.,0.,1.));
#5660=DIRECTION('ref_axis',(0.830130914723543,-0.557568528900488,0.));
#5661=DIRECTION('center_axis',(0.,0.,-1.));
#5662=DIRECTION('ref_axis',(0.830130914723543,-0.557568528900488,0.));
#5663=DIRECTION('',(0.,0.,1.));
#5664=DIRECTION('center_axis',(0.,0.,-1.));
#5665=DIRECTION('ref_axis',(0.830130914723543,-0.557568528900488,0.));
#5666=DIRECTION('',(0.,0.,-1.));
#5667=DIRECTION('center_axis',(-0.218927397486859,0.975741151448288,0.));
#5668=DIRECTION('ref_axis',(-0.975741151448288,-0.218927397486859,0.));
#5669=DIRECTION('',(-0.975741151448288,-0.218927397486859,0.));
#5670=DIRECTION('',(0.,0.,1.));
#5671=DIRECTION('',(-0.975741151448288,-0.218927397486859,0.));
#5672=DIRECTION('center_axis',(0.,0.,-1.));
#5673=DIRECTION('ref_axis',(0.617203264866995,0.786803742897504,0.));
#5674=DIRECTION('center_axis',(0.,0.,-1.));
#5675=DIRECTION('ref_axis',(0.617203264866995,0.786803742897504,0.));
#5676=DIRECTION('',(0.,0.,-1.));
#5677=DIRECTION('center_axis',(0.,0.,-1.));
#5678=DIRECTION('ref_axis',(0.617203264866995,0.786803742897504,0.));
#5679=DIRECTION('',(0.,0.,1.));
#5680=DIRECTION('center_axis',(0.0933082699330836,-0.995637266659949,0.));
#5681=DIRECTION('ref_axis',(0.995637266659949,0.0933082699330836,0.));
#5682=DIRECTION('',(0.995637266659949,0.0933082699330836,0.));
#5683=DIRECTION('',(0.,0.,1.));
#5684=DIRECTION('',(-0.995637266659949,-0.0933082699330836,0.));
#5685=DIRECTION('center_axis',(0.,0.,1.));
#5686=DIRECTION('ref_axis',(0.617203264866993,-0.786803742897506,0.));
#5687=DIRECTION('center_axis',(0.,0.,-1.));
#5688=DIRECTION('ref_axis',(0.617203264866993,-0.786803742897506,0.));
#5689=DIRECTION('',(0.,0.,1.));
#5690=DIRECTION('center_axis',(0.,0.,-1.));
#5691=DIRECTION('ref_axis',(0.617203264866993,-0.786803742897506,0.));
#5692=DIRECTION('',(0.,0.,-1.));
#5693=DIRECTION('center_axis',(0.0933082699330837,0.995637266659949,0.));
#5694=DIRECTION('ref_axis',(-0.995637266659949,0.0933082699330837,0.));
#5695=DIRECTION('',(-0.995637266659949,0.0933082699330837,0.));
#5696=DIRECTION('',(0.,0.,1.));
#5697=DIRECTION('',(-0.995637266659949,0.0933082699330837,0.));
#5698=DIRECTION('center_axis',(0.,0.,-1.));
#5699=DIRECTION('ref_axis',(0.830130914723545,0.557568528900485,0.));
#5700=DIRECTION('center_axis',(0.,0.,-1.));
#5701=DIRECTION('ref_axis',(0.830130914723545,0.557568528900485,0.));
#5702=DIRECTION('',(0.,0.,-1.));
#5703=DIRECTION('center_axis',(0.,0.,-1.));
#5704=DIRECTION('ref_axis',(0.830130914723545,0.557568528900485,0.));
#5705=DIRECTION('',(0.,0.,1.));
#5706=DIRECTION('center_axis',(-0.218927397486859,-0.975741151448288,0.));
#5707=DIRECTION('ref_axis',(0.975741151448288,-0.218927397486859,0.));
#5708=DIRECTION('',(0.975741151448288,-0.218927397486859,0.));
#5709=DIRECTION('',(0.,0.,1.));
#5710=DIRECTION('',(-0.975741151448288,0.218927397486859,0.));
#5711=DIRECTION('center_axis',(0.,0.,1.));
#5712=DIRECTION('ref_axis',(0.343859459137252,-0.939021124555692,0.));
#5713=DIRECTION('center_axis',(0.,0.,-1.));
#5714=DIRECTION('ref_axis',(0.343859459137252,-0.939021124555692,0.));
#5715=DIRECTION('',(0.,0.,1.));
#5716=DIRECTION('center_axis',(0.,0.,-1.));
#5717=DIRECTION('ref_axis',(0.343859459137252,-0.939021124555692,0.));
#5718=DIRECTION('',(0.,0.,-1.));
#5719=DIRECTION('center_axis',(0.396410273775032,0.918073469198192,0.));
#5720=DIRECTION('ref_axis',(-0.918073469198192,0.396410273775032,0.));
#5721=DIRECTION('',(-0.918073469198192,0.396410273775032,0.));
#5722=DIRECTION('',(0.,0.,1.));
#5723=DIRECTION('',(-0.918073469198192,0.396410273775032,0.));
#5724=DIRECTION('center_axis',(0.,0.,-1.));
#5725=DIRECTION('ref_axis',(0.961799566784772,0.273754622486314,0.));
#5726=DIRECTION('center_axis',(0.,0.,-1.));
#5727=DIRECTION('ref_axis',(0.961799566784772,0.273754622486314,0.));
#5728=DIRECTION('',(0.,0.,-1.));
#5729=DIRECTION('center_axis',(0.,0.,-1.));
#5730=DIRECTION('ref_axis',(0.961799566784772,0.273754622486314,0.));
#5731=DIRECTION('',(0.,0.,1.));
#5732=DIRECTION('center_axis',(-0.509732925883917,-0.860332693944512,0.));
#5733=DIRECTION('ref_axis',(0.860332693944512,-0.509732925883917,0.));
#5734=DIRECTION('',(0.860332693944512,-0.509732925883917,0.));
#5735=DIRECTION('',(0.,0.,1.));
#5736=DIRECTION('',(-0.860332693944512,0.509732925883917,0.));
#5737=DIRECTION('center_axis',(0.,0.,1.));
#5738=DIRECTION('ref_axis',(0.0368562937374283,-0.999320575997483,0.));
#5739=DIRECTION('center_axis',(0.,0.,-1.));
#5740=DIRECTION('ref_axis',(0.0368562937374283,-0.999320575997483,0.));
#5741=DIRECTION('',(0.,0.,1.));
#5742=DIRECTION('center_axis',(0.,0.,-1.));
#5743=DIRECTION('ref_axis',(0.0368562937374283,-0.999320575997483,0.));
#5744=DIRECTION('',(0.,0.,-1.));
#5745=DIRECTION('center_axis',(0.660708878067096,0.750642243977328,0.));
#5746=DIRECTION('ref_axis',(-0.750642243977328,0.660708878067096,0.));
#5747=DIRECTION('',(-0.750642243977328,0.660708878067096,0.));
#5748=DIRECTION('',(0.,0.,1.));
#5749=DIRECTION('',(-0.750642243977328,0.660708878067096,0.));
#5750=DIRECTION('center_axis',(0.,0.,-1.));
#5751=DIRECTION('ref_axis',(0.999320575997483,-0.0368562937374252,0.));
#5752=DIRECTION('center_axis',(0.,0.,-1.));
#5753=DIRECTION('ref_axis',(0.999320575997483,-0.0368562937374252,0.));
#5754=DIRECTION('',(0.,0.,-1.));
#5755=DIRECTION('center_axis',(0.,0.,-1.));
#5756=DIRECTION('ref_axis',(0.999320575997483,-0.0368562937374252,0.));
#5757=DIRECTION('',(0.,0.,1.));
#5758=DIRECTION('center_axis',(-0.750642243977329,-0.660708878067096,0.));
#5759=DIRECTION('ref_axis',(0.660708878067096,-0.750642243977329,0.));
#5760=DIRECTION('',(0.660708878067096,-0.750642243977329,0.));
#5761=DIRECTION('',(0.,0.,1.));
#5762=DIRECTION('',(-0.660708878067096,0.750642243977328,0.));
#5763=DIRECTION('center_axis',(0.,0.,1.));
#5764=DIRECTION('ref_axis',(-0.273754622486316,-0.961799566784772,0.));
#5765=DIRECTION('center_axis',(0.,0.,-1.));
#5766=DIRECTION('ref_axis',(-0.273754622486316,-0.961799566784772,0.));
#5767=DIRECTION('',(0.,0.,1.));
#5768=DIRECTION('center_axis',(0.,0.,-1.));
#5769=DIRECTION('ref_axis',(-0.273754622486316,-0.961799566784772,0.));
#5770=DIRECTION('',(0.,0.,-1.));
#5771=DIRECTION('center_axis',(0.860332693944512,0.509732925883917,0.));
#5772=DIRECTION('ref_axis',(-0.509732925883917,0.860332693944512,0.));
#5773=DIRECTION('',(-0.509732925883917,0.860332693944512,0.));
#5774=DIRECTION('',(0.,0.,1.));
#5775=DIRECTION('',(-0.509732925883917,0.860332693944512,0.));
#5776=DIRECTION('center_axis',(0.,0.,-1.));
#5777=DIRECTION('ref_axis',(0.939021124555692,-0.343859459137252,0.));
#5778=DIRECTION('center_axis',(0.,0.,-1.));
#5779=DIRECTION('ref_axis',(0.939021124555692,-0.343859459137252,0.));
#5780=DIRECTION('',(0.,0.,-1.));
#5781=DIRECTION('center_axis',(0.,0.,-1.));
#5782=DIRECTION('ref_axis',(0.939021124555692,-0.343859459137252,0.));
#5783=DIRECTION('',(0.,0.,1.));
#5784=DIRECTION('center_axis',(-0.918073469198192,-0.396410273775032,0.));
#5785=DIRECTION('ref_axis',(0.396410273775032,-0.918073469198192,0.));
#5786=DIRECTION('',(0.396410273775032,-0.918073469198192,0.));
#5787=DIRECTION('',(0.,0.,1.));
#5788=DIRECTION('',(-0.396410273775032,0.918073469198192,0.));
#5789=DIRECTION('center_axis',(0.,0.,1.));
#5790=DIRECTION('ref_axis',(-0.557568528900488,-0.830130914723543,0.));
#5791=DIRECTION('center_axis',(0.,0.,-1.));
#5792=DIRECTION('ref_axis',(-0.557568528900488,-0.830130914723543,0.));
#5793=DIRECTION('',(0.,0.,1.));
#5794=DIRECTION('center_axis',(0.,0.,-1.));
#5795=DIRECTION('ref_axis',(-0.557568528900488,-0.830130914723543,0.));
#5796=DIRECTION('',(0.,0.,-1.));
#5797=DIRECTION('center_axis',(0.975741151448288,0.218927397486859,0.));
#5798=DIRECTION('ref_axis',(-0.218927397486859,0.975741151448288,0.));
#5799=DIRECTION('',(-0.218927397486859,0.975741151448288,0.));
#5800=DIRECTION('',(0.,0.,1.));
#5801=DIRECTION('',(-0.218927397486859,0.975741151448288,0.));
#5802=DIRECTION('center_axis',(0.,0.,-1.));
#5803=DIRECTION('ref_axis',(0.786803742897506,-0.617203264866993,0.));
#5804=DIRECTION('center_axis',(0.,0.,-1.));
#5805=DIRECTION('ref_axis',(0.786803742897506,-0.617203264866993,0.));
#5806=DIRECTION('',(0.,0.,-1.));
#5807=DIRECTION('center_axis',(0.,0.,-1.));
#5808=DIRECTION('ref_axis',(0.786803742897506,-0.617203264866993,0.));
#5809=DIRECTION('',(0.,0.,1.));
#5810=DIRECTION('center_axis',(-0.995637266659949,-0.0933082699330836,0.));
#5811=DIRECTION('ref_axis',(0.0933082699330836,-0.995637266659949,0.));
#5812=DIRECTION('',(0.0933082699330836,-0.995637266659949,0.));
#5813=DIRECTION('',(0.,0.,1.));
#5814=DIRECTION('',(-0.0933082699330836,0.995637266659949,0.));
#5815=DIRECTION('center_axis',(0.,0.,1.));
#5816=DIRECTION('ref_axis',(-0.786803742897506,-0.617203264866993,0.));
#5817=DIRECTION('center_axis',(0.,0.,-1.));
#5818=DIRECTION('ref_axis',(-0.786803742897506,-0.617203264866993,0.));
#5819=DIRECTION('',(0.,0.,1.));
#5820=DIRECTION('center_axis',(0.,0.,-1.));
#5821=DIRECTION('ref_axis',(-0.786803742897506,-0.617203264866993,0.));
#5822=DIRECTION('',(0.,0.,-1.));
#5823=DIRECTION('center_axis',(0.995637266659949,-0.0933082699330837,0.));
#5824=DIRECTION('ref_axis',(0.0933082699330837,0.995637266659949,0.));
#5825=DIRECTION('',(0.0933082699330837,0.995637266659949,0.));
#5826=DIRECTION('',(0.,0.,1.));
#5827=DIRECTION('',(0.0933082699330837,0.995637266659949,0.));
#5828=DIRECTION('center_axis',(0.,0.,-1.));
#5829=DIRECTION('ref_axis',(0.557568528900485,-0.830130914723545,0.));
#5830=DIRECTION('center_axis',(0.,0.,-1.));
#5831=DIRECTION('ref_axis',(0.557568528900485,-0.830130914723545,0.));
#5832=DIRECTION('',(0.,0.,-1.));
#5833=DIRECTION('center_axis',(0.,0.,-1.));
#5834=DIRECTION('ref_axis',(0.557568528900485,-0.830130914723545,0.));
#5835=DIRECTION('',(0.,0.,1.));
#5836=DIRECTION('center_axis',(-0.975741151448288,0.218927397486859,0.));
#5837=DIRECTION('ref_axis',(-0.218927397486859,-0.975741151448288,0.));
#5838=DIRECTION('',(-0.218927397486859,-0.975741151448288,0.));
#5839=DIRECTION('',(0.,0.,1.));
#5840=DIRECTION('',(0.218927397486859,0.975741151448288,0.));
#5841=DIRECTION('center_axis',(0.,0.,1.));
#5842=DIRECTION('ref_axis',(-0.939021124555691,-0.343859459137255,0.));
#5843=DIRECTION('center_axis',(0.,0.,-1.));
#5844=DIRECTION('ref_axis',(-0.939021124555691,-0.343859459137255,0.));
#5845=DIRECTION('',(0.,0.,1.));
#5846=DIRECTION('center_axis',(0.,0.,-1.));
#5847=DIRECTION('ref_axis',(-0.939021124555691,-0.343859459137255,0.));
#5848=DIRECTION('',(0.,0.,-1.));
#5849=DIRECTION('center_axis',(0.918073469198192,-0.396410273775032,0.));
#5850=DIRECTION('ref_axis',(0.396410273775032,0.918073469198192,0.));
#5851=DIRECTION('',(0.396410273775032,0.918073469198192,0.));
#5852=DIRECTION('',(0.,0.,1.));
#5853=DIRECTION('',(0.396410273775032,0.918073469198192,0.));
#5854=DIRECTION('center_axis',(0.,0.,-1.));
#5855=DIRECTION('ref_axis',(0.273754622486314,-0.961799566784772,0.));
#5856=DIRECTION('center_axis',(0.,0.,-1.));
#5857=DIRECTION('ref_axis',(0.273754622486314,-0.961799566784772,0.));
#5858=DIRECTION('',(0.,0.,-1.));
#5859=DIRECTION('center_axis',(0.,0.,-1.));
#5860=DIRECTION('ref_axis',(0.273754622486314,-0.961799566784772,0.));
#5861=DIRECTION('',(0.,0.,1.));
#5862=DIRECTION('center_axis',(-0.860332693944512,0.509732925883917,0.));
#5863=DIRECTION('ref_axis',(-0.509732925883917,-0.860332693944512,0.));
#5864=DIRECTION('',(-0.509732925883917,-0.860332693944512,0.));
#5865=DIRECTION('',(0.,0.,1.));
#5866=DIRECTION('',(0.509732925883917,0.860332693944512,0.));
#5867=DIRECTION('center_axis',(0.,0.,1.));
#5868=DIRECTION('ref_axis',(-0.999320575997483,-0.0368562937374282,0.));
#5869=DIRECTION('center_axis',(0.,0.,-1.));
#5870=DIRECTION('ref_axis',(-0.999320575997483,-0.0368562937374282,0.));
#5871=DIRECTION('',(0.,0.,1.));
#5872=DIRECTION('center_axis',(0.,0.,-1.));
#5873=DIRECTION('ref_axis',(-0.999320575997483,-0.0368562937374282,0.));
#5874=DIRECTION('',(0.,0.,-1.));
#5875=DIRECTION('center_axis',(0.750642243977328,-0.660708878067096,0.));
#5876=DIRECTION('ref_axis',(0.660708878067096,0.750642243977328,0.));
#5877=DIRECTION('',(0.660708878067096,0.750642243977328,0.));
#5878=DIRECTION('',(0.,0.,1.));
#5879=DIRECTION('',(0.660708878067096,0.750642243977328,0.));
#5880=DIRECTION('center_axis',(0.,0.,-1.));
#5881=DIRECTION('ref_axis',(-0.0368562937374283,-0.999320575997483,0.));
#5882=DIRECTION('center_axis',(0.,0.,-1.));
#5883=DIRECTION('ref_axis',(-0.0368562937374283,-0.999320575997483,0.));
#5884=DIRECTION('',(0.,0.,-1.));
#5885=DIRECTION('center_axis',(0.,0.,-1.));
#5886=DIRECTION('ref_axis',(-0.0368562937374283,-0.999320575997483,0.));
#5887=DIRECTION('',(0.,0.,1.));
#5888=DIRECTION('center_axis',(-0.660708878067096,0.750642243977328,0.));
#5889=DIRECTION('ref_axis',(-0.750642243977328,-0.660708878067096,0.));
#5890=DIRECTION('',(-0.750642243977328,-0.660708878067096,0.));
#5891=DIRECTION('',(0.,0.,1.));
#5892=DIRECTION('',(0.750642243977328,0.660708878067096,0.));
#5893=DIRECTION('center_axis',(0.,0.,1.));
#5894=DIRECTION('ref_axis',(-0.961799566784773,0.273754622486313,0.));
#5895=DIRECTION('center_axis',(0.,0.,-1.));
#5896=DIRECTION('ref_axis',(-0.961799566784773,0.273754622486313,0.));
#5897=DIRECTION('',(0.,0.,1.));
#5898=DIRECTION('center_axis',(0.,0.,-1.));
#5899=DIRECTION('ref_axis',(-0.961799566784773,0.273754622486313,0.));
#5900=DIRECTION('',(0.,0.,-1.));
#5901=DIRECTION('center_axis',(0.509732925883917,-0.860332693944512,0.));
#5902=DIRECTION('ref_axis',(0.860332693944512,0.509732925883917,0.));
#5903=DIRECTION('',(0.860332693944512,0.509732925883917,0.));
#5904=DIRECTION('',(0.,0.,1.));
#5905=DIRECTION('',(0.860332693944512,0.509732925883917,0.));
#5906=DIRECTION('center_axis',(0.,0.,-1.));
#5907=DIRECTION('ref_axis',(-0.343859459137254,-0.939021124555691,0.));
#5908=DIRECTION('center_axis',(0.,0.,-1.));
#5909=DIRECTION('ref_axis',(-0.343859459137254,-0.939021124555691,0.));
#5910=DIRECTION('',(0.,0.,-1.));
#5911=DIRECTION('center_axis',(0.,0.,-1.));
#5912=DIRECTION('ref_axis',(-0.343859459137254,-0.939021124555691,0.));
#5913=DIRECTION('',(0.,0.,1.));
#5914=DIRECTION('center_axis',(-0.396410273775032,0.918073469198192,0.));
#5915=DIRECTION('ref_axis',(-0.918073469198192,-0.396410273775032,0.));
#5916=DIRECTION('',(-0.918073469198192,-0.396410273775032,0.));
#5917=DIRECTION('',(0.,0.,1.));
#5918=DIRECTION('',(0.918073469198192,0.396410273775032,0.));
#5919=DIRECTION('center_axis',(0.,0.,1.));
#5920=DIRECTION('ref_axis',(-0.830130914723544,0.557568528900486,0.));
#5921=DIRECTION('center_axis',(0.,0.,-1.));
#5922=DIRECTION('ref_axis',(-0.830130914723544,0.557568528900486,0.));
#5923=DIRECTION('',(0.,0.,1.));
#5924=DIRECTION('center_axis',(0.,0.,-1.));
#5925=DIRECTION('ref_axis',(-0.830130914723544,0.557568528900486,0.));
#5926=DIRECTION('',(0.,0.,-1.));
#5927=DIRECTION('center_axis',(0.218927397486859,-0.975741151448288,0.));
#5928=DIRECTION('ref_axis',(0.975741151448288,0.218927397486859,0.));
#5929=DIRECTION('',(0.975741151448288,0.218927397486859,0.));
#5930=DIRECTION('',(0.,0.,1.));
#5931=DIRECTION('',(0.975741151448288,0.218927397486859,0.));
#5932=DIRECTION('',(0.,0.,1.));
#5933=DIRECTION('center_axis',(0.,0.,1.));
#5934=DIRECTION('ref_axis',(0.940823330106451,-0.338897420361099,0.));
#5935=DIRECTION('center_axis',(0.,0.,1.));
#5936=DIRECTION('ref_axis',(0.940823330106451,-0.338897420361099,0.));
#5937=DIRECTION('center_axis',(0.,0.,1.));
#5938=DIRECTION('ref_axis',(0.940823330106451,-0.338897420361099,0.));
#5939=DIRECTION('',(0.,0.,1.));
#5940=DIRECTION('',(0.,0.,1.));
#5941=DIRECTION('center_axis',(0.,0.,1.));
#5942=DIRECTION('ref_axis',(0.790051096538837,-0.613040997697366,0.));
#5943=DIRECTION('center_axis',(0.,0.,1.));
#5944=DIRECTION('ref_axis',(0.790051096538837,-0.613040997697366,0.));
#5945=DIRECTION('center_axis',(0.,0.,1.));
#5946=DIRECTION('ref_axis',(0.790051096538837,-0.613040997697366,0.));
#5947=DIRECTION('',(0.,0.,1.));
#5948=DIRECTION('',(0.,0.,1.));
#5949=DIRECTION('center_axis',(0.,0.,1.));
#5950=DIRECTION('ref_axis',(0.561943157032333,-0.827175850871225,0.));
#5951=DIRECTION('center_axis',(0.,0.,1.));
#5952=DIRECTION('ref_axis',(0.561943157032333,-0.827175850871225,0.));
#5953=DIRECTION('center_axis',(0.,0.,1.));
#5954=DIRECTION('ref_axis',(0.561943157032333,-0.827175850871225,0.));
#5955=DIRECTION('',(0.,0.,1.));
#5956=DIRECTION('',(0.,0.,1.));
#5957=DIRECTION('center_axis',(0.,0.,1.));
#5958=DIRECTION('ref_axis',(0.278828306027306,-0.960340968488767,0.));
#5959=DIRECTION('center_axis',(0.,0.,1.));
#5960=DIRECTION('ref_axis',(0.278828306027306,-0.960340968488767,0.));
#5961=DIRECTION('center_axis',(0.,0.,1.));
#5962=DIRECTION('ref_axis',(0.278828306027306,-0.960340968488767,0.));
#5963=DIRECTION('',(0.,0.,1.));
#5964=DIRECTION('',(0.,0.,1.));
#5965=DIRECTION('center_axis',(0.,0.,1.));
#5966=DIRECTION('ref_axis',(-0.0315802022827165,-0.999501221021657,0.));
#5967=DIRECTION('center_axis',(0.,0.,1.));
#5968=DIRECTION('ref_axis',(-0.0315802022827165,-0.999501221021657,0.));
#5969=DIRECTION('center_axis',(0.,0.,1.));
#5970=DIRECTION('ref_axis',(-0.0315802022827165,-0.999501221021657,0.));
#5971=DIRECTION('',(0.,0.,1.));
#5972=DIRECTION('',(0.,0.,1.));
#5973=DIRECTION('center_axis',(0.,0.,1.));
#5974=DIRECTION('ref_axis',(-0.338897420361099,-0.940823330106451,0.));
#5975=DIRECTION('center_axis',(0.,0.,1.));
#5976=DIRECTION('ref_axis',(-0.338897420361099,-0.940823330106451,0.));
#5977=DIRECTION('center_axis',(0.,0.,1.));
#5978=DIRECTION('ref_axis',(-0.338897420361099,-0.940823330106451,0.));
#5979=DIRECTION('',(0.,0.,1.));
#5980=DIRECTION('',(0.,0.,1.));
#5981=DIRECTION('center_axis',(0.,0.,1.));
#5982=DIRECTION('ref_axis',(-0.613040997697366,-0.790051096538837,0.));
#5983=DIRECTION('center_axis',(0.,0.,1.));
#5984=DIRECTION('ref_axis',(-0.613040997697366,-0.790051096538837,0.));
#5985=DIRECTION('center_axis',(0.,0.,1.));
#5986=DIRECTION('ref_axis',(-0.613040997697366,-0.790051096538837,0.));
#5987=DIRECTION('',(0.,0.,1.));
#5988=DIRECTION('',(0.,0.,1.));
#5989=DIRECTION('center_axis',(0.,0.,1.));
#5990=DIRECTION('ref_axis',(-0.827175850871225,-0.561943157032333,0.));
#5991=DIRECTION('center_axis',(0.,0.,1.));
#5992=DIRECTION('ref_axis',(-0.827175850871225,-0.561943157032333,0.));
#5993=DIRECTION('center_axis',(0.,0.,1.));
#5994=DIRECTION('ref_axis',(-0.827175850871225,-0.561943157032333,0.));
#5995=DIRECTION('',(0.,0.,1.));
#5996=DIRECTION('',(0.,0.,1.));
#5997=DIRECTION('center_axis',(0.,0.,1.));
#5998=DIRECTION('ref_axis',(-0.960340968488767,-0.278828306027306,0.));
#5999=DIRECTION('center_axis',(0.,0.,1.));
#6000=DIRECTION('ref_axis',(-0.960340968488767,-0.278828306027306,0.));
#6001=DIRECTION('center_axis',(0.,0.,1.));
#6002=DIRECTION('ref_axis',(-0.960340968488767,-0.278828306027306,0.));
#6003=DIRECTION('',(0.,0.,1.));
#6004=DIRECTION('',(0.,0.,1.));
#6005=DIRECTION('center_axis',(0.,0.,1.));
#6006=DIRECTION('ref_axis',(-0.999501221021657,0.0315802022827165,0.));
#6007=DIRECTION('center_axis',(0.,0.,1.));
#6008=DIRECTION('ref_axis',(-0.999501221021657,0.0315802022827165,0.));
#6009=DIRECTION('center_axis',(0.,0.,1.));
#6010=DIRECTION('ref_axis',(-0.999501221021657,0.0315802022827165,0.));
#6011=DIRECTION('',(0.,0.,1.));
#6012=DIRECTION('',(0.,0.,1.));
#6013=DIRECTION('center_axis',(0.,0.,1.));
#6014=DIRECTION('ref_axis',(-0.940823330106451,0.338897420361099,0.));
#6015=DIRECTION('center_axis',(0.,0.,1.));
#6016=DIRECTION('ref_axis',(-0.940823330106451,0.338897420361099,0.));
#6017=DIRECTION('center_axis',(0.,0.,1.));
#6018=DIRECTION('ref_axis',(-0.940823330106451,0.338897420361099,0.));
#6019=DIRECTION('',(0.,0.,1.));
#6020=DIRECTION('',(0.,0.,1.));
#6021=DIRECTION('center_axis',(0.,0.,1.));
#6022=DIRECTION('ref_axis',(-0.790051096538837,0.613040997697366,0.));
#6023=DIRECTION('center_axis',(0.,0.,1.));
#6024=DIRECTION('ref_axis',(-0.790051096538837,0.613040997697366,0.));
#6025=DIRECTION('center_axis',(0.,0.,1.));
#6026=DIRECTION('ref_axis',(-0.790051096538837,0.613040997697366,0.));
#6027=DIRECTION('',(0.,0.,1.));
#6028=DIRECTION('',(0.,0.,1.));
#6029=DIRECTION('center_axis',(0.,0.,1.));
#6030=DIRECTION('ref_axis',(-0.561943157032333,0.827175850871225,0.));
#6031=DIRECTION('center_axis',(0.,0.,1.));
#6032=DIRECTION('ref_axis',(-0.561943157032333,0.827175850871225,0.));
#6033=DIRECTION('center_axis',(0.,0.,1.));
#6034=DIRECTION('ref_axis',(-0.561943157032333,0.827175850871225,0.));
#6035=DIRECTION('',(0.,0.,1.));
#6036=DIRECTION('',(0.,0.,1.));
#6037=DIRECTION('center_axis',(0.,0.,1.));
#6038=DIRECTION('ref_axis',(-0.278828306027306,0.960340968488767,0.));
#6039=DIRECTION('center_axis',(0.,0.,1.));
#6040=DIRECTION('ref_axis',(-0.278828306027306,0.960340968488767,0.));
#6041=DIRECTION('center_axis',(0.,0.,1.));
#6042=DIRECTION('ref_axis',(-0.278828306027306,0.960340968488767,0.));
#6043=DIRECTION('',(0.,0.,1.));
#6044=DIRECTION('',(0.,0.,1.));
#6045=DIRECTION('center_axis',(0.,0.,1.));
#6046=DIRECTION('ref_axis',(0.0315802022827164,0.999501221021657,0.));
#6047=DIRECTION('center_axis',(0.,0.,1.));
#6048=DIRECTION('ref_axis',(0.0315802022827164,0.999501221021657,0.));
#6049=DIRECTION('center_axis',(0.,0.,1.));
#6050=DIRECTION('ref_axis',(0.0315802022827164,0.999501221021657,0.));
#6051=DIRECTION('',(0.,0.,1.));
#6052=DIRECTION('',(0.,0.,1.));
#6053=DIRECTION('center_axis',(0.,0.,1.));
#6054=DIRECTION('ref_axis',(0.338897420361099,0.940823330106451,0.));
#6055=DIRECTION('center_axis',(0.,0.,1.));
#6056=DIRECTION('ref_axis',(0.338897420361099,0.940823330106451,0.));
#6057=DIRECTION('center_axis',(0.,0.,1.));
#6058=DIRECTION('ref_axis',(0.338897420361099,0.940823330106451,0.));
#6059=DIRECTION('',(0.,0.,1.));
#6060=DIRECTION('',(0.,0.,1.));
#6061=DIRECTION('center_axis',(0.,0.,1.));
#6062=DIRECTION('ref_axis',(0.613040997697366,0.790051096538837,0.));
#6063=DIRECTION('center_axis',(0.,0.,1.));
#6064=DIRECTION('ref_axis',(0.613040997697366,0.790051096538837,0.));
#6065=DIRECTION('center_axis',(0.,0.,1.));
#6066=DIRECTION('ref_axis',(0.613040997697366,0.790051096538837,0.));
#6067=DIRECTION('',(0.,0.,1.));
#6068=DIRECTION('',(0.,0.,1.));
#6069=DIRECTION('center_axis',(0.,0.,1.));
#6070=DIRECTION('ref_axis',(0.827175850871225,0.561943157032333,0.));
#6071=DIRECTION('center_axis',(0.,0.,1.));
#6072=DIRECTION('ref_axis',(0.827175850871225,0.561943157032333,0.));
#6073=DIRECTION('center_axis',(0.,0.,1.));
#6074=DIRECTION('ref_axis',(0.827175850871225,0.561943157032333,0.));
#6075=DIRECTION('',(0.,0.,1.));
#6076=DIRECTION('',(0.,0.,1.));
#6077=DIRECTION('center_axis',(0.,0.,1.));
#6078=DIRECTION('ref_axis',(0.960340968488767,0.278828306027306,0.));
#6079=DIRECTION('center_axis',(0.,0.,1.));
#6080=DIRECTION('ref_axis',(0.960340968488767,0.278828306027306,0.));
#6081=DIRECTION('center_axis',(0.,0.,1.));
#6082=DIRECTION('ref_axis',(0.960340968488767,0.278828306027306,0.));
#6083=DIRECTION('',(0.,0.,1.));
#6084=DIRECTION('center_axis',(0.,0.,1.));
#6085=DIRECTION('ref_axis',(1.,0.,0.));
#6086=DIRECTION('center_axis',(0.,0.,1.));
#6087=DIRECTION('ref_axis',(1.,0.,0.));
#6088=DIRECTION('center_axis',(0.,0.,1.));
#6089=DIRECTION('ref_axis',(1.,0.,0.));
#6090=DIRECTION('center_axis',(0.,0.,1.));
#6091=DIRECTION('ref_axis',(1.,0.,0.));
#6092=DIRECTION('center_axis',(0.,0.,1.));
#6093=DIRECTION('ref_axis',(1.,0.,0.));
#6094=DIRECTION('center_axis',(0.,0.,1.));
#6095=DIRECTION('ref_axis',(1.,0.,0.));
#6096=DIRECTION('center_axis',(0.,0.,1.));
#6097=DIRECTION('ref_axis',(1.,0.,0.));
#6098=DIRECTION('center_axis',(0.,0.,1.));
#6099=DIRECTION('ref_axis',(1.,0.,0.));
#6100=DIRECTION('center_axis',(0.,0.,1.));
#6101=DIRECTION('ref_axis',(1.,0.,0.));
#6102=DIRECTION('center_axis',(0.,0.,1.));
#6103=DIRECTION('ref_axis',(1.,0.,0.));
#6104=DIRECTION('center_axis',(0.,0.,1.));
#6105=DIRECTION('ref_axis',(1.,0.,0.));
#6106=DIRECTION('center_axis',(0.,0.,1.));
#6107=DIRECTION('ref_axis',(1.,0.,0.));
#6108=DIRECTION('center_axis',(0.,0.,1.));
#6109=DIRECTION('ref_axis',(1.,0.,0.));
#6110=DIRECTION('center_axis',(0.,0.,1.));
#6111=DIRECTION('ref_axis',(1.,0.,0.));
#6112=DIRECTION('center_axis',(0.,0.,1.));
#6113=DIRECTION('ref_axis',(1.,0.,0.));
#6114=DIRECTION('center_axis',(0.,0.,1.));
#6115=DIRECTION('ref_axis',(1.,0.,0.));
#6116=DIRECTION('center_axis',(0.,0.,1.));
#6117=DIRECTION('ref_axis',(1.,0.,0.));
#6118=DIRECTION('center_axis',(0.,0.,1.));
#6119=DIRECTION('ref_axis',(1.,0.,0.));
#6120=DIRECTION('center_axis',(0.,0.,1.));
#6121=DIRECTION('ref_axis',(1.,0.,0.));
#6122=DIRECTION('center_axis',(0.,0.,-1.));
#6123=DIRECTION('ref_axis',(-0.617203264866994,-0.786803742897505,0.));
#6124=DIRECTION('',(0.995637266659949,0.0933082699330836,0.));
#6125=DIRECTION('center_axis',(0.,0.,1.));
#6126=DIRECTION('ref_axis',(0.999501221021657,-0.0315802022827163,0.));
#6127=DIRECTION('',(0.995637266659949,-0.0933082699330836,0.));
#6128=DIRECTION('center_axis',(0.,0.,-1.));
#6129=DIRECTION('ref_axis',(-0.617203264866994,0.786803742897505,0.));
#6130=DIRECTION('center_axis',(0.,0.,1.));
#6131=DIRECTION('ref_axis',(1.,0.,0.));
#6132=DIRECTION('center_axis',(0.,0.,1.));
#6133=DIRECTION('ref_axis',(1.,0.,0.));
#6134=DIRECTION('center_axis',(0.,0.,1.));
#6135=DIRECTION('ref_axis',(1.,0.,0.));
#6136=DIRECTION('center_axis',(0.,0.,1.));
#6137=DIRECTION('ref_axis',(1.,0.,0.));
#6138=DIRECTION('center_axis',(0.,0.,-1.));
#6139=DIRECTION('ref_axis',(-0.617203264866994,0.786803742897505,0.));
#6140=DIRECTION('',(0.995637266659949,-0.0933082699330836,0.));
#6141=DIRECTION('center_axis',(0.,0.,1.));
#6142=DIRECTION('ref_axis',(0.999501221021657,-0.0315802022827163,0.));
#6143=DIRECTION('',(-0.995637266659949,-0.0933082699330836,0.));
#6144=DIRECTION('center_axis',(0.,0.,-1.));
#6145=DIRECTION('ref_axis',(-0.617203264866994,-0.786803742897505,0.));
#6146=DIRECTION('center_axis',(0.,0.,1.));
#6147=DIRECTION('ref_axis',(1.,0.,0.));
#6148=DIRECTION('center_axis',(0.,0.,1.));
#6149=DIRECTION('ref_axis',(1.,0.,0.));
#6150=DIRECTION('center_axis',(0.,0.,1.));
#6151=DIRECTION('ref_axis',(1.,0.,0.));
#6152=DIRECTION('center_axis',(0.,0.,1.));
#6153=DIRECTION('ref_axis',(1.,0.,0.));
#6154=DIRECTION('center_axis',(0.,0.,1.));
#6155=DIRECTION('ref_axis',(1.,0.,0.));
#6156=DIRECTION('center_axis',(0.,0.,1.));
#6157=DIRECTION('ref_axis',(1.,0.,0.));
#6158=DIRECTION('center_axis',(0.,0.,1.));
#6159=DIRECTION('ref_axis',(1.,0.,0.));
#6160=DIRECTION('center_axis',(0.,0.,1.));
#6161=DIRECTION('ref_axis',(1.,0.,0.));
#6162=DIRECTION('center_axis',(0.,0.,1.));
#6163=DIRECTION('ref_axis',(1.,0.,0.));
#6164=DIRECTION('center_axis',(0.,0.,1.));
#6165=DIRECTION('ref_axis',(1.,0.,0.));
#6166=DIRECTION('center_axis',(0.,0.,1.));
#6167=DIRECTION('ref_axis',(1.,0.,0.));
#6168=DIRECTION('center_axis',(0.,0.,1.));
#6169=DIRECTION('ref_axis',(1.,0.,0.));
#6170=DIRECTION('center_axis',(0.,0.,1.));
#6171=DIRECTION('ref_axis',(1.,0.,0.));
#6172=DIRECTION('center_axis',(0.,0.,1.));
#6173=DIRECTION('ref_axis',(1.,0.,0.));
#6174=DIRECTION('center_axis',(0.,0.,1.));
#6175=DIRECTION('ref_axis',(1.,0.,0.));
#6176=DIRECTION('center_axis',(0.,0.,1.));
#6177=DIRECTION('ref_axis',(1.,0.,0.));
#6178=DIRECTION('center_axis',(0.,0.,1.));
#6179=DIRECTION('ref_axis',(1.,0.,0.));
#6180=DIRECTION('center_axis',(0.,0.,1.));
#6181=DIRECTION('ref_axis',(1.,0.,0.));
#6182=DIRECTION('center_axis',(0.,0.,1.));
#6183=DIRECTION('ref_axis',(1.,0.,0.));
#6184=DIRECTION('center_axis',(0.,0.,1.));
#6185=DIRECTION('ref_axis',(1.,0.,0.));
#6186=DIRECTION('',(0.,0.,1.));
#6187=DIRECTION('center_axis',(0.,0.,1.));
#6188=DIRECTION('ref_axis',(1.,0.,0.));
#6189=DIRECTION('center_axis',(0.,0.,1.));
#6190=DIRECTION('ref_axis',(1.,0.,0.));
#6191=DIRECTION('center_axis',(0.,0.,1.));
#6192=DIRECTION('ref_axis',(1.,0.,0.));
#6193=DIRECTION('center_axis',(0.,0.,1.));
#6194=DIRECTION('ref_axis',(1.,0.,0.));
#6195=DIRECTION('center_axis',(0.,0.,1.));
#6196=DIRECTION('ref_axis',(1.,0.,0.));
#6197=DIRECTION('center_axis',(0.,0.,1.));
#6198=DIRECTION('ref_axis',(1.,0.,0.));
#6199=DIRECTION('center_axis',(0.,0.,1.));
#6200=DIRECTION('ref_axis',(1.,0.,0.));
#6201=DIRECTION('center_axis',(0.,0.,1.));
#6202=DIRECTION('ref_axis',(1.,0.,0.));
#6203=DIRECTION('center_axis',(0.,0.,1.));
#6204=DIRECTION('ref_axis',(1.,0.,0.));
#6205=DIRECTION('center_axis',(0.,0.,1.));
#6206=DIRECTION('ref_axis',(1.,0.,0.));
#6207=DIRECTION('center_axis',(0.,0.,1.));
#6208=DIRECTION('ref_axis',(1.,0.,0.));
#6209=DIRECTION('center_axis',(0.,0.,1.));
#6210=DIRECTION('ref_axis',(1.,0.,0.));
#6211=DIRECTION('center_axis',(0.,0.,1.));
#6212=DIRECTION('ref_axis',(1.,0.,0.));
#6213=DIRECTION('center_axis',(0.,0.,1.));
#6214=DIRECTION('ref_axis',(1.,0.,0.));
#6215=DIRECTION('center_axis',(0.,0.,1.));
#6216=DIRECTION('ref_axis',(1.,0.,0.));
#6217=DIRECTION('center_axis',(0.,0.,1.));
#6218=DIRECTION('ref_axis',(1.,0.,0.));
#6219=DIRECTION('center_axis',(0.,0.,1.));
#6220=DIRECTION('ref_axis',(1.,0.,0.));
#6221=DIRECTION('center_axis',(0.,0.,1.));
#6222=DIRECTION('ref_axis',(1.,0.,0.));
#6223=DIRECTION('center_axis',(0.,0.,-1.));
#6224=DIRECTION('ref_axis',(-0.617203264866994,-0.786803742897505,0.));
#6225=DIRECTION('',(0.,0.,-1.));
#6226=DIRECTION('center_axis',(-0.0933082699330836,0.995637266659949,0.));
#6227=DIRECTION('ref_axis',(-0.995637266659949,-0.0933082699330836,0.));
#6228=DIRECTION('',(0.,0.,1.));
#6229=DIRECTION('center_axis',(0.,0.,1.));
#6230=DIRECTION('ref_axis',(-0.617203264866994,0.786803742897505,0.));
#6231=DIRECTION('',(0.,0.,1.));
#6232=DIRECTION('',(0.,0.,-1.));
#6233=DIRECTION('center_axis',(-0.0933082699330836,-0.995637266659949,0.));
#6234=DIRECTION('ref_axis',(0.995637266659949,-0.0933082699330836,0.));
#6235=DIRECTION('',(0.,0.,1.));
#6236=DIRECTION('',(0.,0.,1.));
#6237=DIRECTION('center_axis',(0.,0.,1.));
#6238=DIRECTION('ref_axis',(0.999501221021657,-0.0315802022827163,0.));
#6239=DIRECTION('',(0.,0.,1.));
#6240=DIRECTION('center_axis',(0.,0.,1.));
#6241=DIRECTION('ref_axis',(1.,0.,0.));
#6818=CARTESIAN_POINT('',(0.,0.,0.));
#6819=CARTESIAN_POINT('Origin',(0.,0.,13.));
#6820=CARTESIAN_POINT('',(5.,6.12323399573677E-16,13.));
#6821=CARTESIAN_POINT('Origin',(0.,0.,13.));
#6822=CARTESIAN_POINT('',(5.,6.12323399573677E-16,0.));
#6823=CARTESIAN_POINT('',(5.,-6.12323399573677E-16,13.));
#6824=CARTESIAN_POINT('Origin',(0.,0.,0.));
#6825=CARTESIAN_POINT('Origin',(18.4254989505611,-3.10927393821618,0.));
#6826=CARTESIAN_POINT('',(17.4394399250575,-2.94287803014511,13.));
#6827=CARTESIAN_POINT('',(18.2065715530743,-4.08501508966447,13.));
#6828=CARTESIAN_POINT('Origin',(18.4254989505611,-3.10927393821618,13.));
#6829=CARTESIAN_POINT('',(18.2065715530743,-4.08501508966447,0.));
#6830=CARTESIAN_POINT('',(18.2065715530743,-4.08501508966447,0.));
#6831=CARTESIAN_POINT('',(17.4394399250575,-2.94287803014511,0.));
#6832=CARTESIAN_POINT('Origin',(18.4254989505611,-3.10927393821618,0.));
#6833=CARTESIAN_POINT('',(17.4394399250575,-2.94287803014511,0.));
#6834=CARTESIAN_POINT('Origin',(18.337935196262,-4.11448919812531,0.));
#6835=CARTESIAN_POINT('',(18.337935196262,-4.11448919812531,13.));
#6836=CARTESIAN_POINT('',(9.16896759813102,-2.05724459906266,13.));
#6837=CARTESIAN_POINT('',(18.337935196262,-4.11448919812531,0.));
#6838=CARTESIAN_POINT('',(18.337935196262,-4.11448919812531,0.));
#6839=CARTESIAN_POINT('',(17.2472005929999,-3.86976067797773,0.));
#6840=CARTESIAN_POINT('Origin',(16.7341271470625,-8.31478109308627,0.));
#6841=CARTESIAN_POINT('',(15.8385835771673,-7.8698072574293,0.));
#6842=CARTESIAN_POINT('',(17.1305374208376,-7.39670762388808,0.));
#6843=CARTESIAN_POINT('Origin',(16.7341271470625,-8.31478109308627,0.));
#6844=CARTESIAN_POINT('',(17.1305374208376,-7.39670762388808,13.));
#6845=CARTESIAN_POINT('',(17.1305374208376,-7.39670762388808,0.));
#6846=CARTESIAN_POINT('',(15.8385835771673,-7.8698072574293,13.));
#6847=CARTESIAN_POINT('Origin',(16.7341271470625,-8.31478109308627,13.));
#6848=CARTESIAN_POINT('',(15.8385835771673,-7.8698072574293,0.));
#6849=CARTESIAN_POINT('Origin',(16.2278666415473,-7.00694799924747,0.));
#6850=CARTESIAN_POINT('',(17.2541372868972,-7.45007618140239,0.));
#6851=CARTESIAN_POINT('',(16.2278666415473,-7.00694799924747,0.));
#6852=CARTESIAN_POINT('',(17.2541372868972,-7.45007618140239,13.));
#6853=CARTESIAN_POINT('',(17.2541372868972,-7.45007618140239,0.));
#6854=CARTESIAN_POINT('',(8.11393332077363,-3.50347399962373,13.));
#6855=CARTESIAN_POINT('Origin',(16.5628723558448,-8.65088754544835,0.));
#6856=CARTESIAN_POINT('',(15.6764936575763,-8.18792663645507,13.));
#6857=CARTESIAN_POINT('',(16.0531394299608,-9.51122023939286,13.));
#6858=CARTESIAN_POINT('Origin',(16.5628723558448,-8.65088754544835,13.));
#6859=CARTESIAN_POINT('',(16.0531394299608,-9.51122023939286,0.));
#6860=CARTESIAN_POINT('',(16.0531394299608,-9.51122023939286,0.));
#6861=CARTESIAN_POINT('',(15.6764936575763,-8.18792663645507,0.));
#6862=CARTESIAN_POINT('Origin',(16.5628723558448,-8.65088754544835,0.));
#6863=CARTESIAN_POINT('',(15.6764936575763,-8.18792663645507,0.));
#6864=CARTESIAN_POINT('Origin',(16.1689656784104,-9.57984538049455,0.));
#6865=CARTESIAN_POINT('',(16.1689656784104,-9.57984538049455,13.));
#6866=CARTESIAN_POINT('',(8.08448283920519,-4.78992269024728,13.));
#6867=CARTESIAN_POINT('',(16.1689656784104,-9.57984538049455,0.));
#6868=CARTESIAN_POINT('',(16.1689656784104,-9.57984538049455,0.));
#6869=CARTESIAN_POINT('',(15.2072406981632,-9.01003919792413,0.));
#6870=CARTESIAN_POINT('Origin',(13.3456920054543,-13.0789564146209,0.));
#6871=CARTESIAN_POINT('',(12.6314839349494,-12.3790229663377,0.));
#6872=CARTESIAN_POINT('',(14.0064008835214,-12.3283141706436,0.));
#6873=CARTESIAN_POINT('Origin',(13.3456920054543,-13.0789564146209,0.));
#6874=CARTESIAN_POINT('',(14.0064008835214,-12.3283141706436,13.));
#6875=CARTESIAN_POINT('',(14.0064008835214,-12.3283141706436,0.));
#6876=CARTESIAN_POINT('',(12.6314839349494,-12.3790229663377,13.));
#6877=CARTESIAN_POINT('Origin',(13.3456920054543,-13.0789564146209,13.));
#6878=CARTESIAN_POINT('',(12.6314839349494,-12.3790229663377,0.));
#6879=CARTESIAN_POINT('Origin',(13.2683523045433,-11.678690128714,0.));
#6880=CARTESIAN_POINT('',(14.1074595503134,-12.4172651441477,0.));
#6881=CARTESIAN_POINT('',(13.2683523045433,-11.678690128714,0.));
#6882=CARTESIAN_POINT('',(14.1074595503134,-12.4172651441477,13.));
#6883=CARTESIAN_POINT('',(14.1074595503134,-12.4172651441477,0.));
#6884=CARTESIAN_POINT('',(6.63417615227163,-5.839345064357,13.));
#6885=CARTESIAN_POINT('Origin',(13.0789564146209,-13.3456920054543,0.));
#6886=CARTESIAN_POINT('',(12.3790229663377,-12.6314839349494,13.));
#6887=CARTESIAN_POINT('',(12.3283141706436,-14.0064008835214,13.));
#6888=CARTESIAN_POINT('Origin',(13.0789564146209,-13.3456920054543,13.));
#6889=CARTESIAN_POINT('',(12.3283141706436,-14.0064008835214,0.));
#6890=CARTESIAN_POINT('',(12.3283141706436,-14.0064008835214,0.));
#6891=CARTESIAN_POINT('',(12.3790229663377,-12.6314839349494,0.));
#6892=CARTESIAN_POINT('Origin',(13.0789564146209,-13.3456920054543,0.));
#6893=CARTESIAN_POINT('',(12.3790229663377,-12.6314839349494,0.));
#6894=CARTESIAN_POINT('Origin',(12.4172651441477,-14.1074595503134,0.));
#6895=CARTESIAN_POINT('',(12.4172651441477,-14.1074595503134,13.));
#6896=CARTESIAN_POINT('',(6.20863257207386,-7.05372977515671,13.));
#6897=CARTESIAN_POINT('',(12.4172651441477,-14.1074595503134,0.));
#6898=CARTESIAN_POINT('',(12.4172651441477,-14.1074595503134,0.));
#6899=CARTESIAN_POINT('',(11.678690128714,-13.2683523045433,0.));
#6900=CARTESIAN_POINT('Origin',(8.65088754544834,-16.5628723558448,0.));
#6901=CARTESIAN_POINT('',(8.18792663645507,-15.6764936575763,0.));
#6902=CARTESIAN_POINT('',(9.51122023939285,-16.0531394299608,0.));
#6903=CARTESIAN_POINT('Origin',(8.65088754544834,-16.5628723558448,0.));
#6904=CARTESIAN_POINT('',(9.51122023939285,-16.0531394299608,13.));
#6905=CARTESIAN_POINT('',(9.51122023939285,-16.0531394299608,0.));
#6906=CARTESIAN_POINT('',(8.18792663645507,-15.6764936575763,13.));
#6907=CARTESIAN_POINT('Origin',(8.65088754544834,-16.5628723558448,13.));
#6908=CARTESIAN_POINT('',(8.18792663645507,-15.6764936575763,0.));
#6909=CARTESIAN_POINT('Origin',(9.01003919792412,-15.2072406981632,0.));
#6910=CARTESIAN_POINT('',(9.57984538049454,-16.1689656784104,0.));
#6911=CARTESIAN_POINT('',(9.01003919792412,-15.2072406981632,0.));
#6912=CARTESIAN_POINT('',(9.57984538049454,-16.1689656784104,13.));
#6913=CARTESIAN_POINT('',(9.57984538049454,-16.1689656784104,0.));
#6914=CARTESIAN_POINT('',(4.50501959896206,-7.6036203490816,13.));
#6915=CARTESIAN_POINT('Origin',(8.31478109308627,-16.7341271470625,0.));
#6916=CARTESIAN_POINT('',(7.86980725742929,-15.8385835771673,13.));
#6917=CARTESIAN_POINT('',(7.39670762388807,-17.1305374208376,13.));
#6918=CARTESIAN_POINT('Origin',(8.31478109308627,-16.7341271470625,13.));
#6919=CARTESIAN_POINT('',(7.39670762388807,-17.1305374208376,0.));
#6920=CARTESIAN_POINT('',(7.39670762388807,-17.1305374208376,0.));
#6921=CARTESIAN_POINT('',(7.86980725742929,-15.8385835771673,0.));
#6922=CARTESIAN_POINT('Origin',(8.31478109308627,-16.7341271470625,0.));
#6923=CARTESIAN_POINT('',(7.86980725742929,-15.8385835771673,0.));
#6924=CARTESIAN_POINT('Origin',(7.45007618140238,-17.2541372868972,0.));
#6925=CARTESIAN_POINT('',(7.45007618140238,-17.2541372868972,13.));
#6926=CARTESIAN_POINT('',(3.72503809070119,-8.62706864344861,13.));
#6927=CARTESIAN_POINT('',(7.45007618140238,-17.2541372868972,0.));
#6928=CARTESIAN_POINT('',(7.45007618140238,-17.2541372868972,0.));
#6929=CARTESIAN_POINT('',(7.00694799924746,-16.2278666415473,0.));
#6930=CARTESIAN_POINT('Origin',(3.10927393821617,-18.4254989505611,0.));
#6931=CARTESIAN_POINT('',(2.9428780301451,-17.4394399250575,0.));
#6932=CARTESIAN_POINT('',(4.08501508966446,-18.2065715530743,0.));
#6933=CARTESIAN_POINT('Origin',(3.10927393821617,-18.4254989505611,0.));
#6934=CARTESIAN_POINT('',(4.08501508966446,-18.2065715530743,13.));
#6935=CARTESIAN_POINT('',(4.08501508966446,-18.2065715530743,0.));
#6936=CARTESIAN_POINT('',(2.9428780301451,-17.4394399250575,13.));
#6937=CARTESIAN_POINT('Origin',(3.10927393821617,-18.4254989505611,13.));
#6938=CARTESIAN_POINT('',(2.9428780301451,-17.4394399250575,0.));
#6939=CARTESIAN_POINT('Origin',(3.86976067797772,-17.2472005929999,0.));
#6940=CARTESIAN_POINT('',(4.1144891981253,-18.337935196262,0.));
#6941=CARTESIAN_POINT('',(3.86976067797772,-17.2472005929999,0.));
#6942=CARTESIAN_POINT('',(4.1144891981253,-18.337935196262,13.));
#6943=CARTESIAN_POINT('',(4.1144891981253,-18.337935196262,0.));
#6944=CARTESIAN_POINT('',(1.93488033898886,-8.62360029649997,13.));
#6945=CARTESIAN_POINT('Origin',(2.73669706567396,-18.4845093299966,0.));
#6946=CARTESIAN_POINT('',(2.59023998199238,-17.4952923049513,13.));
#6947=CARTESIAN_POINT('',(1.741059799014,-18.5778175999297,13.));
#6948=CARTESIAN_POINT('Origin',(2.73669706567396,-18.4845093299966,13.));
#6949=CARTESIAN_POINT('',(1.741059799014,-18.5778175999297,0.));
#6950=CARTESIAN_POINT('',(1.741059799014,-18.5778175999297,0.));
#6951=CARTESIAN_POINT('',(2.59023998199238,-17.4952923049513,0.));
#6952=CARTESIAN_POINT('Origin',(2.73669706567396,-18.4845093299966,0.));
#6953=CARTESIAN_POINT('',(2.59023998199238,-17.4952923049513,0.));
#6954=CARTESIAN_POINT('Origin',(1.75362185428836,-18.7118598491961,0.));
#6955=CARTESIAN_POINT('',(1.75362185428836,-18.7118598491961,13.));
#6956=CARTESIAN_POINT('',(0.876810927144179,-9.35592992459806,13.));
#6957=CARTESIAN_POINT('',(1.75362185428836,-18.7118598491961,0.));
#6958=CARTESIAN_POINT('',(1.75362185428836,-18.7118598491961,0.));
#6959=CARTESIAN_POINT('',(1.64931697933718,-17.5988843254813,0.));
#6960=CARTESIAN_POINT('Origin',(-2.73669706567396,-18.4845093299966,0.));
#6961=CARTESIAN_POINT('',(-2.59023998199239,-17.4952923049513,0.));
#6962=CARTESIAN_POINT('',(-1.74105979901401,-18.5778175999297,0.));
#6963=CARTESIAN_POINT('Origin',(-2.73669706567396,-18.4845093299966,0.));
#6964=CARTESIAN_POINT('',(-1.74105979901401,-18.5778175999297,13.));
#6965=CARTESIAN_POINT('',(-1.74105979901401,-18.5778175999297,0.));
#6966=CARTESIAN_POINT('',(-2.59023998199239,-17.4952923049513,13.));
#6967=CARTESIAN_POINT('Origin',(-2.73669706567396,-18.4845093299966,13.));
#6968=CARTESIAN_POINT('',(-2.59023998199239,-17.4952923049513,0.));
#6969=CARTESIAN_POINT('Origin',(-1.64931697933719,-17.5988843254813,0.));
#6970=CARTESIAN_POINT('',(-1.75362185428837,-18.7118598491961,0.));
#6971=CARTESIAN_POINT('',(-1.64931697933719,-17.5988843254813,0.));
#6972=CARTESIAN_POINT('',(-1.75362185428837,-18.7118598491961,13.));
#6973=CARTESIAN_POINT('',(-1.75362185428837,-18.7118598491961,0.));
#6974=CARTESIAN_POINT('',(-0.824658489668592,-8.79944216274063,13.));
#6975=CARTESIAN_POINT('Origin',(-3.10927393821618,-18.4254989505611,0.));
#6976=CARTESIAN_POINT('',(-2.94287803014511,-17.4394399250575,13.));
#6977=CARTESIAN_POINT('',(-4.08501508966447,-18.2065715530743,13.));
#6978=CARTESIAN_POINT('Origin',(-3.10927393821618,-18.4254989505611,13.));
#6979=CARTESIAN_POINT('',(-4.08501508966447,-18.2065715530743,0.));
#6980=CARTESIAN_POINT('',(-4.08501508966447,-18.2065715530743,0.));
#6981=CARTESIAN_POINT('',(-2.94287803014511,-17.4394399250575,0.));
#6982=CARTESIAN_POINT('Origin',(-3.10927393821618,-18.4254989505611,0.));
#6983=CARTESIAN_POINT('',(-2.94287803014511,-17.4394399250575,0.));
#6984=CARTESIAN_POINT('Origin',(-4.11448919812531,-18.337935196262,0.));
#6985=CARTESIAN_POINT('',(-4.11448919812531,-18.337935196262,13.));
#6986=CARTESIAN_POINT('',(-2.05724459906266,-9.16896759813102,13.));
#6987=CARTESIAN_POINT('',(-4.11448919812531,-18.337935196262,0.));
#6988=CARTESIAN_POINT('',(-4.11448919812531,-18.337935196262,0.));
#6989=CARTESIAN_POINT('',(-3.86976067797773,-17.2472005929999,0.));
#6990=CARTESIAN_POINT('Origin',(-8.31478109308627,-16.7341271470625,0.));
#6991=CARTESIAN_POINT('',(-7.86980725742929,-15.8385835771673,0.));
#6992=CARTESIAN_POINT('',(-7.39670762388808,-17.1305374208376,0.));
#6993=CARTESIAN_POINT('Origin',(-8.31478109308627,-16.7341271470625,0.));
#6994=CARTESIAN_POINT('',(-7.39670762388808,-17.1305374208376,13.));
#6995=CARTESIAN_POINT('',(-7.39670762388808,-17.1305374208376,0.));
#6996=CARTESIAN_POINT('',(-7.86980725742929,-15.8385835771673,13.));
#6997=CARTESIAN_POINT('Origin',(-8.31478109308627,-16.7341271470625,13.));
#6998=CARTESIAN_POINT('',(-7.86980725742929,-15.8385835771673,0.));
#6999=CARTESIAN_POINT('Origin',(-7.00694799924747,-16.2278666415473,0.));
#7000=CARTESIAN_POINT('',(-7.45007618140239,-17.2541372868972,0.));
#7001=CARTESIAN_POINT('',(-7.00694799924747,-16.2278666415473,0.));
#7002=CARTESIAN_POINT('',(-7.45007618140239,-17.2541372868972,13.));
#7003=CARTESIAN_POINT('',(-7.45007618140239,-17.2541372868972,0.));
#7004=CARTESIAN_POINT('',(-3.50347399962373,-8.11393332077363,13.));
#7005=CARTESIAN_POINT('Origin',(-8.65088754544835,-16.5628723558448,0.));
#7006=CARTESIAN_POINT('',(-8.18792663645507,-15.6764936575763,13.));
#7007=CARTESIAN_POINT('',(-9.51122023939286,-16.0531394299608,13.));
#7008=CARTESIAN_POINT('Origin',(-8.65088754544835,-16.5628723558448,13.));
#7009=CARTESIAN_POINT('',(-9.51122023939286,-16.0531394299608,0.));
#7010=CARTESIAN_POINT('',(-9.51122023939286,-16.0531394299608,0.));
#7011=CARTESIAN_POINT('',(-8.18792663645507,-15.6764936575763,0.));
#7012=CARTESIAN_POINT('Origin',(-8.65088754544835,-16.5628723558448,0.));
#7013=CARTESIAN_POINT('',(-8.18792663645507,-15.6764936575763,0.));
#7014=CARTESIAN_POINT('Origin',(-9.57984538049455,-16.1689656784104,0.));
#7015=CARTESIAN_POINT('',(-9.57984538049455,-16.1689656784104,13.));
#7016=CARTESIAN_POINT('',(-4.78992269024728,-8.08448283920519,13.));
#7017=CARTESIAN_POINT('',(-9.57984538049455,-16.1689656784104,0.));
#7018=CARTESIAN_POINT('',(-9.57984538049455,-16.1689656784104,0.));
#7019=CARTESIAN_POINT('',(-9.01003919792412,-15.2072406981632,0.));
#7020=CARTESIAN_POINT('Origin',(-13.0789564146209,-13.3456920054543,0.));
#7021=CARTESIAN_POINT('',(-12.3790229663377,-12.6314839349494,0.));
#7022=CARTESIAN_POINT('',(-12.3283141706436,-14.0064008835214,0.));
#7023=CARTESIAN_POINT('Origin',(-13.0789564146209,-13.3456920054543,0.));
#7024=CARTESIAN_POINT('',(-12.3283141706436,-14.0064008835214,13.));
#7025=CARTESIAN_POINT('',(-12.3283141706436,-14.0064008835214,0.));
#7026=CARTESIAN_POINT('',(-12.3790229663377,-12.6314839349494,13.));
#7027=CARTESIAN_POINT('Origin',(-13.0789564146209,-13.3456920054543,13.));
#7028=CARTESIAN_POINT('',(-12.3790229663377,-12.6314839349494,0.));
#7029=CARTESIAN_POINT('Origin',(-11.678690128714,-13.2683523045433,0.));
#7030=CARTESIAN_POINT('',(-12.4172651441477,-14.1074595503134,0.));
#7031=CARTESIAN_POINT('',(-11.678690128714,-13.2683523045433,0.));
#7032=CARTESIAN_POINT('',(-12.4172651441477,-14.1074595503134,13.));
#7033=CARTESIAN_POINT('',(-12.4172651441477,-14.1074595503134,0.));
#7034=CARTESIAN_POINT('',(-5.83934506435699,-6.63417615227163,13.));
#7035=CARTESIAN_POINT('Origin',(-13.3456920054543,-13.0789564146209,0.));
#7036=CARTESIAN_POINT('',(-12.6314839349494,-12.3790229663377,13.));
#7037=CARTESIAN_POINT('',(-14.0064008835214,-12.3283141706436,13.));
#7038=CARTESIAN_POINT('Origin',(-13.3456920054543,-13.0789564146209,13.));
#7039=CARTESIAN_POINT('',(-14.0064008835214,-12.3283141706436,0.));
#7040=CARTESIAN_POINT('',(-14.0064008835214,-12.3283141706436,0.));
#7041=CARTESIAN_POINT('',(-12.6314839349494,-12.3790229663377,0.));
#7042=CARTESIAN_POINT('Origin',(-13.3456920054543,-13.0789564146209,0.));
#7043=CARTESIAN_POINT('',(-12.6314839349494,-12.3790229663377,0.));
#7044=CARTESIAN_POINT('Origin',(-14.1074595503134,-12.4172651441477,0.));
#7045=CARTESIAN_POINT('',(-14.1074595503134,-12.4172651441477,13.));
#7046=CARTESIAN_POINT('',(-7.05372977515671,-6.20863257207387,13.));
#7047=CARTESIAN_POINT('',(-14.1074595503134,-12.4172651441477,0.));
#7048=CARTESIAN_POINT('',(-14.1074595503134,-12.4172651441477,0.));
#7049=CARTESIAN_POINT('',(-13.2683523045433,-11.678690128714,0.));
#7050=CARTESIAN_POINT('Origin',(-16.5628723558448,-8.65088754544834,0.));
#7051=CARTESIAN_POINT('',(-15.6764936575763,-8.18792663645507,0.));
#7052=CARTESIAN_POINT('',(-16.0531394299608,-9.51122023939286,0.));
#7053=CARTESIAN_POINT('Origin',(-16.5628723558448,-8.65088754544834,0.));
#7054=CARTESIAN_POINT('',(-16.0531394299608,-9.51122023939286,13.));
#7055=CARTESIAN_POINT('',(-16.0531394299608,-9.51122023939286,0.));
#7056=CARTESIAN_POINT('',(-15.6764936575763,-8.18792663645507,13.));
#7057=CARTESIAN_POINT('Origin',(-16.5628723558448,-8.65088754544834,13.));
#7058=CARTESIAN_POINT('',(-15.6764936575763,-8.18792663645507,0.));
#7059=CARTESIAN_POINT('Origin',(-15.2072406981632,-9.01003919792412,0.));
#7060=CARTESIAN_POINT('',(-16.1689656784104,-9.57984538049455,0.));
#7061=CARTESIAN_POINT('',(-15.2072406981632,-9.01003919792412,0.));
#7062=CARTESIAN_POINT('',(-16.1689656784104,-9.57984538049455,13.));
#7063=CARTESIAN_POINT('',(-16.1689656784104,-9.57984538049455,0.));
#7064=CARTESIAN_POINT('',(-7.6036203490816,-4.50501959896206,13.));
#7065=CARTESIAN_POINT('Origin',(-16.7341271470625,-8.31478109308626,0.));
#7066=CARTESIAN_POINT('',(-15.8385835771673,-7.86980725742929,13.));
#7067=CARTESIAN_POINT('',(-17.1305374208376,-7.39670762388807,13.));
#7068=CARTESIAN_POINT('Origin',(-16.7341271470625,-8.31478109308626,13.));
#7069=CARTESIAN_POINT('',(-17.1305374208376,-7.39670762388807,0.));
#7070=CARTESIAN_POINT('',(-17.1305374208376,-7.39670762388807,0.));
#7071=CARTESIAN_POINT('',(-15.8385835771673,-7.86980725742929,0.));
#7072=CARTESIAN_POINT('Origin',(-16.7341271470625,-8.31478109308626,0.));
#7073=CARTESIAN_POINT('',(-15.8385835771673,-7.86980725742929,0.));
#7074=CARTESIAN_POINT('Origin',(-17.2541372868972,-7.45007618140238,0.));
#7075=CARTESIAN_POINT('',(-17.2541372868972,-7.45007618140238,13.));
#7076=CARTESIAN_POINT('',(-8.62706864344861,-3.72503809070119,13.));
#7077=CARTESIAN_POINT('',(-17.2541372868972,-7.45007618140238,0.));
#7078=CARTESIAN_POINT('',(-17.2541372868972,-7.45007618140238,0.));
#7079=CARTESIAN_POINT('',(-16.2278666415473,-7.00694799924746,0.));
#7080=CARTESIAN_POINT('Origin',(-18.4254989505611,-3.10927393821617,0.));
#7081=CARTESIAN_POINT('',(-17.4394399250575,-2.94287803014509,0.));
#7082=CARTESIAN_POINT('',(-18.2065715530743,-4.08501508966446,0.));
#7083=CARTESIAN_POINT('Origin',(-18.4254989505611,-3.10927393821617,0.));
#7084=CARTESIAN_POINT('',(-18.2065715530743,-4.08501508966447,13.));
#7085=CARTESIAN_POINT('',(-18.2065715530743,-4.08501508966447,0.));
#7086=CARTESIAN_POINT('',(-17.4394399250575,-2.94287803014509,13.));
#7087=CARTESIAN_POINT('Origin',(-18.4254989505611,-3.10927393821617,13.));
#7088=CARTESIAN_POINT('',(-17.4394399250575,-2.94287803014509,0.));
#7089=CARTESIAN_POINT('Origin',(-17.2472005929999,-3.86976067797772,0.));
#7090=CARTESIAN_POINT('',(-18.337935196262,-4.1144891981253,0.));
#7091=CARTESIAN_POINT('',(-17.2472005929999,-3.86976067797772,0.));
#7092=CARTESIAN_POINT('',(-18.337935196262,-4.1144891981253,13.));
#7093=CARTESIAN_POINT('',(-18.337935196262,-4.1144891981253,0.));
#7094=CARTESIAN_POINT('',(-8.62360029649997,-1.93488033898886,13.));
#7095=CARTESIAN_POINT('Origin',(-18.4845093299966,-2.73669706567395,0.));
#7096=CARTESIAN_POINT('',(-17.4952923049513,-2.59023998199238,13.));
#7097=CARTESIAN_POINT('',(-18.5778175999297,-1.74105979901401,13.));
#7098=CARTESIAN_POINT('Origin',(-18.4845093299966,-2.73669706567395,13.));
#7099=CARTESIAN_POINT('',(-18.5778175999297,-1.74105979901401,0.));
#7100=CARTESIAN_POINT('',(-18.5778175999297,-1.74105979901401,0.));
#7101=CARTESIAN_POINT('',(-17.4952923049513,-2.59023998199238,0.));
#7102=CARTESIAN_POINT('Origin',(-18.4845093299966,-2.73669706567395,0.));
#7103=CARTESIAN_POINT('',(-17.4952923049513,-2.59023998199238,0.));
#7104=CARTESIAN_POINT('Origin',(-18.7118598491961,-1.75362185428836,0.));
#7105=CARTESIAN_POINT('',(-18.7118598491961,-1.75362185428836,13.));
#7106=CARTESIAN_POINT('',(-9.35592992459806,-0.87681092714418,13.));
#7107=CARTESIAN_POINT('',(-18.7118598491961,-1.75362185428836,0.));
#7108=CARTESIAN_POINT('',(-18.7118598491961,-1.75362185428836,0.));
#7109=CARTESIAN_POINT('',(-17.5988843254813,-1.64931697933718,0.));
#7110=CARTESIAN_POINT('Origin',(-18.4845093299966,2.73669706567396,0.));
#7111=CARTESIAN_POINT('',(-17.4952923049513,2.59023998199238,0.));
#7112=CARTESIAN_POINT('',(-18.5778175999297,1.74105979901401,0.));
#7113=CARTESIAN_POINT('Origin',(-18.4845093299966,2.73669706567396,0.));
#7114=CARTESIAN_POINT('',(-18.5778175999297,1.74105979901401,13.));
#7115=CARTESIAN_POINT('',(-18.5778175999297,1.74105979901401,0.));
#7116=CARTESIAN_POINT('',(-17.4952923049513,2.59023998199238,13.));
#7117=CARTESIAN_POINT('Origin',(-18.4845093299966,2.73669706567396,13.));
#7118=CARTESIAN_POINT('',(-17.4952923049513,2.59023998199238,0.));
#7119=CARTESIAN_POINT('Origin',(-17.5988843254813,1.64931697933719,0.));
#7120=CARTESIAN_POINT('',(-18.7118598491961,1.75362185428837,0.));
#7121=CARTESIAN_POINT('',(-17.5988843254813,1.64931697933719,0.));
#7122=CARTESIAN_POINT('',(-18.7118598491961,1.75362185428837,13.));
#7123=CARTESIAN_POINT('',(-18.7118598491961,1.75362185428837,0.));
#7124=CARTESIAN_POINT('',(-8.79944216274063,0.824658489668592,13.));
#7125=CARTESIAN_POINT('Origin',(-18.4254989505611,3.10927393821618,0.));
#7126=CARTESIAN_POINT('',(-17.4394399250575,2.9428780301451,13.));
#7127=CARTESIAN_POINT('',(-18.2065715530743,4.08501508966447,13.));
#7128=CARTESIAN_POINT('Origin',(-18.4254989505611,3.10927393821618,13.));
#7129=CARTESIAN_POINT('',(-18.2065715530743,4.08501508966447,0.));
#7130=CARTESIAN_POINT('',(-18.2065715530743,4.08501508966447,0.));
#7131=CARTESIAN_POINT('',(-17.4394399250575,2.9428780301451,0.));
#7132=CARTESIAN_POINT('Origin',(-18.4254989505611,3.10927393821618,0.));
#7133=CARTESIAN_POINT('',(-17.4394399250575,2.9428780301451,0.));
#7134=CARTESIAN_POINT('Origin',(-18.337935196262,4.11448919812531,0.));
#7135=CARTESIAN_POINT('',(-18.337935196262,4.11448919812531,13.));
#7136=CARTESIAN_POINT('',(-9.16896759813102,2.05724459906266,13.));
#7137=CARTESIAN_POINT('',(-18.337935196262,4.11448919812531,0.));
#7138=CARTESIAN_POINT('',(-18.337935196262,4.11448919812531,0.));
#7139=CARTESIAN_POINT('',(-17.2472005929999,3.86976067797773,0.));
#7140=CARTESIAN_POINT('Origin',(-16.7341271470625,8.31478109308627,0.));
#7141=CARTESIAN_POINT('',(-15.8385835771673,7.86980725742929,0.));
#7142=CARTESIAN_POINT('',(-17.1305374208376,7.39670762388808,0.));
#7143=CARTESIAN_POINT('Origin',(-16.7341271470625,8.31478109308627,0.));
#7144=CARTESIAN_POINT('',(-17.1305374208376,7.39670762388807,13.));
#7145=CARTESIAN_POINT('',(-17.1305374208376,7.39670762388807,0.));
#7146=CARTESIAN_POINT('',(-15.8385835771673,7.86980725742929,13.));
#7147=CARTESIAN_POINT('Origin',(-16.7341271470625,8.31478109308627,13.));
#7148=CARTESIAN_POINT('',(-15.8385835771673,7.86980725742929,0.));
#7149=CARTESIAN_POINT('Origin',(-16.2278666415473,7.00694799924746,0.));
#7150=CARTESIAN_POINT('',(-17.2541372868972,7.45007618140238,0.));
#7151=CARTESIAN_POINT('',(-16.2278666415473,7.00694799924746,0.));
#7152=CARTESIAN_POINT('',(-17.2541372868972,7.45007618140238,13.));
#7153=CARTESIAN_POINT('',(-17.2541372868972,7.45007618140238,0.));
#7154=CARTESIAN_POINT('',(-8.11393332077363,3.50347399962373,13.));
#7155=CARTESIAN_POINT('Origin',(-16.5628723558448,8.65088754544834,0.));
#7156=CARTESIAN_POINT('',(-15.6764936575763,8.18792663645507,13.));
#7157=CARTESIAN_POINT('',(-16.0531394299608,9.51122023939286,13.));
#7158=CARTESIAN_POINT('Origin',(-16.5628723558448,8.65088754544834,13.));
#7159=CARTESIAN_POINT('',(-16.0531394299608,9.51122023939286,0.));
#7160=CARTESIAN_POINT('',(-16.0531394299608,9.51122023939286,0.));
#7161=CARTESIAN_POINT('',(-15.6764936575763,8.18792663645507,0.));
#7162=CARTESIAN_POINT('Origin',(-16.5628723558448,8.65088754544834,0.));
#7163=CARTESIAN_POINT('',(-15.6764936575763,8.18792663645507,0.));
#7164=CARTESIAN_POINT('Origin',(-16.1689656784104,9.57984538049455,0.));
#7165=CARTESIAN_POINT('',(-16.1689656784104,9.57984538049455,13.));
#7166=CARTESIAN_POINT('',(-8.08448283920519,4.78992269024728,13.));
#7167=CARTESIAN_POINT('',(-16.1689656784104,9.57984538049455,0.));
#7168=CARTESIAN_POINT('',(-16.1689656784104,9.57984538049455,0.));
#7169=CARTESIAN_POINT('',(-15.2072406981632,9.01003919792412,0.));
#7170=CARTESIAN_POINT('Origin',(-13.3456920054543,13.0789564146209,0.));
#7171=CARTESIAN_POINT('',(-12.6314839349494,12.3790229663377,0.));
#7172=CARTESIAN_POINT('',(-14.0064008835214,12.3283141706436,0.));
#7173=CARTESIAN_POINT('Origin',(-13.3456920054543,13.0789564146209,0.));
#7174=CARTESIAN_POINT('',(-14.0064008835214,12.3283141706436,13.));
#7175=CARTESIAN_POINT('',(-14.0064008835214,12.3283141706436,0.));
#7176=CARTESIAN_POINT('',(-12.6314839349494,12.3790229663377,13.));
#7177=CARTESIAN_POINT('Origin',(-13.3456920054543,13.0789564146209,13.));
#7178=CARTESIAN_POINT('',(-12.6314839349494,12.3790229663377,0.));
#7179=CARTESIAN_POINT('Origin',(-13.2683523045433,11.678690128714,0.));
#7180=CARTESIAN_POINT('',(-14.1074595503134,12.4172651441477,0.));
#7181=CARTESIAN_POINT('',(-13.2683523045433,11.678690128714,0.));
#7182=CARTESIAN_POINT('',(-14.1074595503134,12.4172651441477,13.));
#7183=CARTESIAN_POINT('',(-14.1074595503134,12.4172651441477,0.));
#7184=CARTESIAN_POINT('',(-6.63417615227163,5.83934506435699,13.));
#7185=CARTESIAN_POINT('Origin',(-13.0789564146209,13.3456920054543,0.));
#7186=CARTESIAN_POINT('',(-12.3790229663377,12.6314839349494,13.));
#7187=CARTESIAN_POINT('',(-12.3283141706436,14.0064008835214,13.));
#7188=CARTESIAN_POINT('Origin',(-13.0789564146209,13.3456920054543,13.));
#7189=CARTESIAN_POINT('',(-12.3283141706436,14.0064008835214,0.));
#7190=CARTESIAN_POINT('',(-12.3283141706436,14.0064008835214,0.));
#7191=CARTESIAN_POINT('',(-12.3790229663377,12.6314839349494,0.));
#7192=CARTESIAN_POINT('Origin',(-13.0789564146209,13.3456920054543,0.));
#7193=CARTESIAN_POINT('',(-12.3790229663377,12.6314839349494,0.));
#7194=CARTESIAN_POINT('Origin',(-12.4172651441477,14.1074595503134,0.));
#7195=CARTESIAN_POINT('',(-12.4172651441477,14.1074595503134,13.));
#7196=CARTESIAN_POINT('',(-6.20863257207387,7.05372977515671,13.));
#7197=CARTESIAN_POINT('',(-12.4172651441477,14.1074595503134,0.));
#7198=CARTESIAN_POINT('',(-12.4172651441477,14.1074595503134,0.));
#7199=CARTESIAN_POINT('',(-11.678690128714,13.2683523045433,0.));
#7200=CARTESIAN_POINT('Origin',(-8.65088754544834,16.5628723558448,0.));
#7201=CARTESIAN_POINT('',(-8.18792663645507,15.6764936575763,0.));
#7202=CARTESIAN_POINT('',(-9.51122023939285,16.0531394299608,0.));
#7203=CARTESIAN_POINT('Origin',(-8.65088754544834,16.5628723558448,0.));
#7204=CARTESIAN_POINT('',(-9.51122023939285,16.0531394299608,13.));
#7205=CARTESIAN_POINT('',(-9.51122023939285,16.0531394299608,0.));
#7206=CARTESIAN_POINT('',(-8.18792663645507,15.6764936575763,13.));
#7207=CARTESIAN_POINT('Origin',(-8.65088754544834,16.5628723558448,13.));
#7208=CARTESIAN_POINT('',(-8.18792663645507,15.6764936575763,0.));
#7209=CARTESIAN_POINT('Origin',(-9.01003919792412,15.2072406981632,0.));
#7210=CARTESIAN_POINT('',(-9.57984538049455,16.1689656784104,0.));
#7211=CARTESIAN_POINT('',(-9.01003919792412,15.2072406981632,0.));
#7212=CARTESIAN_POINT('',(-9.57984538049455,16.1689656784104,13.));
#7213=CARTESIAN_POINT('',(-9.57984538049455,16.1689656784104,0.));
#7214=CARTESIAN_POINT('',(-4.50501959896206,7.6036203490816,13.));
#7215=CARTESIAN_POINT('Origin',(-8.31478109308627,16.7341271470625,0.));
#7216=CARTESIAN_POINT('',(-7.86980725742929,15.8385835771673,13.));
#7217=CARTESIAN_POINT('',(-7.39670762388807,17.1305374208376,13.));
#7218=CARTESIAN_POINT('Origin',(-8.31478109308627,16.7341271470625,13.));
#7219=CARTESIAN_POINT('',(-7.39670762388807,17.1305374208376,0.));
#7220=CARTESIAN_POINT('',(-7.39670762388807,17.1305374208376,0.));
#7221=CARTESIAN_POINT('',(-7.86980725742929,15.8385835771673,0.));
#7222=CARTESIAN_POINT('Origin',(-8.31478109308627,16.7341271470625,0.));
#7223=CARTESIAN_POINT('',(-7.86980725742929,15.8385835771673,0.));
#7224=CARTESIAN_POINT('Origin',(-7.45007618140238,17.2541372868972,0.));
#7225=CARTESIAN_POINT('',(-7.45007618140238,17.2541372868972,13.));
#7226=CARTESIAN_POINT('',(-3.72503809070119,8.62706864344861,13.));
#7227=CARTESIAN_POINT('',(-7.45007618140238,17.2541372868972,0.));
#7228=CARTESIAN_POINT('',(-7.45007618140238,17.2541372868972,0.));
#7229=CARTESIAN_POINT('',(-7.00694799924746,16.2278666415473,0.));
#7230=CARTESIAN_POINT('Origin',(-3.10927393821618,18.4254989505611,0.));
#7231=CARTESIAN_POINT('',(-2.9428780301451,17.4394399250575,0.));
#7232=CARTESIAN_POINT('',(-4.08501508966447,18.2065715530743,0.));
#7233=CARTESIAN_POINT('Origin',(-3.10927393821618,18.4254989505611,0.));
#7234=CARTESIAN_POINT('',(-4.08501508966447,18.2065715530743,13.));
#7235=CARTESIAN_POINT('',(-4.08501508966447,18.2065715530743,0.));
#7236=CARTESIAN_POINT('',(-2.9428780301451,17.4394399250575,13.));
#7237=CARTESIAN_POINT('Origin',(-3.10927393821618,18.4254989505611,13.));
#7238=CARTESIAN_POINT('',(-2.9428780301451,17.4394399250575,0.));
#7239=CARTESIAN_POINT('Origin',(-3.86976067797772,17.2472005929999,0.));
#7240=CARTESIAN_POINT('',(-4.1144891981253,18.337935196262,0.));
#7241=CARTESIAN_POINT('',(-3.86976067797772,17.2472005929999,0.));
#7242=CARTESIAN_POINT('',(-4.1144891981253,18.337935196262,13.));
#7243=CARTESIAN_POINT('',(-4.1144891981253,18.337935196262,0.));
#7244=CARTESIAN_POINT('',(-1.93488033898886,8.62360029649997,13.));
#7245=CARTESIAN_POINT('Origin',(-2.73669706567396,18.4845093299966,0.));
#7246=CARTESIAN_POINT('',(-2.59023998199238,17.4952923049513,13.));
#7247=CARTESIAN_POINT('',(-1.74105979901401,18.5778175999297,13.));
#7248=CARTESIAN_POINT('Origin',(-2.73669706567396,18.4845093299966,13.));
#7249=CARTESIAN_POINT('',(-1.74105979901401,18.5778175999297,0.));
#7250=CARTESIAN_POINT('',(-1.74105979901401,18.5778175999297,0.));
#7251=CARTESIAN_POINT('',(-2.59023998199238,17.4952923049513,0.));
#7252=CARTESIAN_POINT('Origin',(-2.73669706567396,18.4845093299966,0.));
#7253=CARTESIAN_POINT('',(-2.59023998199238,17.4952923049513,0.));
#7254=CARTESIAN_POINT('Origin',(-1.75362185428836,18.7118598491961,0.));
#7255=CARTESIAN_POINT('',(-1.75362185428836,18.7118598491961,13.));
#7256=CARTESIAN_POINT('',(-0.87681092714418,9.35592992459806,13.));
#7257=CARTESIAN_POINT('',(-1.75362185428836,18.7118598491961,0.));
#7258=CARTESIAN_POINT('',(-1.75362185428836,18.7118598491961,0.));
#7259=CARTESIAN_POINT('',(-1.64931697933718,17.5988843254813,0.));
#7260=CARTESIAN_POINT('Origin',(2.73669706567396,18.4845093299966,0.));
#7261=CARTESIAN_POINT('',(2.59023998199238,17.4952923049513,0.));
#7262=CARTESIAN_POINT('',(1.74105979901401,18.5778175999297,0.));
#7263=CARTESIAN_POINT('Origin',(2.73669706567396,18.4845093299966,0.));
#7264=CARTESIAN_POINT('',(1.74105979901401,18.5778175999297,13.));
#7265=CARTESIAN_POINT('',(1.74105979901401,18.5778175999297,0.));
#7266=CARTESIAN_POINT('',(2.59023998199238,17.4952923049513,13.));
#7267=CARTESIAN_POINT('Origin',(2.73669706567396,18.4845093299966,13.));
#7268=CARTESIAN_POINT('',(2.59023998199238,17.4952923049513,0.));
#7269=CARTESIAN_POINT('Origin',(1.64931697933718,17.5988843254813,0.));
#7270=CARTESIAN_POINT('',(1.75362185428837,18.7118598491961,0.));
#7271=CARTESIAN_POINT('',(1.64931697933718,17.5988843254813,0.));
#7272=CARTESIAN_POINT('',(1.75362185428837,18.7118598491961,13.));
#7273=CARTESIAN_POINT('',(1.75362185428837,18.7118598491961,0.));
#7274=CARTESIAN_POINT('',(0.82465848966859,8.79944216274063,13.));
#7275=CARTESIAN_POINT('Origin',(3.10927393821618,18.4254989505611,0.));
#7276=CARTESIAN_POINT('',(2.9428780301451,17.4394399250575,13.));
#7277=CARTESIAN_POINT('',(4.08501508966447,18.2065715530743,13.));
#7278=CARTESIAN_POINT('Origin',(3.10927393821618,18.4254989505611,13.));
#7279=CARTESIAN_POINT('',(4.08501508966447,18.2065715530743,0.));
#7280=CARTESIAN_POINT('',(4.08501508966447,18.2065715530743,0.));
#7281=CARTESIAN_POINT('',(2.9428780301451,17.4394399250575,0.));
#7282=CARTESIAN_POINT('Origin',(3.10927393821618,18.4254989505611,0.));
#7283=CARTESIAN_POINT('',(2.9428780301451,17.4394399250575,0.));
#7284=CARTESIAN_POINT('Origin',(4.11448919812531,18.337935196262,0.));
#7285=CARTESIAN_POINT('',(4.11448919812531,18.337935196262,13.));
#7286=CARTESIAN_POINT('',(2.05724459906266,9.16896759813102,13.));
#7287=CARTESIAN_POINT('',(4.11448919812531,18.337935196262,0.));
#7288=CARTESIAN_POINT('',(4.11448919812531,18.337935196262,0.));
#7289=CARTESIAN_POINT('',(3.86976067797773,17.2472005929999,0.));
#7290=CARTESIAN_POINT('Origin',(8.31478109308627,16.7341271470625,0.));
#7291=CARTESIAN_POINT('',(7.86980725742929,15.8385835771673,0.));
#7292=CARTESIAN_POINT('',(7.39670762388808,17.1305374208376,0.));
#7293=CARTESIAN_POINT('Origin',(8.31478109308627,16.7341271470625,0.));
#7294=CARTESIAN_POINT('',(7.39670762388808,17.1305374208376,13.));
#7295=CARTESIAN_POINT('',(7.39670762388808,17.1305374208376,0.));
#7296=CARTESIAN_POINT('',(7.86980725742929,15.8385835771673,13.));
#7297=CARTESIAN_POINT('Origin',(8.31478109308627,16.7341271470625,13.));
#7298=CARTESIAN_POINT('',(7.86980725742929,15.8385835771673,0.));
#7299=CARTESIAN_POINT('Origin',(7.00694799924747,16.2278666415473,0.));
#7300=CARTESIAN_POINT('',(7.45007618140239,17.2541372868972,0.));
#7301=CARTESIAN_POINT('',(7.00694799924747,16.2278666415473,0.));
#7302=CARTESIAN_POINT('',(7.45007618140239,17.2541372868972,13.));
#7303=CARTESIAN_POINT('',(7.45007618140239,17.2541372868972,0.));
#7304=CARTESIAN_POINT('',(3.50347399962373,8.11393332077363,13.));
#7305=CARTESIAN_POINT('Origin',(8.65088754544834,16.5628723558448,0.));
#7306=CARTESIAN_POINT('',(8.18792663645507,15.6764936575763,13.));
#7307=CARTESIAN_POINT('',(9.51122023939286,16.0531394299608,13.));
#7308=CARTESIAN_POINT('Origin',(8.65088754544834,16.5628723558448,13.));
#7309=CARTESIAN_POINT('',(9.51122023939286,16.0531394299608,0.));
#7310=CARTESIAN_POINT('',(9.51122023939286,16.0531394299608,0.));
#7311=CARTESIAN_POINT('',(8.18792663645507,15.6764936575763,0.));
#7312=CARTESIAN_POINT('Origin',(8.65088754544834,16.5628723558448,0.));
#7313=CARTESIAN_POINT('',(8.18792663645507,15.6764936575763,0.));
#7314=CARTESIAN_POINT('Origin',(9.57984538049455,16.1689656784104,0.));
#7315=CARTESIAN_POINT('',(9.57984538049455,16.1689656784104,13.));
#7316=CARTESIAN_POINT('',(4.78992269024728,8.08448283920519,13.));
#7317=CARTESIAN_POINT('',(9.57984538049455,16.1689656784104,0.));
#7318=CARTESIAN_POINT('',(9.57984538049455,16.1689656784104,0.));
#7319=CARTESIAN_POINT('',(9.01003919792412,15.2072406981632,0.));
#7320=CARTESIAN_POINT('Origin',(13.0789564146209,13.3456920054543,0.));
#7321=CARTESIAN_POINT('',(12.3790229663377,12.6314839349494,0.));
#7322=CARTESIAN_POINT('',(12.3283141706436,14.0064008835214,0.));
#7323=CARTESIAN_POINT('Origin',(13.0789564146209,13.3456920054543,0.));
#7324=CARTESIAN_POINT('',(12.3283141706436,14.0064008835214,13.));
#7325=CARTESIAN_POINT('',(12.3283141706436,14.0064008835214,0.));
#7326=CARTESIAN_POINT('',(12.3790229663377,12.6314839349494,13.));
#7327=CARTESIAN_POINT('Origin',(13.0789564146209,13.3456920054543,13.));
#7328=CARTESIAN_POINT('',(12.3790229663377,12.6314839349494,0.));
#7329=CARTESIAN_POINT('Origin',(11.678690128714,13.2683523045433,0.));
#7330=CARTESIAN_POINT('',(12.4172651441477,14.1074595503134,0.));
#7331=CARTESIAN_POINT('',(11.678690128714,13.2683523045433,0.));
#7332=CARTESIAN_POINT('',(12.4172651441477,14.1074595503134,13.));
#7333=CARTESIAN_POINT('',(12.4172651441477,14.1074595503134,0.));
#7334=CARTESIAN_POINT('',(5.839345064357,6.63417615227163,13.));
#7335=CARTESIAN_POINT('Origin',(13.3456920054543,13.0789564146209,0.));
#7336=CARTESIAN_POINT('',(12.6314839349494,12.3790229663377,13.));
#7337=CARTESIAN_POINT('',(14.0064008835214,12.3283141706436,13.));
#7338=CARTESIAN_POINT('Origin',(13.3456920054543,13.0789564146209,13.));
#7339=CARTESIAN_POINT('',(14.0064008835214,12.3283141706436,0.));
#7340=CARTESIAN_POINT('',(14.0064008835214,12.3283141706436,0.));
#7341=CARTESIAN_POINT('',(12.6314839349494,12.3790229663377,0.));
#7342=CARTESIAN_POINT('Origin',(13.3456920054543,13.0789564146209,0.));
#7343=CARTESIAN_POINT('',(12.6314839349494,12.3790229663377,0.));
#7344=CARTESIAN_POINT('Origin',(14.1074595503134,12.4172651441477,0.));
#7345=CARTESIAN_POINT('',(14.1074595503134,12.4172651441477,13.));
#7346=CARTESIAN_POINT('',(7.05372977515671,6.20863257207387,13.));
#7347=CARTESIAN_POINT('',(14.1074595503134,12.4172651441477,0.));
#7348=CARTESIAN_POINT('',(14.1074595503134,12.4172651441477,0.));
#7349=CARTESIAN_POINT('',(13.2683523045433,11.678690128714,0.));
#7350=CARTESIAN_POINT('Origin',(16.5628723558448,8.65088754544834,0.));
#7351=CARTESIAN_POINT('',(15.6764936575763,8.18792663645507,0.));
#7352=CARTESIAN_POINT('',(16.0531394299608,9.51122023939286,0.));
#7353=CARTESIAN_POINT('Origin',(16.5628723558448,8.65088754544834,0.));
#7354=CARTESIAN_POINT('',(16.0531394299608,9.51122023939286,13.));
#7355=CARTESIAN_POINT('',(16.0531394299608,9.51122023939286,0.));
#7356=CARTESIAN_POINT('',(15.6764936575763,8.18792663645507,13.));
#7357=CARTESIAN_POINT('Origin',(16.5628723558448,8.65088754544834,13.));
#7358=CARTESIAN_POINT('',(15.6764936575763,8.18792663645507,0.));
#7359=CARTESIAN_POINT('Origin',(15.2072406981632,9.01003919792412,0.));
#7360=CARTESIAN_POINT('',(16.1689656784104,9.57984538049455,0.));
#7361=CARTESIAN_POINT('',(15.2072406981632,9.01003919792412,0.));
#7362=CARTESIAN_POINT('',(16.1689656784104,9.57984538049455,13.));
#7363=CARTESIAN_POINT('',(16.1689656784104,9.57984538049455,0.));
#7364=CARTESIAN_POINT('',(7.6036203490816,4.50501959896206,13.));
#7365=CARTESIAN_POINT('Origin',(16.7341271470625,8.31478109308627,0.));
#7366=CARTESIAN_POINT('',(15.8385835771673,7.86980725742929,13.));
#7367=CARTESIAN_POINT('',(17.1305374208376,7.39670762388807,13.));
#7368=CARTESIAN_POINT('Origin',(16.7341271470625,8.31478109308627,13.));
#7369=CARTESIAN_POINT('',(17.1305374208376,7.39670762388807,0.));
#7370=CARTESIAN_POINT('',(17.1305374208376,7.39670762388807,0.));
#7371=CARTESIAN_POINT('',(15.8385835771673,7.86980725742929,0.));
#7372=CARTESIAN_POINT('Origin',(16.7341271470625,8.31478109308627,0.));
#7373=CARTESIAN_POINT('',(15.8385835771673,7.86980725742929,0.));
#7374=CARTESIAN_POINT('Origin',(17.2541372868972,7.45007618140238,0.));
#7375=CARTESIAN_POINT('',(17.2541372868972,7.45007618140238,13.));
#7376=CARTESIAN_POINT('',(8.62706864344861,3.72503809070119,13.));
#7377=CARTESIAN_POINT('',(17.2541372868972,7.45007618140238,0.));
#7378=CARTESIAN_POINT('',(17.2541372868972,7.45007618140238,0.));
#7379=CARTESIAN_POINT('',(16.2278666415473,7.00694799924746,0.));
#7380=CARTESIAN_POINT('Origin',(18.4254989505611,3.10927393821618,0.));
#7381=CARTESIAN_POINT('',(17.4394399250575,2.9428780301451,0.));
#7382=CARTESIAN_POINT('',(18.2065715530743,4.08501508966447,0.));
#7383=CARTESIAN_POINT('Origin',(18.4254989505611,3.10927393821618,0.));
#7384=CARTESIAN_POINT('',(18.2065715530743,4.08501508966447,13.));
#7385=CARTESIAN_POINT('',(18.2065715530743,4.08501508966447,0.));
#7386=CARTESIAN_POINT('',(17.4394399250575,2.9428780301451,13.));
#7387=CARTESIAN_POINT('Origin',(18.4254989505611,3.10927393821618,13.));
#7388=CARTESIAN_POINT('',(17.4394399250575,2.9428780301451,0.));
#7389=CARTESIAN_POINT('Origin',(17.2472005929999,3.86976067797773,0.));
#7390=CARTESIAN_POINT('',(18.337935196262,4.1144891981253,0.));
#7391=CARTESIAN_POINT('',(17.2472005929999,3.86976067797773,0.));
#7392=CARTESIAN_POINT('',(18.337935196262,4.1144891981253,13.));
#7393=CARTESIAN_POINT('',(18.337935196262,4.1144891981253,0.));
#7394=CARTESIAN_POINT('',(8.62360029649997,1.93488033898886,13.));
#7395=CARTESIAN_POINT('Ctrl Pts',(21.1275013067528,-6.13422273260091,0.));
#7396=CARTESIAN_POINT('Ctrl Pts',(21.1275013067528,-6.13422273260091,21.));
#7397=CARTESIAN_POINT('Ctrl Pts',(21.1204271980506,-6.12649903511518,0.));
#7398=CARTESIAN_POINT('Ctrl Pts',(21.1204271980506,-6.12649903511518,21.));
#7399=CARTESIAN_POINT('Ctrl Pts',(21.1062663590356,-6.11107360216958,0.));
#7400=CARTESIAN_POINT('Ctrl Pts',(21.1062663590356,-6.11107360216958,21.));
#7401=CARTESIAN_POINT('Ctrl Pts',(21.0849872356853,-6.08800133883115,0.));
#7402=CARTESIAN_POINT('Ctrl Pts',(21.0849872356853,-6.08800133883115,21.));
#7403=CARTESIAN_POINT('Ctrl Pts',(21.0565393163693,-6.05737013696533,0.));
#7404=CARTESIAN_POINT('Ctrl Pts',(21.0565393163693,-6.05737013696533,21.));
#7405=CARTESIAN_POINT('Ctrl Pts',(21.0208530236003,-6.01930117633045,0.));
#7406=CARTESIAN_POINT('Ctrl Pts',(21.0208530236003,-6.01930117633045,21.));
#7407=CARTESIAN_POINT('Ctrl Pts',(20.9850401822713,-5.98145286361837,0.));
#7408=CARTESIAN_POINT('Ctrl Pts',(20.9850401822713,-5.98145286361837,21.));
#7409=CARTESIAN_POINT('Ctrl Pts',(20.9491006734021,-5.94382608200804,0.));
#7410=CARTESIAN_POINT('Ctrl Pts',(20.9491006734021,-5.94382608200804,21.));
#7411=CARTESIAN_POINT('Ctrl Pts',(20.9130344665641,-5.906422006626,0.));
#7412=CARTESIAN_POINT('Ctrl Pts',(20.9130344665641,-5.906422006626,21.));
#7413=CARTESIAN_POINT('Ctrl Pts',(20.8768416821402,-5.86924212736288,0.));
#7414=CARTESIAN_POINT('Ctrl Pts',(20.8768416821402,-5.86924212736288,21.));
#7415=CARTESIAN_POINT('Ctrl Pts',(20.8405225541277,-5.83228817460178,0.));
#7416=CARTESIAN_POINT('Ctrl Pts',(20.8405225541277,-5.83228817460178,21.));
#7417=CARTESIAN_POINT('Ctrl Pts',(20.8040773827343,-5.79556203439644,0.));
#7418=CARTESIAN_POINT('Ctrl Pts',(20.8040773827343,-5.79556203439644,21.));
#7419=CARTESIAN_POINT('Ctrl Pts',(20.7675064905026,-5.75906566327796,0.));
#7420=CARTESIAN_POINT('Ctrl Pts',(20.7675064905026,-5.75906566327796,21.));
#7421=CARTESIAN_POINT('Ctrl Pts',(20.7308101804425,-5.72280100798241,0.));
#7422=CARTESIAN_POINT('Ctrl Pts',(20.7308101804425,-5.72280100798241,21.));
#7423=CARTESIAN_POINT('Ctrl Pts',(20.6939886877061,-5.68676990500164,0.));
#7424=CARTESIAN_POINT('Ctrl Pts',(20.6939886877061,-5.68676990500164,21.));
#7425=CARTESIAN_POINT('Ctrl Pts',(20.6570421847033,-5.65097411164335,0.));
#7426=CARTESIAN_POINT('Ctrl Pts',(20.6570421847033,-5.65097411164335,21.));
#7427=CARTESIAN_POINT('Ctrl Pts',(20.6199707996366,-5.6154153671515,0.));
#7428=CARTESIAN_POINT('Ctrl Pts',(20.6199707996366,-5.6154153671515,21.));
#7429=CARTESIAN_POINT('Ctrl Pts',(20.5827746317185,-5.58009544402475,0.));
#7430=CARTESIAN_POINT('Ctrl Pts',(20.5827746317185,-5.58009544402475,21.));
#7431=CARTESIAN_POINT('Ctrl Pts',(20.5454537676144,-5.5450161968946,0.));
#7432=CARTESIAN_POINT('Ctrl Pts',(20.5454537676144,-5.5450161968946,21.));
#7433=CARTESIAN_POINT('Ctrl Pts',(20.5080083009242,-5.51017962306782,0.));
#7434=CARTESIAN_POINT('Ctrl Pts',(20.5080083009242,-5.51017962306782,21.));
#7435=CARTESIAN_POINT('Ctrl Pts',(20.4704383353718,-5.47558784449851,0.));
#7436=CARTESIAN_POINT('Ctrl Pts',(20.4704383353718,-5.47558784449851,21.));
#7437=CARTESIAN_POINT('Ctrl Pts',(20.4327439816542,-5.44124306065111,0.));
#7438=CARTESIAN_POINT('Ctrl Pts',(20.4327439816542,-5.44124306065111,21.));
#7439=CARTESIAN_POINT('Ctrl Pts',(20.3949253578015,-5.40714750595875,0.));
#7440=CARTESIAN_POINT('Ctrl Pts',(20.3949253578015,-5.40714750595875,21.));
#7441=CARTESIAN_POINT('Ctrl Pts',(20.3569825877537,-5.37330341114649,0.));
#7442=CARTESIAN_POINT('Ctrl Pts',(20.3569825877537,-5.37330341114649,21.));
#7443=CARTESIAN_POINT('Ctrl Pts',(20.3189158047642,-5.33971294212214,0.));
#7444=CARTESIAN_POINT('Ctrl Pts',(20.3189158047642,-5.33971294212214,21.));
#7445=CARTESIAN_POINT('Ctrl Pts',(20.2807251380077,-5.30637824220998,0.));
#7446=CARTESIAN_POINT('Ctrl Pts',(20.2807251380077,-5.30637824220998,21.));
#7447=CARTESIAN_POINT('Ctrl Pts',(20.2424106921768,-5.27330152298151,0.));
#7448=CARTESIAN_POINT('Ctrl Pts',(20.2424106921768,-5.27330152298151,21.));
#7449=CARTESIAN_POINT('Ctrl Pts',(20.2039725283917,-5.24048514441891,0.));
#7450=CARTESIAN_POINT('Ctrl Pts',(20.2039725283917,-5.24048514441891,21.));
#7451=CARTESIAN_POINT('Ctrl Pts',(20.1654106491899,-5.20793168386164,0.));
#7452=CARTESIAN_POINT('Ctrl Pts',(20.1654106491899,-5.20793168386164,21.));
#7453=CARTESIAN_POINT('Ctrl Pts',(20.1267249732337,-5.17564404279922,0.));
#7454=CARTESIAN_POINT('Ctrl Pts',(20.1267249732337,-5.17564404279922,21.));
#7455=CARTESIAN_POINT('Ctrl Pts',(20.087915358486,-5.14362537555398,0.));
#7456=CARTESIAN_POINT('Ctrl Pts',(20.087915358486,-5.14362537555398,21.));
#7457=CARTESIAN_POINT('Ctrl Pts',(20.0489816528155,-5.11187891582335,0.));
#7458=CARTESIAN_POINT('Ctrl Pts',(20.0489816528155,-5.11187891582335,21.));
#7459=CARTESIAN_POINT('Ctrl Pts',(20.0099237417205,-5.08040781745337,0.));
#7460=CARTESIAN_POINT('Ctrl Pts',(20.0099237417205,-5.08040781745337,21.));
#7461=CARTESIAN_POINT('Ctrl Pts',(19.9707415879783,-5.04921502064063,0.));
#7462=CARTESIAN_POINT('Ctrl Pts',(19.9707415879783,-5.04921502064063,21.));
#7463=CARTESIAN_POINT('Ctrl Pts',(19.931435301086,-5.01830302225558,0.));
#7464=CARTESIAN_POINT('Ctrl Pts',(19.931435301086,-5.01830302225558,21.));
#7465=CARTESIAN_POINT('Ctrl Pts',(19.8920050831202,-4.98767405031333,0.));
#7466=CARTESIAN_POINT('Ctrl Pts',(19.8920050831202,-4.98767405031333,21.));
#7467=CARTESIAN_POINT('Ctrl Pts',(19.8524510953961,-4.95733049830096,0.));
#7468=CARTESIAN_POINT('Ctrl Pts',(19.8524510953961,-4.95733049830096,21.));
#7469=CARTESIAN_POINT('Ctrl Pts',(19.8127733387903,-4.92727531494347,0.));
#7470=CARTESIAN_POINT('Ctrl Pts',(19.8127733387903,-4.92727531494347,21.));
#7471=CARTESIAN_POINT('Ctrl Pts',(19.772971552601,-4.89751233527805,0.));
#7472=CARTESIAN_POINT('Ctrl Pts',(19.772971552601,-4.89751233527805,21.));
#7473=CARTESIAN_POINT('Ctrl Pts',(19.7330450480715,-4.86804682289087,0.));
#7474=CARTESIAN_POINT('Ctrl Pts',(19.7330450480715,-4.86804682289087,21.));
#7475=CARTESIAN_POINT('Ctrl Pts',(19.6929928227072,-4.83888510708974,0.));
#7476=CARTESIAN_POINT('Ctrl Pts',(19.6929928227072,-4.83888510708974,21.));
#7477=CARTESIAN_POINT('Ctrl Pts',(19.6528138625329,-4.81003361418061,0.));
#7478=CARTESIAN_POINT('Ctrl Pts',(19.6528138625329,-4.81003361418061,21.));
#7479=CARTESIAN_POINT('Ctrl Pts',(19.6125074152527,-4.78149799361731,0.));
#7480=CARTESIAN_POINT('Ctrl Pts',(19.6125074152527,-4.78149799361731,21.));
#7481=CARTESIAN_POINT('Ctrl Pts',(19.5720732205813,-4.75328238194611,0.));
#7482=CARTESIAN_POINT('Ctrl Pts',(19.5720732205813,-4.75328238194611,21.));
#7483=CARTESIAN_POINT('Ctrl Pts',(19.531511899192,-4.72538815796616,0.));
#7484=CARTESIAN_POINT('Ctrl Pts',(19.531511899192,-4.72538815796616,21.));
#7485=CARTESIAN_POINT('Ctrl Pts',(19.4908246636763,-4.69781487613785,0.));
#7486=CARTESIAN_POINT('Ctrl Pts',(19.4908246636763,-4.69781487613785,21.));
#7487=CARTESIAN_POINT('Ctrl Pts',(19.4500125912299,-4.67056260851454,0.));
#7488=CARTESIAN_POINT('Ctrl Pts',(19.4500125912299,-4.67056260851454,21.));
#7489=CARTESIAN_POINT('Ctrl Pts',(19.4090759683639,-4.64363405547472,0.));
#7490=CARTESIAN_POINT('Ctrl Pts',(19.4090759683639,-4.64363405547472,21.));
#7491=CARTESIAN_POINT('Ctrl Pts',(19.3680137353983,-4.61703633725712,0.));
#7492=CARTESIAN_POINT('Ctrl Pts',(19.3680137353983,-4.61703633725712,21.));
#7493=CARTESIAN_POINT('Ctrl Pts',(19.3268225655679,-4.59078395765677,0.));
#7494=CARTESIAN_POINT('Ctrl Pts',(19.3268225655679,-4.59078395765677,21.));
#7495=CARTESIAN_POINT('Ctrl Pts',(19.2854975819105,-4.56489651606741,0.));
#7496=CARTESIAN_POINT('Ctrl Pts',(19.2854975819105,-4.56489651606741,21.));
#7497=CARTESIAN_POINT('Ctrl Pts',(19.2440340196551,-4.53939338835152,0.));
#7498=CARTESIAN_POINT('Ctrl Pts',(19.2440340196551,-4.53939338835152,21.));
#7499=CARTESIAN_POINT('Ctrl Pts',(19.2024287376926,-4.51428889122955,0.));
#7500=CARTESIAN_POINT('Ctrl Pts',(19.2024287376926,-4.51428889122955,21.));
#7501=CARTESIAN_POINT('Ctrl Pts',(19.1606814968494,-4.48958819710577,0.));
#7502=CARTESIAN_POINT('Ctrl Pts',(19.1606814968494,-4.48958819710577,21.));
#7503=CARTESIAN_POINT('Ctrl Pts',(19.1187970904932,-4.46528051067022,0.));
#7504=CARTESIAN_POINT('Ctrl Pts',(19.1187970904932,-4.46528051067022,21.));
#7505=CARTESIAN_POINT('Ctrl Pts',(19.0767833717249,-4.44134542994082,0.));
#7506=CARTESIAN_POINT('Ctrl Pts',(19.0767833717249,-4.44134542994082,21.));
#7507=CARTESIAN_POINT('Ctrl Pts',(19.034647328575,-4.41776558033332,0.));
#7508=CARTESIAN_POINT('Ctrl Pts',(19.034647328575,-4.41776558033332,21.));
#7509=CARTESIAN_POINT('Ctrl Pts',(18.9923914823906,-4.39453820875555,0.));
#7510=CARTESIAN_POINT('Ctrl Pts',(18.9923914823906,-4.39453820875555,21.));
#7511=CARTESIAN_POINT('Ctrl Pts',(18.9500107909187,-4.37168516143123,0.));
#7512=CARTESIAN_POINT('Ctrl Pts',(18.9500107909187,-4.37168516143123,21.));
#7513=CARTESIAN_POINT('Ctrl Pts',(18.9074876952706,-4.34926881342022,0.));
#7514=CARTESIAN_POINT('Ctrl Pts',(18.9074876952706,-4.34926881342022,21.));
#7515=CARTESIAN_POINT('Ctrl Pts',(18.8647973781745,-4.32737526247704,0.));
#7516=CARTESIAN_POINT('Ctrl Pts',(18.8647973781745,-4.32737526247704,21.));
#7517=CARTESIAN_POINT('Ctrl Pts',(18.8219166495975,-4.30608591031526,0.));
#7518=CARTESIAN_POINT('Ctrl Pts',(18.8219166495975,-4.30608591031526,21.));
#7519=CARTESIAN_POINT('Ctrl Pts',(18.778832216358,-4.28545098663153,0.));
#7520=CARTESIAN_POINT('Ctrl Pts',(18.778832216358,-4.28545098663153,21.));
#7521=CARTESIAN_POINT('Ctrl Pts',(18.735547949685,-4.26546636161933,0.));
#7522=CARTESIAN_POINT('Ctrl Pts',(18.735547949685,-4.26546636161933,21.));
#7523=CARTESIAN_POINT('Ctrl Pts',(18.6920958920047,-4.24603817988453,0.));
#7524=CARTESIAN_POINT('Ctrl Pts',(18.6920958920047,-4.24603817988453,21.));
#7525=CARTESIAN_POINT('Ctrl Pts',(18.6485210883348,-4.22703266508919,0.));
#7526=CARTESIAN_POINT('Ctrl Pts',(18.6485210883348,-4.22703266508919,21.));
#7527=CARTESIAN_POINT('Ctrl Pts',(18.6048602364653,-4.20834600700665,0.));
#7528=CARTESIAN_POINT('Ctrl Pts',(18.6048602364653,-4.20834600700665,21.));
#7529=CARTESIAN_POINT('Ctrl Pts',(18.5611217636409,-4.18996967278621,0.));
#7530=CARTESIAN_POINT('Ctrl Pts',(18.5611217636409,-4.18996967278621,21.));
#7531=CARTESIAN_POINT('Ctrl Pts',(18.5172668097744,-4.17205262766562,0.));
#7532=CARTESIAN_POINT('Ctrl Pts',(18.5172668097744,-4.17205262766562,21.));
#7533=CARTESIAN_POINT('Ctrl Pts',(18.4731856794913,-4.15497867673974,0.));
#7534=CARTESIAN_POINT('Ctrl Pts',(18.4731856794913,-4.15497867673974,21.));
#7535=CARTESIAN_POINT('Ctrl Pts',(18.4287286547442,-4.13926275457062,0.));
#7536=CARTESIAN_POINT('Ctrl Pts',(18.4287286547442,-4.13926275457062,21.));
#7537=CARTESIAN_POINT('Ctrl Pts',(18.3927403741815,-4.12819301671079,0.));
#7538=CARTESIAN_POINT('Ctrl Pts',(18.3927403741815,-4.12819301671079,21.));
#7539=CARTESIAN_POINT('Ctrl Pts',(18.3654573320481,-4.1209201986886,0.));
#7540=CARTESIAN_POINT('Ctrl Pts',(18.3654573320481,-4.1209201986886,21.));
#7541=CARTESIAN_POINT('Ctrl Pts',(18.3471320125699,-4.11655269114952,0.));
#7542=CARTESIAN_POINT('Ctrl Pts',(18.3471320125699,-4.11655269114952,21.));
#7543=CARTESIAN_POINT('Ctrl Pts',(18.337935196262,-4.11448919812531,0.));
#7544=CARTESIAN_POINT('Ctrl Pts',(18.337935196262,-4.11448919812531,21.));
#7545=CARTESIAN_POINT('',(21.1275013067528,-6.13422273260085,0.));
#7546=CARTESIAN_POINT('Ctrl Pts',(18.337935196262,-4.11448919812531,0.));
#7547=CARTESIAN_POINT('Ctrl Pts',(18.3471320125699,-4.11655269114952,0.));
#7548=CARTESIAN_POINT('Ctrl Pts',(18.3654573320481,-4.1209201986886,0.));
#7549=CARTESIAN_POINT('Ctrl Pts',(18.3927403741815,-4.12819301671079,0.));
#7550=CARTESIAN_POINT('Ctrl Pts',(18.4287286547442,-4.13926275457062,0.));
#7551=CARTESIAN_POINT('Ctrl Pts',(18.4731856794913,-4.15497867673974,0.));
#7552=CARTESIAN_POINT('Ctrl Pts',(18.5172668097744,-4.17205262766562,0.));
#7553=CARTESIAN_POINT('Ctrl Pts',(18.5611217636409,-4.18996967278621,0.));
#7554=CARTESIAN_POINT('Ctrl Pts',(18.6048602364653,-4.20834600700665,0.));
#7555=CARTESIAN_POINT('Ctrl Pts',(18.6485210883348,-4.22703266508919,0.));
#7556=CARTESIAN_POINT('Ctrl Pts',(18.6920958920047,-4.24603817988453,0.));
#7557=CARTESIAN_POINT('Ctrl Pts',(18.735547949685,-4.26546636161933,0.));
#7558=CARTESIAN_POINT('Ctrl Pts',(18.778832216358,-4.28545098663153,0.));
#7559=CARTESIAN_POINT('Ctrl Pts',(18.8219166495975,-4.30608591031526,0.));
#7560=CARTESIAN_POINT('Ctrl Pts',(18.8647973781745,-4.32737526247704,0.));
#7561=CARTESIAN_POINT('Ctrl Pts',(18.9074876952706,-4.34926881342022,0.));
#7562=CARTESIAN_POINT('Ctrl Pts',(18.9500107909187,-4.37168516143123,0.));
#7563=CARTESIAN_POINT('Ctrl Pts',(18.9923914823906,-4.39453820875555,0.));
#7564=CARTESIAN_POINT('Ctrl Pts',(19.034647328575,-4.41776558033332,0.));
#7565=CARTESIAN_POINT('Ctrl Pts',(19.0767833717249,-4.44134542994082,0.));
#7566=CARTESIAN_POINT('Ctrl Pts',(19.1187970904932,-4.46528051067022,0.));
#7567=CARTESIAN_POINT('Ctrl Pts',(19.1606814968494,-4.48958819710577,0.));
#7568=CARTESIAN_POINT('Ctrl Pts',(19.2024287376926,-4.51428889122955,0.));
#7569=CARTESIAN_POINT('Ctrl Pts',(19.2440340196551,-4.53939338835152,0.));
#7570=CARTESIAN_POINT('Ctrl Pts',(19.2854975819105,-4.56489651606741,0.));
#7571=CARTESIAN_POINT('Ctrl Pts',(19.3268225655679,-4.59078395765677,0.));
#7572=CARTESIAN_POINT('Ctrl Pts',(19.3680137353983,-4.61703633725712,0.));
#7573=CARTESIAN_POINT('Ctrl Pts',(19.4090759683639,-4.64363405547472,0.));
#7574=CARTESIAN_POINT('Ctrl Pts',(19.4500125912299,-4.67056260851454,0.));
#7575=CARTESIAN_POINT('Ctrl Pts',(19.4908246636763,-4.69781487613785,0.));
#7576=CARTESIAN_POINT('Ctrl Pts',(19.531511899192,-4.72538815796616,0.));
#7577=CARTESIAN_POINT('Ctrl Pts',(19.5720732205813,-4.75328238194611,0.));
#7578=CARTESIAN_POINT('Ctrl Pts',(19.6125074152527,-4.78149799361731,0.));
#7579=CARTESIAN_POINT('Ctrl Pts',(19.6528138625329,-4.81003361418061,0.));
#7580=CARTESIAN_POINT('Ctrl Pts',(19.6929928227072,-4.83888510708974,0.));
#7581=CARTESIAN_POINT('Ctrl Pts',(19.7330450480715,-4.86804682289087,0.));
#7582=CARTESIAN_POINT('Ctrl Pts',(19.772971552601,-4.89751233527805,0.));
#7583=CARTESIAN_POINT('Ctrl Pts',(19.8127733387903,-4.92727531494347,0.));
#7584=CARTESIAN_POINT('Ctrl Pts',(19.8524510953961,-4.95733049830096,0.));
#7585=CARTESIAN_POINT('Ctrl Pts',(19.8920050831202,-4.98767405031333,0.));
#7586=CARTESIAN_POINT('Ctrl Pts',(19.931435301086,-5.01830302225558,0.));
#7587=CARTESIAN_POINT('Ctrl Pts',(19.9707415879783,-5.04921502064063,0.));
#7588=CARTESIAN_POINT('Ctrl Pts',(20.0099237417205,-5.08040781745337,0.));
#7589=CARTESIAN_POINT('Ctrl Pts',(20.0489816528155,-5.11187891582335,0.));
#7590=CARTESIAN_POINT('Ctrl Pts',(20.087915358486,-5.14362537555398,0.));
#7591=CARTESIAN_POINT('Ctrl Pts',(20.1267249732337,-5.17564404279922,0.));
#7592=CARTESIAN_POINT('Ctrl Pts',(20.1654106491899,-5.20793168386164,0.));
#7593=CARTESIAN_POINT('Ctrl Pts',(20.2039725283917,-5.24048514441891,0.));
#7594=CARTESIAN_POINT('Ctrl Pts',(20.2424106921768,-5.27330152298151,0.));
#7595=CARTESIAN_POINT('Ctrl Pts',(20.2807251380077,-5.30637824220998,0.));
#7596=CARTESIAN_POINT('Ctrl Pts',(20.3189158047642,-5.33971294212214,0.));
#7597=CARTESIAN_POINT('Ctrl Pts',(20.3569825877537,-5.37330341114649,0.));
#7598=CARTESIAN_POINT('Ctrl Pts',(20.3949253578015,-5.40714750595875,0.));
#7599=CARTESIAN_POINT('Ctrl Pts',(20.4327439816542,-5.44124306065111,0.));
#7600=CARTESIAN_POINT('Ctrl Pts',(20.4704383353718,-5.47558784449851,0.));
#7601=CARTESIAN_POINT('Ctrl Pts',(20.5080083009242,-5.51017962306782,0.));
#7602=CARTESIAN_POINT('Ctrl Pts',(20.5454537676144,-5.5450161968946,0.));
#7603=CARTESIAN_POINT('Ctrl Pts',(20.5827746317185,-5.58009544402475,0.));
#7604=CARTESIAN_POINT('Ctrl Pts',(20.6199707996366,-5.6154153671515,0.));
#7605=CARTESIAN_POINT('Ctrl Pts',(20.6570421847033,-5.65097411164335,0.));
#7606=CARTESIAN_POINT('Ctrl Pts',(20.6939886877061,-5.68676990500164,0.));
#7607=CARTESIAN_POINT('Ctrl Pts',(20.7308101804425,-5.72280100798241,0.));
#7608=CARTESIAN_POINT('Ctrl Pts',(20.7675064905026,-5.75906566327796,0.));
#7609=CARTESIAN_POINT('Ctrl Pts',(20.8040773827343,-5.79556203439644,0.));
#7610=CARTESIAN_POINT('Ctrl Pts',(20.8405225541277,-5.83228817460178,0.));
#7611=CARTESIAN_POINT('Ctrl Pts',(20.8768416821402,-5.86924212736288,0.));
#7612=CARTESIAN_POINT('Ctrl Pts',(20.9130344665641,-5.906422006626,0.));
#7613=CARTESIAN_POINT('Ctrl Pts',(20.9491006734021,-5.94382608200804,0.));
#7614=CARTESIAN_POINT('Ctrl Pts',(20.9850401822713,-5.98145286361837,0.));
#7615=CARTESIAN_POINT('Ctrl Pts',(21.0280155918661,-6.02687083887287,0.));
#7616=CARTESIAN_POINT('Ctrl Pts',(21.0636702474951,-6.06499496148845,0.));
#7617=CARTESIAN_POINT('Ctrl Pts',(21.0920928984154,-6.09567013127872,0.));
#7618=CARTESIAN_POINT('Ctrl Pts',(21.1133530893457,-6.11877533761501,0.));
#7619=CARTESIAN_POINT('Ctrl Pts',(21.1275013067528,-6.13422273260091,0.));
#7620=CARTESIAN_POINT('',(21.1275013067528,-6.13422273260085,13.));
#7621=CARTESIAN_POINT('Ctrl Pts',(21.1275013067528,-6.13422273260091,13.));
#7622=CARTESIAN_POINT('Ctrl Pts',(21.0578559224639,-6.05818207473574,13.));
#7623=CARTESIAN_POINT('Ctrl Pts',(20.9874765040291,-5.98341417184727,13.));
#7624=CARTESIAN_POINT('Ctrl Pts',(20.91635991547,-5.90994468705572,13.));
#7625=CARTESIAN_POINT('Ctrl Pts',(20.7985166473367,-5.78820256793373,13.));
#7626=CARTESIAN_POINT('Ctrl Pts',(20.6786545089329,-5.67003811891004,13.));
#7627=CARTESIAN_POINT('Ctrl Pts',(20.5568062999927,-5.55573863837939,13.));
#7628=CARTESIAN_POINT('Ctrl Pts',(20.4631466220902,-5.46788135574845,13.));
#7629=CARTESIAN_POINT('Ctrl Pts',(20.3683108766313,-5.38230707224949,13.));
#7630=CARTESIAN_POINT('Ctrl Pts',(20.272307558011,-5.29917141503086,13.));
#7631=CARTESIAN_POINT('Ctrl Pts',(20.1689623013743,-5.20967788549041,13.));
#7632=CARTESIAN_POINT('Ctrl Pts',(20.0642651120126,-5.12300396000483,13.));
#7633=CARTESIAN_POINT('Ctrl Pts',(19.9582092065757,-5.03941267542058,13.));
#7634=CARTESIAN_POINT('Ctrl Pts',(19.8994937733358,-4.99313426716769,13.));
#7635=CARTESIAN_POINT('Ctrl Pts',(19.8403635603379,-4.9477958395688,13.));
#7636=CARTESIAN_POINT('Ctrl Pts',(19.780817320786,-4.90344584463339,13.));
#7637=CARTESIAN_POINT('Ctrl Pts',(19.72343623378,-4.86070845370395,13.));
#7638=CARTESIAN_POINT('Ctrl Pts',(19.665666793385,-4.81889538674849,13.));
#7639=CARTESIAN_POINT('Ctrl Pts',(19.607498635726,-4.7780829655059,13.));
#7640=CARTESIAN_POINT('Ctrl Pts',(19.5572235050457,-4.74280851477666,13.));
#7641=CARTESIAN_POINT('Ctrl Pts',(19.5066514991033,-4.70827845306304,13.));
#7642=CARTESIAN_POINT('Ctrl Pts',(19.4557905173051,-4.67449772148844,13.));
#7643=CARTESIAN_POINT('Ctrl Pts',(19.4192898920658,-4.65025481897416,13.));
#7644=CARTESIAN_POINT('Ctrl Pts',(19.382641288743,-4.62639514838843,13.));
#7645=CARTESIAN_POINT('Ctrl Pts',(19.3458364383459,-4.60295743063937,13.));
#7646=CARTESIAN_POINT('Ctrl Pts',(19.309630908347,-4.57990136645455,13.));
#7647=CARTESIAN_POINT('Ctrl Pts',(19.273272273525,-4.55725971984417,13.));
#7648=CARTESIAN_POINT('Ctrl Pts',(19.2367485575731,-4.5350835755811,13.));
#7649=CARTESIAN_POINT('Ctrl Pts',(19.2050803503215,-4.51585555580649,13.));
#7650=CARTESIAN_POINT('Ctrl Pts',(19.1732873013029,-4.49697986255775,13.));
#7651=CARTESIAN_POINT('Ctrl Pts',(19.1413765621579,-4.47844262265296,13.));
#7652=CARTESIAN_POINT('Ctrl Pts',(19.1124727544724,-4.46165213670422,13.));
#7653=CARTESIAN_POINT('Ctrl Pts',(19.0834740456903,-4.4451340112905,13.));
#7654=CARTESIAN_POINT('Ctrl Pts',(19.0543895552964,-4.42886646472448,13.));
#7655=CARTESIAN_POINT('Ctrl Pts',(19.0298903167199,-4.41516354268672,13.));
#7656=CARTESIAN_POINT('Ctrl Pts',(19.0053307306813,-4.40163676089501,13.));
#7657=CARTESIAN_POINT('Ctrl Pts',(18.9807063064772,-4.38830551710826,13.));
#7658=CARTESIAN_POINT('Ctrl Pts',(18.9450720847457,-4.36901375649227,13.));
#7659=CARTESIAN_POINT('Ctrl Pts',(18.9093017976319,-4.35013223002823,13.));
#7660=CARTESIAN_POINT('Ctrl Pts',(18.8733353264261,-4.33187128669082,13.));
#7661=CARTESIAN_POINT('Ctrl Pts',(18.8516029896876,-4.32083731653844,13.));
#7662=CARTESIAN_POINT('Ctrl Pts',(18.829798004179,-4.31003325584325,13.));
#7663=CARTESIAN_POINT('Ctrl Pts',(18.807913802916,-4.29948469303248,13.));
#7664=CARTESIAN_POINT('Ctrl Pts',(18.787730412872,-4.28975595059153,13.));
#7665=CARTESIAN_POINT('Ctrl Pts',(18.7674792481688,-4.28024580001115,13.));
#7666=CARTESIAN_POINT('Ctrl Pts',(18.7471689057697,-4.27093067976999,13.));
#7667=CARTESIAN_POINT('Ctrl Pts',(18.7192299720025,-4.25811678809167,13.));
#7668=CARTESIAN_POINT('Ctrl Pts',(18.6911811213678,-4.24566493398932,13.));
#7669=CARTESIAN_POINT('Ctrl Pts',(18.6630711735883,-4.23343245343576,13.));
#7670=CARTESIAN_POINT('Ctrl Pts',(18.6452377209709,-4.22567194943,13.));
#7671=CARTESIAN_POINT('Ctrl Pts',(18.6273802008519,-4.21799814921869,13.));
#7672=CARTESIAN_POINT('Ctrl Pts',(18.6095026819575,-4.21040342108815,13.));
#7673=CARTESIAN_POINT('Ctrl Pts',(18.5934584408824,-4.2035875060976,13.));
#7674=CARTESIAN_POINT('Ctrl Pts',(18.5773983085029,-4.1968345819819,13.));
#7675=CARTESIAN_POINT('Ctrl Pts',(18.5613135378487,-4.19017810368168,13.));
#7676=CARTESIAN_POINT('Ctrl Pts',(18.5444052404372,-4.18318081927935,13.));
#7677=CARTESIAN_POINT('Ctrl Pts',(18.5274697699669,-4.17628995976621,13.));
#7678=CARTESIAN_POINT('Ctrl Pts',(18.5104789585687,-4.16960404102653,13.));
#7679=CARTESIAN_POINT('Ctrl Pts',(18.4822572583451,-4.15849874475977,13.));
#7680=CARTESIAN_POINT('Ctrl Pts',(18.4538805850219,-4.14796697295268,13.));
#7681=CARTESIAN_POINT('Ctrl Pts',(18.4251735640106,-4.13860964460765,13.));
#7682=CARTESIAN_POINT('Ctrl Pts',(18.4093434909821,-4.13344968074392,13.));
#7683=CARTESIAN_POINT('Ctrl Pts',(18.3934125378936,-4.12864814562055,13.));
#7684=CARTESIAN_POINT('Ctrl Pts',(18.3773590065616,-4.1242788981144,13.));
#7685=CARTESIAN_POINT('Ctrl Pts',(18.3643002867737,-4.1207247406093,13.));
#7686=CARTESIAN_POINT('Ctrl Pts',(18.3511604736845,-4.11745655843684,13.));
#7687=CARTESIAN_POINT('Ctrl Pts',(18.337935196262,-4.11448919812531,13.));
#7688=CARTESIAN_POINT('',(21.1275013067528,-6.13422273260085,0.));
#7689=CARTESIAN_POINT('Origin',(5.38923623413286E-12,-1.75106900012182E-12,
0.));
#7690=CARTESIAN_POINT('',(20.698113262342,-7.45574324794401,0.));
#7691=CARTESIAN_POINT('Origin',(5.38923623413286E-12,-1.75106900012182E-12,
0.));
#7692=CARTESIAN_POINT('',(20.698113262342,-7.45574324794401,13.));
#7693=CARTESIAN_POINT('Origin',(5.38923623413286E-12,-1.75106900012182E-12,
13.));
#7694=CARTESIAN_POINT('',(20.698113262342,-7.45574324794401,0.));
#7695=CARTESIAN_POINT('Ctrl Pts',(17.2541372868972,-7.45007618140239,0.));
#7696=CARTESIAN_POINT('Ctrl Pts',(17.2541372868972,-7.45007618140239,21.));
#7697=CARTESIAN_POINT('Ctrl Pts',(17.2627905583523,-7.45381253347183,0.));
#7698=CARTESIAN_POINT('Ctrl Pts',(17.2627905583523,-7.45381253347183,21.));
#7699=CARTESIAN_POINT('Ctrl Pts',(17.2801832097582,-7.46105049818251,0.));
#7700=CARTESIAN_POINT('Ctrl Pts',(17.2801832097582,-7.46105049818251,21.));
#7701=CARTESIAN_POINT('Ctrl Pts',(17.3065305096784,-7.4712032346092,0.));
#7702=CARTESIAN_POINT('Ctrl Pts',(17.3065305096784,-7.4712032346092,21.));
#7703=CARTESIAN_POINT('Ctrl Pts',(17.3421522689127,-7.48340100912745,0.));
#7704=CARTESIAN_POINT('Ctrl Pts',(17.3421522689127,-7.48340100912745,21.));
#7705=CARTESIAN_POINT('Ctrl Pts',(17.3873563447297,-7.49681774451751,0.));
#7706=CARTESIAN_POINT('Ctrl Pts',(17.3873563447297,-7.49681774451751,21.));
#7707=CARTESIAN_POINT('Ctrl Pts',(17.4330545448126,-7.50891486634214,0.));
#7708=CARTESIAN_POINT('Ctrl Pts',(17.4330545448126,-7.50891486634214,21.));
#7709=CARTESIAN_POINT('Ctrl Pts',(17.4790653226646,-7.52019696747329,0.));
#7710=CARTESIAN_POINT('Ctrl Pts',(17.4790653226646,-7.52019696747329,21.));
#7711=CARTESIAN_POINT('Ctrl Pts',(17.5252518287336,-7.53103903007864,0.));
#7712=CARTESIAN_POINT('Ctrl Pts',(17.5252518287336,-7.53103903007864,21.));
#7713=CARTESIAN_POINT('Ctrl Pts',(17.5715579419204,-7.54158441095318,0.));
#7714=CARTESIAN_POINT('Ctrl Pts',(17.5715579419204,-7.54158441095318,21.));
#7715=CARTESIAN_POINT('Ctrl Pts',(17.6179818599248,-7.55182125346564,0.));
#7716=CARTESIAN_POINT('Ctrl Pts',(17.6179818599248,-7.55182125346564,21.));
#7717=CARTESIAN_POINT('Ctrl Pts',(17.6645549117314,-7.56164400295863,0.));
#7718=CARTESIAN_POINT('Ctrl Pts',(17.6645549117314,-7.56164400295863,21.));
#7719=CARTESIAN_POINT('Ctrl Pts',(17.7113192869136,-7.57091795530424,0.));
#7720=CARTESIAN_POINT('Ctrl Pts',(17.7113192869136,-7.57091795530424,21.));
#7721=CARTESIAN_POINT('Ctrl Pts',(17.7583042294209,-7.57954834582804,0.));
#7722=CARTESIAN_POINT('Ctrl Pts',(17.7583042294209,-7.57954834582804,21.));
#7723=CARTESIAN_POINT('Ctrl Pts',(17.8055090348024,-7.58752955799499,0.));
#7724=CARTESIAN_POINT('Ctrl Pts',(17.8055090348024,-7.58752955799499,21.));
#7725=CARTESIAN_POINT('Ctrl Pts',(17.8529149331931,-7.59491004201956,0.));
#7726=CARTESIAN_POINT('Ctrl Pts',(17.8529149331931,-7.59491004201956,21.));
#7727=CARTESIAN_POINT('Ctrl Pts',(17.900492838997,-7.60176928403059,0.));
#7728=CARTESIAN_POINT('Ctrl Pts',(17.900492838997,-7.60176928403059,21.));
#7729=CARTESIAN_POINT('Ctrl Pts',(17.9482122228183,-7.60819152580111,0.));
#7730=CARTESIAN_POINT('Ctrl Pts',(17.9482122228183,-7.60819152580111,21.));
#7731=CARTESIAN_POINT('Ctrl Pts',(17.9960506269561,-7.61423755067038,0.));
#7732=CARTESIAN_POINT('Ctrl Pts',(17.9960506269561,-7.61423755067038,21.));
#7733=CARTESIAN_POINT('Ctrl Pts',(18.0439992897906,-7.61992799636654,0.));
#7734=CARTESIAN_POINT('Ctrl Pts',(18.0439992897906,-7.61992799636654,21.));
#7735=CARTESIAN_POINT('Ctrl Pts',(18.0920577897363,-7.62525915358074,0.));
#7736=CARTESIAN_POINT('Ctrl Pts',(18.0920577897363,-7.62525915358074,21.));
#7737=CARTESIAN_POINT('Ctrl Pts',(18.1402306858819,-7.63021285851762,0.));
#7738=CARTESIAN_POINT('Ctrl Pts',(18.1402306858819,-7.63021285851762,21.));
#7739=CARTESIAN_POINT('Ctrl Pts',(18.1885236169197,-7.63476798969017,0.));
#7740=CARTESIAN_POINT('Ctrl Pts',(18.1885236169197,-7.63476798969017,21.));
#7741=CARTESIAN_POINT('Ctrl Pts',(18.2369390502576,-7.63891299603827,0.));
#7742=CARTESIAN_POINT('Ctrl Pts',(18.2369390502576,-7.63891299603827,21.));
#7743=CARTESIAN_POINT('Ctrl Pts',(18.2854741391282,-7.6426522027076,0.));
#7744=CARTESIAN_POINT('Ctrl Pts',(18.2854741391282,-7.6426522027076,21.));
#7745=CARTESIAN_POINT('Ctrl Pts',(18.3341230095852,-7.64599903846601,0.));
#7746=CARTESIAN_POINT('Ctrl Pts',(18.3341230095852,-7.64599903846601,21.));
#7747=CARTESIAN_POINT('Ctrl Pts',(18.3828781275628,-7.6489719793775,0.));
#7748=CARTESIAN_POINT('Ctrl Pts',(18.3828781275628,-7.6489719793775,21.));
#7749=CARTESIAN_POINT('Ctrl Pts',(18.4317319183719,-7.65158974829127,0.));
#7750=CARTESIAN_POINT('Ctrl Pts',(18.4317319183719,-7.65158974829127,21.));
#7751=CARTESIAN_POINT('Ctrl Pts',(18.4806785483052,-7.65386603444743,0.));
#7752=CARTESIAN_POINT('Ctrl Pts',(18.4806785483052,-7.65386603444743,21.));
#7753=CARTESIAN_POINT('Ctrl Pts',(18.5297146894905,-7.65580722110437,0.));
#7754=CARTESIAN_POINT('Ctrl Pts',(18.5297146894905,-7.65580722110437,21.));
#7755=CARTESIAN_POINT('Ctrl Pts',(18.5788385228928,-7.65741532450727,0.));
#7756=CARTESIAN_POINT('Ctrl Pts',(18.5788385228928,-7.65741532450727,21.));
#7757=CARTESIAN_POINT('Ctrl Pts',(18.6280491346907,-7.65868976978872,0.));
#7758=CARTESIAN_POINT('Ctrl Pts',(18.6280491346907,-7.65868976978872,21.));
#7759=CARTESIAN_POINT('Ctrl Pts',(18.6773458057584,-7.65962948375622,0.));
#7760=CARTESIAN_POINT('Ctrl Pts',(18.6773458057584,-7.65962948375622,21.));
#7761=CARTESIAN_POINT('Ctrl Pts',(18.7267272235231,-7.66023521705905,0.));
#7762=CARTESIAN_POINT('Ctrl Pts',(18.7267272235231,-7.66023521705905,21.));
#7763=CARTESIAN_POINT('Ctrl Pts',(18.7761911671591,-7.66051046922541,0.));
#7764=CARTESIAN_POINT('Ctrl Pts',(18.7761911671591,-7.66051046922541,21.));
#7765=CARTESIAN_POINT('Ctrl Pts',(18.8257349246207,-7.66046025294775,0.));
#7766=CARTESIAN_POINT('Ctrl Pts',(18.8257349246207,-7.66046025294775,21.));
#7767=CARTESIAN_POINT('Ctrl Pts',(18.8753555389435,-7.66009036321663,0.));
#7768=CARTESIAN_POINT('Ctrl Pts',(18.8753555389435,-7.66009036321663,21.));
#7769=CARTESIAN_POINT('Ctrl Pts',(18.9250501008887,-7.65940650980099,0.));
#7770=CARTESIAN_POINT('Ctrl Pts',(18.9250501008887,-7.65940650980099,21.));
#7771=CARTESIAN_POINT('Ctrl Pts',(18.974816073814,-7.65841335587266,0.));
#7772=CARTESIAN_POINT('Ctrl Pts',(18.974816073814,-7.65841335587266,21.));
#7773=CARTESIAN_POINT('Ctrl Pts',(19.0246514144531,-7.65711415727855,0.));
#7774=CARTESIAN_POINT('Ctrl Pts',(19.0246514144531,-7.65711415727855,21.));
#7775=CARTESIAN_POINT('Ctrl Pts',(19.0745543888799,-7.65551129907202,0.));
#7776=CARTESIAN_POINT('Ctrl Pts',(19.0745543888799,-7.65551129907202,21.));
#7777=CARTESIAN_POINT('Ctrl Pts',(19.1245234597312,-7.65360662280609,0.));
#7778=CARTESIAN_POINT('Ctrl Pts',(19.1245234597312,-7.65360662280609,21.));
#7779=CARTESIAN_POINT('Ctrl Pts',(19.1745571539291,-7.65140181220526,0.));
#7780=CARTESIAN_POINT('Ctrl Pts',(19.1745571539291,-7.65140181220526,21.));
#7781=CARTESIAN_POINT('Ctrl Pts',(19.224653915265,-7.64889882291924,0.));
#7782=CARTESIAN_POINT('Ctrl Pts',(19.224653915265,-7.64889882291924,21.));
#7783=CARTESIAN_POINT('Ctrl Pts',(19.2748120456486,-7.64610005549614,0.));
#7784=CARTESIAN_POINT('Ctrl Pts',(19.2748120456486,-7.64610005549614,21.));
#7785=CARTESIAN_POINT('Ctrl Pts',(19.3250297839295,-7.64300812875339,0.));
#7786=CARTESIAN_POINT('Ctrl Pts',(19.3250297839295,-7.64300812875339,21.));
#7787=CARTESIAN_POINT('Ctrl Pts',(19.3753053524647,-7.63962574822761,0.));
#7788=CARTESIAN_POINT('Ctrl Pts',(19.3753053524647,-7.63962574822761,21.));
#7789=CARTESIAN_POINT('Ctrl Pts',(19.4256370121006,-7.63595554930654,0.));
#7790=CARTESIAN_POINT('Ctrl Pts',(19.4256370121006,-7.63595554930654,21.));
#7791=CARTESIAN_POINT('Ctrl Pts',(19.4760231231881,-7.63199992715366,0.));
#7792=CARTESIAN_POINT('Ctrl Pts',(19.4760231231881,-7.63199992715366,21.));
#7793=CARTESIAN_POINT('Ctrl Pts',(19.5264621687521,-7.62776096538883,0.));
#7794=CARTESIAN_POINT('Ctrl Pts',(19.5264621687521,-7.62776096538883,21.));
#7795=CARTESIAN_POINT('Ctrl Pts',(19.5769527121826,-7.6232405373522,0.));
#7796=CARTESIAN_POINT('Ctrl Pts',(19.5769527121826,-7.6232405373522,21.));
#7797=CARTESIAN_POINT('Ctrl Pts',(19.6274933688524,-7.61844037070591,0.));
#7798=CARTESIAN_POINT('Ctrl Pts',(19.6274933688524,-7.61844037070591,21.));
#7799=CARTESIAN_POINT('Ctrl Pts',(19.6780827744426,-7.61336212350879,0.));
#7800=CARTESIAN_POINT('Ctrl Pts',(19.6780827744426,-7.61336212350879,21.));
#7801=CARTESIAN_POINT('Ctrl Pts',(19.7287195480601,-7.60800746969262,0.));
#7802=CARTESIAN_POINT('Ctrl Pts',(19.7287195480601,-7.60800746969262,21.));
#7803=CARTESIAN_POINT('Ctrl Pts',(19.7794022782484,-7.60237814110187,0.));
#7804=CARTESIAN_POINT('Ctrl Pts',(19.7794022782484,-7.60237814110187,21.));
#7805=CARTESIAN_POINT('Ctrl Pts',(19.830129556152,-7.59647587605448,0.));
#7806=CARTESIAN_POINT('Ctrl Pts',(19.830129556152,-7.59647587605448,21.));
#7807=CARTESIAN_POINT('Ctrl Pts',(19.8808999994024,-7.59030238888852,0.));
#7808=CARTESIAN_POINT('Ctrl Pts',(19.8808999994024,-7.59030238888852,21.));
#7809=CARTESIAN_POINT('Ctrl Pts',(19.931712276832,-7.58385933533352,0.));
#7810=CARTESIAN_POINT('Ctrl Pts',(19.931712276832,-7.58385933533352,21.));
#7811=CARTESIAN_POINT('Ctrl Pts',(19.9825651387294,-7.57714827622806,0.));
#7812=CARTESIAN_POINT('Ctrl Pts',(19.9825651387294,-7.57714827622806,21.));
#7813=CARTESIAN_POINT('Ctrl Pts',(20.0334574248556,-7.57017066105973,0.));
#7814=CARTESIAN_POINT('Ctrl Pts',(20.0334574248556,-7.57017066105973,21.));
#7815=CARTESIAN_POINT('Ctrl Pts',(20.0843880130978,-7.56292786549461,0.));
#7816=CARTESIAN_POINT('Ctrl Pts',(20.0843880130978,-7.56292786549461,21.));
#7817=CARTESIAN_POINT('Ctrl Pts',(20.1353557774357,-7.55542122125495,0.));
#7818=CARTESIAN_POINT('Ctrl Pts',(20.1353557774357,-7.55542122125495,21.));
#7819=CARTESIAN_POINT('Ctrl Pts',(20.1863595454674,-7.54765204869255,0.));
#7820=CARTESIAN_POINT('Ctrl Pts',(20.1863595454674,-7.54765204869255,21.));
#7821=CARTESIAN_POINT('Ctrl Pts',(20.2373980474879,-7.53962169534167,0.));
#7822=CARTESIAN_POINT('Ctrl Pts',(20.2373980474879,-7.53962169534167,21.));
#7823=CARTESIAN_POINT('Ctrl Pts',(20.2884698940944,-7.53133155804008,0.));
#7824=CARTESIAN_POINT('Ctrl Pts',(20.2884698940944,-7.53133155804008,21.));
#7825=CARTESIAN_POINT('Ctrl Pts',(20.3395736743243,-7.52278303006887,0.));
#7826=CARTESIAN_POINT('Ctrl Pts',(20.3395736743243,-7.52278303006887,21.));
#7827=CARTESIAN_POINT('Ctrl Pts',(20.3907080367098,-7.51397746081994,0.));
#7828=CARTESIAN_POINT('Ctrl Pts',(20.3907080367098,-7.51397746081994,21.));
#7829=CARTESIAN_POINT('Ctrl Pts',(20.4418717748497,-7.50491611266253,0.));
#7830=CARTESIAN_POINT('Ctrl Pts',(20.4418717748497,-7.50491611266253,21.));
#7831=CARTESIAN_POINT('Ctrl Pts',(20.493063915616,-7.49560012018406,0.));
#7832=CARTESIAN_POINT('Ctrl Pts',(20.493063915616,-7.49560012018406,21.));
#7833=CARTESIAN_POINT('Ctrl Pts',(20.5442837929044,-7.48603045196745,0.));
#7834=CARTESIAN_POINT('Ctrl Pts',(20.5442837929044,-7.48603045196745,21.));
#7835=CARTESIAN_POINT('Ctrl Pts',(20.5955309838521,-7.47620789245428,0.));
#7836=CARTESIAN_POINT('Ctrl Pts',(20.5955309838521,-7.47620789245428,21.));
#7837=CARTESIAN_POINT('Ctrl Pts',(20.6365504027501,-7.46814799701906,0.));
#7838=CARTESIAN_POINT('Ctrl Pts',(20.6365504027501,-7.46814799701906,21.));
#7839=CARTESIAN_POINT('Ctrl Pts',(20.6673271112931,-7.46198969876654,0.));
#7840=CARTESIAN_POINT('Ctrl Pts',(20.6673271112931,-7.46198969876654,21.));
#7841=CARTESIAN_POINT('Ctrl Pts',(20.6878503127065,-7.45783379370108,0.));
#7842=CARTESIAN_POINT('Ctrl Pts',(20.6878503127065,-7.45783379370108,21.));
#7843=CARTESIAN_POINT('Ctrl Pts',(20.698113262342,-7.45574324794401,0.));
#7844=CARTESIAN_POINT('Ctrl Pts',(20.698113262342,-7.45574324794401,21.));
#7845=CARTESIAN_POINT('Ctrl Pts',(17.2541372868972,-7.45007618140239,0.));
#7846=CARTESIAN_POINT('Ctrl Pts',(17.2627905583523,-7.45381253347183,0.));
#7847=CARTESIAN_POINT('Ctrl Pts',(17.2801832097582,-7.46105049818251,0.));
#7848=CARTESIAN_POINT('Ctrl Pts',(17.3065305096784,-7.4712032346092,0.));
#7849=CARTESIAN_POINT('Ctrl Pts',(17.3421522689127,-7.48340100912745,0.));
#7850=CARTESIAN_POINT('Ctrl Pts',(17.3873563447297,-7.49681774451751,0.));
#7851=CARTESIAN_POINT('Ctrl Pts',(17.4330545448126,-7.50891486634214,0.));
#7852=CARTESIAN_POINT('Ctrl Pts',(17.4790653226646,-7.52019696747329,0.));
#7853=CARTESIAN_POINT('Ctrl Pts',(17.5252518287336,-7.53103903007864,0.));
#7854=CARTESIAN_POINT('Ctrl Pts',(17.5715579419204,-7.54158441095318,0.));
#7855=CARTESIAN_POINT('Ctrl Pts',(17.6179818599248,-7.55182125346564,0.));
#7856=CARTESIAN_POINT('Ctrl Pts',(17.6645549117314,-7.56164400295863,0.));
#7857=CARTESIAN_POINT('Ctrl Pts',(17.7113192869136,-7.57091795530424,0.));
#7858=CARTESIAN_POINT('Ctrl Pts',(17.7583042294209,-7.57954834582804,0.));
#7859=CARTESIAN_POINT('Ctrl Pts',(17.8055090348024,-7.58752955799499,0.));
#7860=CARTESIAN_POINT('Ctrl Pts',(17.8529149331931,-7.59491004201956,0.));
#7861=CARTESIAN_POINT('Ctrl Pts',(17.900492838997,-7.60176928403059,0.));
#7862=CARTESIAN_POINT('Ctrl Pts',(17.9482122228183,-7.60819152580111,0.));
#7863=CARTESIAN_POINT('Ctrl Pts',(17.9960506269561,-7.61423755067038,0.));
#7864=CARTESIAN_POINT('Ctrl Pts',(18.0439992897906,-7.61992799636654,0.));
#7865=CARTESIAN_POINT('Ctrl Pts',(18.0920577897363,-7.62525915358074,0.));
#7866=CARTESIAN_POINT('Ctrl Pts',(18.1402306858819,-7.63021285851762,0.));
#7867=CARTESIAN_POINT('Ctrl Pts',(18.1885236169197,-7.63476798969017,0.));
#7868=CARTESIAN_POINT('Ctrl Pts',(18.2369390502576,-7.63891299603827,0.));
#7869=CARTESIAN_POINT('Ctrl Pts',(18.2854741391282,-7.6426522027076,0.));
#7870=CARTESIAN_POINT('Ctrl Pts',(18.3341230095852,-7.64599903846601,0.));
#7871=CARTESIAN_POINT('Ctrl Pts',(18.3828781275628,-7.6489719793775,0.));
#7872=CARTESIAN_POINT('Ctrl Pts',(18.4317319183719,-7.65158974829127,0.));
#7873=CARTESIAN_POINT('Ctrl Pts',(18.4806785483052,-7.65386603444743,0.));
#7874=CARTESIAN_POINT('Ctrl Pts',(18.5297146894905,-7.65580722110437,0.));
#7875=CARTESIAN_POINT('Ctrl Pts',(18.5788385228928,-7.65741532450727,0.));
#7876=CARTESIAN_POINT('Ctrl Pts',(18.6280491346907,-7.65868976978872,0.));
#7877=CARTESIAN_POINT('Ctrl Pts',(18.6773458057584,-7.65962948375622,0.));
#7878=CARTESIAN_POINT('Ctrl Pts',(18.7267272235231,-7.66023521705905,0.));
#7879=CARTESIAN_POINT('Ctrl Pts',(18.7761911671591,-7.66051046922541,0.));
#7880=CARTESIAN_POINT('Ctrl Pts',(18.8257349246207,-7.66046025294775,0.));
#7881=CARTESIAN_POINT('Ctrl Pts',(18.8753555389435,-7.66009036321663,0.));
#7882=CARTESIAN_POINT('Ctrl Pts',(18.9250501008887,-7.65940650980099,0.));
#7883=CARTESIAN_POINT('Ctrl Pts',(18.974816073814,-7.65841335587266,0.));
#7884=CARTESIAN_POINT('Ctrl Pts',(19.0246514144531,-7.65711415727855,0.));
#7885=CARTESIAN_POINT('Ctrl Pts',(19.0745543888799,-7.65551129907202,0.));
#7886=CARTESIAN_POINT('Ctrl Pts',(19.1245234597312,-7.65360662280609,0.));
#7887=CARTESIAN_POINT('Ctrl Pts',(19.1745571539291,-7.65140181220526,0.));
#7888=CARTESIAN_POINT('Ctrl Pts',(19.224653915265,-7.64889882291924,0.));
#7889=CARTESIAN_POINT('Ctrl Pts',(19.2748120456486,-7.64610005549614,0.));
#7890=CARTESIAN_POINT('Ctrl Pts',(19.3250297839295,-7.64300812875339,0.));
#7891=CARTESIAN_POINT('Ctrl Pts',(19.3753053524647,-7.63962574822761,0.));
#7892=CARTESIAN_POINT('Ctrl Pts',(19.4256370121006,-7.63595554930654,0.));
#7893=CARTESIAN_POINT('Ctrl Pts',(19.4760231231881,-7.63199992715366,0.));
#7894=CARTESIAN_POINT('Ctrl Pts',(19.5264621687521,-7.62776096538883,0.));
#7895=CARTESIAN_POINT('Ctrl Pts',(19.5769527121826,-7.6232405373522,0.));
#7896=CARTESIAN_POINT('Ctrl Pts',(19.6274933688524,-7.61844037070591,0.));
#7897=CARTESIAN_POINT('Ctrl Pts',(19.6780827744426,-7.61336212350879,0.));
#7898=CARTESIAN_POINT('Ctrl Pts',(19.7287195480601,-7.60800746969262,0.));
#7899=CARTESIAN_POINT('Ctrl Pts',(19.7794022782484,-7.60237814110187,0.));
#7900=CARTESIAN_POINT('Ctrl Pts',(19.830129556152,-7.59647587605448,0.));
#7901=CARTESIAN_POINT('Ctrl Pts',(19.8808999994024,-7.59030238888852,0.));
#7902=CARTESIAN_POINT('Ctrl Pts',(19.931712276832,-7.58385933533352,0.));
#7903=CARTESIAN_POINT('Ctrl Pts',(19.9825651387294,-7.57714827622806,0.));
#7904=CARTESIAN_POINT('Ctrl Pts',(20.0334574248556,-7.57017066105973,0.));
#7905=CARTESIAN_POINT('Ctrl Pts',(20.0843880130978,-7.56292786549461,0.));
#7906=CARTESIAN_POINT('Ctrl Pts',(20.1353557774357,-7.55542122125495,0.));
#7907=CARTESIAN_POINT('Ctrl Pts',(20.1863595454674,-7.54765204869255,0.));
#7908=CARTESIAN_POINT('Ctrl Pts',(20.2373980474879,-7.53962169534167,0.));
#7909=CARTESIAN_POINT('Ctrl Pts',(20.2884698940944,-7.53133155804008,0.));
#7910=CARTESIAN_POINT('Ctrl Pts',(20.3395736743243,-7.52278303006887,0.));
#7911=CARTESIAN_POINT('Ctrl Pts',(20.3907080367098,-7.51397746081994,0.));
#7912=CARTESIAN_POINT('Ctrl Pts',(20.4418717748497,-7.50491611266253,0.));
#7913=CARTESIAN_POINT('Ctrl Pts',(20.493063915616,-7.49560012018406,0.));
#7914=CARTESIAN_POINT('Ctrl Pts',(20.5545277683621,-7.48411651832413,0.));
#7915=CARTESIAN_POINT('Ctrl Pts',(20.6057817877246,-7.47423073598682,0.));
#7916=CARTESIAN_POINT('Ctrl Pts',(20.6468066077586,-7.46612041736314,0.));
#7917=CARTESIAN_POINT('Ctrl Pts',(20.6775873630604,-7.45992433946824,0.));
#7918=CARTESIAN_POINT('Ctrl Pts',(20.698113262342,-7.45574324794401,0.));
#7919=CARTESIAN_POINT('Ctrl Pts',(17.2541372868972,-7.45007618140239,13.));
#7920=CARTESIAN_POINT('Ctrl Pts',(17.2687220121489,-7.45637364573816,13.));
#7921=CARTESIAN_POINT('Ctrl Pts',(17.2834550499008,-7.46226667103919,13.));
#7922=CARTESIAN_POINT('Ctrl Pts',(17.2983267669067,-7.46778231425445,13.));
#7923=CARTESIAN_POINT('Ctrl Pts',(17.3157575315993,-7.47424706065699,13.));
#7924=CARTESIAN_POINT('Ctrl Pts',(17.3333785326113,-7.48019417753821,13.));
#7925=CARTESIAN_POINT('Ctrl Pts',(17.3511502187375,-7.48573450280811,13.));
#7926=CARTESIAN_POINT('Ctrl Pts',(17.3761558316968,-7.49353000563121,13.));
#7927=CARTESIAN_POINT('Ctrl Pts',(17.4014574303076,-7.50052692940225,13.));
#7928=CARTESIAN_POINT('Ctrl Pts',(17.4269165094415,-7.50711117101491,13.));
#7929=CARTESIAN_POINT('Ctrl Pts',(17.4438508122163,-7.51149073008789,13.));
#7930=CARTESIAN_POINT('Ctrl Pts',(17.4608540901313,-7.51568961154288,13.));
#7931=CARTESIAN_POINT('Ctrl Pts',(17.477895354957,-7.51979276933228,13.));
#7932=CARTESIAN_POINT('Ctrl Pts',(17.4958340796489,-7.52411201550939,13.));
#7933=CARTESIAN_POINT('Ctrl Pts',(17.5138146001159,-7.52832602172309,13.));
#7934=CARTESIAN_POINT('Ctrl Pts',(17.5318219263269,-7.53247314101538,13.));
#7935=CARTESIAN_POINT('Ctrl Pts',(17.5518200478141,-7.53707874400482,13.));
#7936=CARTESIAN_POINT('Ctrl Pts',(17.5718516505912,-7.54160061545737,13.));
#7937=CARTESIAN_POINT('Ctrl Pts',(17.5919190740356,-7.5460260137895,13.));
#7938=CARTESIAN_POINT('Ctrl Pts',(17.6221716888696,-7.55269751656612,13.));
#7939=CARTESIAN_POINT('Ctrl Pts',(17.6525076946371,-7.55914375118857,13.));
#7940=CARTESIAN_POINT('Ctrl Pts',(17.6829731243219,-7.56521559976811,13.));
#7941=CARTESIAN_POINT('Ctrl Pts',(17.7051055929398,-7.56962666501585,13.));
#7942=CARTESIAN_POINT('Ctrl Pts',(17.727307481075,-7.57383703867015,13.));
#7943=CARTESIAN_POINT('Ctrl Pts',(17.7495842479971,-7.57782678310872,13.));
#7944=CARTESIAN_POINT('Ctrl Pts',(17.7768156880447,-7.58270390405109,13.));
#7945=CARTESIAN_POINT('Ctrl Pts',(17.8041586050554,-7.58725254420668,13.));
#7946=CARTESIAN_POINT('Ctrl Pts',(17.8315958504975,-7.59151733245669,13.));
#7947=CARTESIAN_POINT('Ctrl Pts',(17.8612326292199,-7.59612401157578,13.));
#7948=CARTESIAN_POINT('Ctrl Pts',(17.890977551337,-7.60040516926074,13.));
#7949=CARTESIAN_POINT('Ctrl Pts',(17.9207992272247,-7.60444696777948,13.));
#7950=CARTESIAN_POINT('Ctrl Pts',(17.9483304583238,-7.60817833718655,13.));
#7951=CARTESIAN_POINT('Ctrl Pts',(17.9759263070057,-7.61170808544497,13.));
#7952=CARTESIAN_POINT('Ctrl Pts',(18.0035762489904,-7.61506270604885,13.));
#7953=CARTESIAN_POINT('Ctrl Pts',(18.0411401148466,-7.61962013038026,13.));
#7954=CARTESIAN_POINT('Ctrl Pts',(18.078804438117,-7.62385245909278,13.));
#7955=CARTESIAN_POINT('Ctrl Pts',(18.1165756810882,-7.62773031180414,13.));
#7956=CARTESIAN_POINT('Ctrl Pts',(18.1530241147805,-7.63147235591759,13.));
#7957=CARTESIAN_POINT('Ctrl Pts',(18.1895746220981,-7.63487692331431,13.));
#7958=CARTESIAN_POINT('Ctrl Pts',(18.226229844125,-7.63792794642091,13.));
#7959=CARTESIAN_POINT('Ctrl Pts',(18.2760269902476,-7.6420728467942,13.));
#7960=CARTESIAN_POINT('Ctrl Pts',(18.3260163399595,-7.64556831472346,13.));
#7961=CARTESIAN_POINT('Ctrl Pts',(18.3761647741053,-7.64849356609124,13.));
#7962=CARTESIAN_POINT('Ctrl Pts',(18.4202441575742,-7.65106479845333,13.));
#7963=CARTESIAN_POINT('Ctrl Pts',(18.4644442731323,-7.65320196597273,13.));
#7964=CARTESIAN_POINT('Ctrl Pts',(18.5087513218567,-7.65493429570881,13.));
#7965=CARTESIAN_POINT('Ctrl Pts',(18.5740706685388,-7.65748817031469,13.));
#7966=CARTESIAN_POINT('Ctrl Pts',(18.6396252901705,-7.65915358769517,13.));
#7967=CARTESIAN_POINT('Ctrl Pts',(18.7054034394317,-7.65993127489945,13.));
#7968=CARTESIAN_POINT('Ctrl Pts',(18.7884161056895,-7.66091272374024,13.));
#7969=CARTESIAN_POINT('Ctrl Pts',(18.8717830756661,-7.66048522719283,13.));
#7970=CARTESIAN_POINT('Ctrl Pts',(18.9554457129062,-7.65875983806947,13.));
#7971=CARTESIAN_POINT('Ctrl Pts',(19.0687732052289,-7.65642266547867,13.));
#7972=CARTESIAN_POINT('Ctrl Pts',(19.1826450748833,-7.65169843824266,13.));
#7973=CARTESIAN_POINT('Ctrl Pts',(19.2969757396511,-7.64469887386167,13.));
#7974=CARTESIAN_POINT('Ctrl Pts',(19.3989045212746,-7.63845857891806,13.));
#7975=CARTESIAN_POINT('Ctrl Pts',(19.5011952230427,-7.63041784747171,13.));
#7976=CARTESIAN_POINT('Ctrl Pts',(19.6037897795036,-7.62065725315813,13.));
#7977=CARTESIAN_POINT('Ctrl Pts',(19.7491944785472,-7.6068238069441,13.));
#7978=CARTESIAN_POINT('Ctrl Pts',(19.8952104286167,-7.5895301524174,13.));
#7979=CARTESIAN_POINT('Ctrl Pts',(20.0416957573265,-7.56895177464837,13.));
#7980=CARTESIAN_POINT('Ctrl Pts',(20.15548208037,-7.55296697971251,13.));
#7981=CARTESIAN_POINT('Ctrl Pts',(20.2695554921735,-7.53499708076544,13.));
#7982=CARTESIAN_POINT('Ctrl Pts',(20.3838501740658,-7.51511029118453,13.));
#7983=CARTESIAN_POINT('Ctrl Pts',(20.482723707906,-7.4979067159171,13.));
#7984=CARTESIAN_POINT('Ctrl Pts',(20.5817593863818,-7.47927116738907,13.));
#7985=CARTESIAN_POINT('Ctrl Pts',(20.6809436221336,-7.45922688157452,13.));
#7986=CARTESIAN_POINT('Ctrl Pts',(20.6866663320398,-7.45807037084351,13.));
#7987=CARTESIAN_POINT('Ctrl Pts',(20.6923895454539,-7.45690915954643,13.));
#7988=CARTESIAN_POINT('Ctrl Pts',(20.698113262342,-7.45574324794401,13.));
#7989=CARTESIAN_POINT('Ctrl Pts',(18.1978687191668,-12.3627494547115,0.));
#7990=CARTESIAN_POINT('Ctrl Pts',(18.1978687191668,-12.3627494547115,21.));
#7991=CARTESIAN_POINT('Ctrl Pts',(18.1935275957711,-12.3532177620787,0.));
#7992=CARTESIAN_POINT('Ctrl Pts',(18.1935275957711,-12.3532177620787,21.));
#7993=CARTESIAN_POINT('Ctrl Pts',(18.1848265584754,-12.3341713636489,0.));
#7994=CARTESIAN_POINT('Ctrl Pts',(18.1848265584754,-12.3341713636489,21.));
#7995=CARTESIAN_POINT('Ctrl Pts',(18.1717186310224,-12.3056527265146,0.));
#7996=CARTESIAN_POINT('Ctrl Pts',(18.1717186310224,-12.3056527265146,21.));
#7997=CARTESIAN_POINT('Ctrl Pts',(18.1541286139166,-12.2677298318549,0.));
#7998=CARTESIAN_POINT('Ctrl Pts',(18.1541286139166,-12.2677298318549,21.));
#7999=CARTESIAN_POINT('Ctrl Pts',(18.1319528884305,-12.2204964278426,0.));
#8000=CARTESIAN_POINT('Ctrl Pts',(18.1319528884305,-12.2204964278426,21.));
#8001=CARTESIAN_POINT('Ctrl Pts',(18.109588624154,-12.1734337668195,0.));
#8002=CARTESIAN_POINT('Ctrl Pts',(18.109588624154,-12.1734337668195,21.));
#8003=CARTESIAN_POINT('Ctrl Pts',(18.0870354350127,-12.1265426519718,0.));
#8004=CARTESIAN_POINT('Ctrl Pts',(18.0870354350127,-12.1265426519718,21.));
#8005=CARTESIAN_POINT('Ctrl Pts',(18.0642929289333,-12.0798241915081,0.));
#8006=CARTESIAN_POINT('Ctrl Pts',(18.0642929289333,-12.0798241915081,21.));
#8007=CARTESIAN_POINT('Ctrl Pts',(18.0413607600052,-12.0332798395991,0.));
#8008=CARTESIAN_POINT('Ctrl Pts',(18.0413607600052,-12.0332798395991,21.));
#8009=CARTESIAN_POINT('Ctrl Pts',(18.0182386160553,-11.986911314246,0.));
#8010=CARTESIAN_POINT('Ctrl Pts',(18.0182386160553,-11.986911314246,21.));
#8011=CARTESIAN_POINT('Ctrl Pts',(17.9949261997754,-11.9407205019619,0.));
#8012=CARTESIAN_POINT('Ctrl Pts',(17.9949261997754,-11.9407205019619,21.));
#8013=CARTESIAN_POINT('Ctrl Pts',(17.9714232133203,-11.8947093631895,0.));
#8014=CARTESIAN_POINT('Ctrl Pts',(17.9714232133203,-11.8947093631895,21.));
#8015=CARTESIAN_POINT('Ctrl Pts',(17.9477293432951,-11.8488798430201,0.));
#8016=CARTESIAN_POINT('Ctrl Pts',(17.9477293432951,-11.8488798430201,21.));
#8017=CARTESIAN_POINT('Ctrl Pts',(17.9238442458356,-11.8032337607271,0.));
#8018=CARTESIAN_POINT('Ctrl Pts',(17.9238442458356,-11.8032337607271,21.));
#8019=CARTESIAN_POINT('Ctrl Pts',(17.8997675418752,-11.7577728408871,0.));
#8020=CARTESIAN_POINT('Ctrl Pts',(17.8997675418752,-11.7577728408871,21.));
#8021=CARTESIAN_POINT('Ctrl Pts',(17.8754988158862,-11.7124987772363,0.));
#8022=CARTESIAN_POINT('Ctrl Pts',(17.8754988158862,-11.7124987772363,21.));
#8023=CARTESIAN_POINT('Ctrl Pts',(17.8510376144926,-11.6674132861792,0.));
#8024=CARTESIAN_POINT('Ctrl Pts',(17.8510376144926,-11.6674132861792,21.));
#8025=CARTESIAN_POINT('Ctrl Pts',(17.8263834470057,-11.6225181583564,0.));
#8026=CARTESIAN_POINT('Ctrl Pts',(17.8263834470057,-11.6225181583564,21.));
#8027=CARTESIAN_POINT('Ctrl Pts',(17.8015357852426,-11.5778153222435,0.));
#8028=CARTESIAN_POINT('Ctrl Pts',(17.8015357852426,-11.5778153222435,21.));
#8029=CARTESIAN_POINT('Ctrl Pts',(17.7764940721306,-11.5333068279912,0.));
#8030=CARTESIAN_POINT('Ctrl Pts',(17.7764940721306,-11.5333068279912,21.));
#8031=CARTESIAN_POINT('Ctrl Pts',(17.7512577332768,-11.4889948016216,0.));
#8032=CARTESIAN_POINT('Ctrl Pts',(17.7512577332768,-11.4889948016216,21.));
#8033=CARTESIAN_POINT('Ctrl Pts',(17.725826190457,-11.4448814046804,0.));
#8034=CARTESIAN_POINT('Ctrl Pts',(17.725826190457,-11.4448814046804,21.));
#8035=CARTESIAN_POINT('Ctrl Pts',(17.700198872213,-11.4009687970126,0.));
#8036=CARTESIAN_POINT('Ctrl Pts',(17.700198872213,-11.4009687970126,21.));
#8037=CARTESIAN_POINT('Ctrl Pts',(17.674375235974,-11.3572590796967,0.));
#8038=CARTESIAN_POINT('Ctrl Pts',(17.674375235974,-11.3572590796967,21.));
#8039=CARTESIAN_POINT('Ctrl Pts',(17.6483547422688,-11.3137543310722,0.));
#8040=CARTESIAN_POINT('Ctrl Pts',(17.6483547422688,-11.3137543310722,21.));
#8041=CARTESIAN_POINT('Ctrl Pts',(17.6221368072528,-11.2704566868205,0.));
#8042=CARTESIAN_POINT('Ctrl Pts',(17.6221368072528,-11.2704566868205,21.));
#8043=CARTESIAN_POINT('Ctrl Pts',(17.5957207597803,-11.2273684103052,0.));
#8044=CARTESIAN_POINT('Ctrl Pts',(17.5957207597803,-11.2273684103052,21.));
#8045=CARTESIAN_POINT('Ctrl Pts',(17.5691058058227,-11.1844919535058,0.));
#8046=CARTESIAN_POINT('Ctrl Pts',(17.5691058058227,-11.1844919535058,21.));
#8047=CARTESIAN_POINT('Ctrl Pts',(17.5422909714139,-11.1418300507683,0.));
#8048=CARTESIAN_POINT('Ctrl Pts',(17.5422909714139,-11.1418300507683,21.));
#8049=CARTESIAN_POINT('Ctrl Pts',(17.5152751467292,-11.0993856581394,0.));
#8050=CARTESIAN_POINT('Ctrl Pts',(17.5152751467292,-11.0993856581394,21.));
#8051=CARTESIAN_POINT('Ctrl Pts',(17.4880571878157,-11.0571618040371,0.));
#8052=CARTESIAN_POINT('Ctrl Pts',(17.4880571878157,-11.0571618040371,21.));
#8053=CARTESIAN_POINT('Ctrl Pts',(17.460636011184,-11.0151614525643,0.));
#8054=CARTESIAN_POINT('Ctrl Pts',(17.460636011184,-11.0151614525643,21.));
#8055=CARTESIAN_POINT('Ctrl Pts',(17.4330106728622,-10.9733873885115,0.));
#8056=CARTESIAN_POINT('Ctrl Pts',(17.4330106728622,-10.9733873885115,21.));
#8057=CARTESIAN_POINT('Ctrl Pts',(17.4051805054129,-10.9318420203801,0.));
#8058=CARTESIAN_POINT('Ctrl Pts',(17.4051805054129,-10.9318420203801,21.));
#8059=CARTESIAN_POINT('Ctrl Pts',(17.377145012528,-10.8905275295837,0.));
#8060=CARTESIAN_POINT('Ctrl Pts',(17.377145012528,-10.8905275295837,21.));
#8061=CARTESIAN_POINT('Ctrl Pts',(17.3489036079991,-10.8494462423128,0.));
#8062=CARTESIAN_POINT('Ctrl Pts',(17.3489036079991,-10.8494462423128,21.));
#8063=CARTESIAN_POINT('Ctrl Pts',(17.3204553814537,-10.8086009632423,0.));
#8064=CARTESIAN_POINT('Ctrl Pts',(17.3204553814537,-10.8086009632423,21.));
#8065=CARTESIAN_POINT('Ctrl Pts',(17.2917988998581,-10.7679952591482,0.));
#8066=CARTESIAN_POINT('Ctrl Pts',(17.2917988998581,-10.7679952591482,21.));
#8067=CARTESIAN_POINT('Ctrl Pts',(17.2629318816279,-10.7276339231608,0.));
#8068=CARTESIAN_POINT('Ctrl Pts',(17.2629318816279,-10.7276339231608,21.));
#8069=CARTESIAN_POINT('Ctrl Pts',(17.2338514174708,-10.6875226650217,0.));
#8070=CARTESIAN_POINT('Ctrl Pts',(17.2338514174708,-10.6875226650217,21.));
#8071=CARTESIAN_POINT('Ctrl Pts',(17.2045545572011,-10.6476672831754,0.));
#8072=CARTESIAN_POINT('Ctrl Pts',(17.2045545572011,-10.6476672831754,21.));
#8073=CARTESIAN_POINT('Ctrl Pts',(17.1750388395657,-10.6080729180997,0.));
#8074=CARTESIAN_POINT('Ctrl Pts',(17.1750388395657,-10.6080729180997,21.));
#8075=CARTESIAN_POINT('Ctrl Pts',(17.1453027387554,-10.5687434234512,0.));
#8076=CARTESIAN_POINT('Ctrl Pts',(17.1453027387554,-10.5687434234512,21.));
#8077=CARTESIAN_POINT('Ctrl Pts',(17.1153464189932,-10.5296803023445,0.));
#8078=CARTESIAN_POINT('Ctrl Pts',(17.1153464189932,-10.5296803023445,21.));
#8079=CARTESIAN_POINT('Ctrl Pts',(17.0851711712016,-10.4908835057575,0.));
#8080=CARTESIAN_POINT('Ctrl Pts',(17.0851711712016,-10.4908835057575,21.));
#8081=CARTESIAN_POINT('Ctrl Pts',(17.0547779975888,-10.452353435089,0.));
#8082=CARTESIAN_POINT('Ctrl Pts',(17.0547779975888,-10.452353435089,21.));
#8083=CARTESIAN_POINT('Ctrl Pts',(17.0241663361802,-10.4140927470882,0.));
#8084=CARTESIAN_POINT('Ctrl Pts',(17.0241663361802,-10.4140927470882,21.));
#8085=CARTESIAN_POINT('Ctrl Pts',(16.9933329788855,-10.3761078860454,0.));
#8086=CARTESIAN_POINT('Ctrl Pts',(16.9933329788855,-10.3761078860454,21.));
#8087=CARTESIAN_POINT('Ctrl Pts',(16.9622702798438,-10.3384116178624,0.));
#8088=CARTESIAN_POINT('Ctrl Pts',(16.9622702798438,-10.3384116178624,21.));
#8089=CARTESIAN_POINT('Ctrl Pts',(16.9309675442425,-10.3010210756062,0.));
#8090=CARTESIAN_POINT('Ctrl Pts',(16.9309675442425,-10.3010210756062,21.));
#8091=CARTESIAN_POINT('Ctrl Pts',(16.8994142530447,-10.2639532144219,0.));
#8092=CARTESIAN_POINT('Ctrl Pts',(16.8994142530447,-10.2639532144219,21.));
#8093=CARTESIAN_POINT('Ctrl Pts',(16.8676029947679,-10.2272206796636,0.));
#8094=CARTESIAN_POINT('Ctrl Pts',(16.8676029947679,-10.2272206796636,21.));
#8095=CARTESIAN_POINT('Ctrl Pts',(16.8355319435837,-10.1908283166713,0.));
#8096=CARTESIAN_POINT('Ctrl Pts',(16.8355319435837,-10.1908283166713,21.));
#8097=CARTESIAN_POINT('Ctrl Pts',(16.8032089941901,-10.1547673397274,0.));
#8098=CARTESIAN_POINT('Ctrl Pts',(16.8032089941901,-10.1547673397274,21.));
#8099=CARTESIAN_POINT('Ctrl Pts',(16.7706479198888,-10.1190207721353,0.));
#8100=CARTESIAN_POINT('Ctrl Pts',(16.7706479198888,-10.1190207721353,21.));
#8101=CARTESIAN_POINT('Ctrl Pts',(16.7378607357337,-10.0835742491038,0.));
#8102=CARTESIAN_POINT('Ctrl Pts',(16.7378607357337,-10.0835742491038,21.));
#8103=CARTESIAN_POINT('Ctrl Pts',(16.7048506904207,-10.0484259314257,0.));
#8104=CARTESIAN_POINT('Ctrl Pts',(16.7048506904207,-10.0484259314257,21.));
#8105=CARTESIAN_POINT('Ctrl Pts',(16.6716062376276,-10.0135950379525,0.));
#8106=CARTESIAN_POINT('Ctrl Pts',(16.6716062376276,-10.0135950379525,21.));
#8107=CARTESIAN_POINT('Ctrl Pts',(16.6380914029057,-9.97913546489642,0.));
#8108=CARTESIAN_POINT('Ctrl Pts',(16.6380914029057,-9.97913546489642,21.));
#8109=CARTESIAN_POINT('Ctrl Pts',(16.6042559779574,-9.94512142712911,0.));
#8110=CARTESIAN_POINT('Ctrl Pts',(16.6042559779574,-9.94512142712911,21.));
#8111=CARTESIAN_POINT('Ctrl Pts',(16.570052753238,-9.91162317616649,0.));
#8112=CARTESIAN_POINT('Ctrl Pts',(16.570052753238,-9.91162317616649,21.));
#8113=CARTESIAN_POINT('Ctrl Pts',(16.5354535643506,-9.8786843754698,0.));
#8114=CARTESIAN_POINT('Ctrl Pts',(16.5354535643506,-9.8786843754698,21.));
#8115=CARTESIAN_POINT('Ctrl Pts',(16.5004633692332,-9.84630229363522,0.));
#8116=CARTESIAN_POINT('Ctrl Pts',(16.5004633692332,-9.84630229363522,21.));
#8117=CARTESIAN_POINT('Ctrl Pts',(16.4651416449558,-9.81439757053279,0.));
#8118=CARTESIAN_POINT('Ctrl Pts',(16.4651416449558,-9.81439757053279,21.));
#8119=CARTESIAN_POINT('Ctrl Pts',(16.4295725710378,-9.78285689698058,0.));
#8120=CARTESIAN_POINT('Ctrl Pts',(16.4295725710378,-9.78285689698058,21.));
#8121=CARTESIAN_POINT('Ctrl Pts',(16.3938231282759,-9.75159288382685,0.));
#8122=CARTESIAN_POINT('Ctrl Pts',(16.3938231282759,-9.75159288382685,21.));
#8123=CARTESIAN_POINT('Ctrl Pts',(16.3579039682519,-9.72060002001012,0.));
#8124=CARTESIAN_POINT('Ctrl Pts',(16.3579039682519,-9.72060002001012,21.));
#8125=CARTESIAN_POINT('Ctrl Pts',(16.3217321000366,-9.69000797146316,0.));
#8126=CARTESIAN_POINT('Ctrl Pts',(16.3217321000366,-9.69000797146316,21.));
#8127=CARTESIAN_POINT('Ctrl Pts',(16.2850845948324,-9.66014786078746,0.));
#8128=CARTESIAN_POINT('Ctrl Pts',(16.2850845948324,-9.66014786078746,21.));
#8129=CARTESIAN_POINT('Ctrl Pts',(16.2476599387841,-9.63146315443274,0.));
#8130=CARTESIAN_POINT('Ctrl Pts',(16.2476599387841,-9.63146315443274,21.));
#8131=CARTESIAN_POINT('Ctrl Pts',(16.2168537871666,-9.60981421781524,0.));
#8132=CARTESIAN_POINT('Ctrl Pts',(16.2168537871666,-9.60981421781524,21.));
#8133=CARTESIAN_POINT('Ctrl Pts',(16.1931534965272,-9.59446643316597,0.));
#8134=CARTESIAN_POINT('Ctrl Pts',(16.1931534965272,-9.59446643316597,21.));
#8135=CARTESIAN_POINT('Ctrl Pts',(16.1770747160769,-9.58464985151483,0.));
#8136=CARTESIAN_POINT('Ctrl Pts',(16.1770747160769,-9.58464985151483,21.));
#8137=CARTESIAN_POINT('Ctrl Pts',(16.1689656784104,-9.57984538049455,0.));
#8138=CARTESIAN_POINT('Ctrl Pts',(16.1689656784104,-9.57984538049455,21.));
#8139=CARTESIAN_POINT('',(18.1978687191669,-12.3627494547114,0.));
#8140=CARTESIAN_POINT('Ctrl Pts',(16.1689656784104,-9.57984538049455,0.));
#8141=CARTESIAN_POINT('Ctrl Pts',(16.1770747160769,-9.58464985151483,0.));
#8142=CARTESIAN_POINT('Ctrl Pts',(16.1931534965272,-9.59446643316597,0.));
#8143=CARTESIAN_POINT('Ctrl Pts',(16.2168537871666,-9.60981421781524,0.));
#8144=CARTESIAN_POINT('Ctrl Pts',(16.2476599387841,-9.63146315443274,0.));
#8145=CARTESIAN_POINT('Ctrl Pts',(16.2850845948324,-9.66014786078746,0.));
#8146=CARTESIAN_POINT('Ctrl Pts',(16.3217321000366,-9.69000797146316,0.));
#8147=CARTESIAN_POINT('Ctrl Pts',(16.3579039682519,-9.72060002001012,0.));
#8148=CARTESIAN_POINT('Ctrl Pts',(16.3938231282759,-9.75159288382685,0.));
#8149=CARTESIAN_POINT('Ctrl Pts',(16.4295725710378,-9.78285689698058,0.));
#8150=CARTESIAN_POINT('Ctrl Pts',(16.4651416449558,-9.81439757053279,0.));
#8151=CARTESIAN_POINT('Ctrl Pts',(16.5004633692332,-9.84630229363522,0.));
#8152=CARTESIAN_POINT('Ctrl Pts',(16.5354535643506,-9.8786843754698,0.));
#8153=CARTESIAN_POINT('Ctrl Pts',(16.570052753238,-9.91162317616649,0.));
#8154=CARTESIAN_POINT('Ctrl Pts',(16.6042559779574,-9.94512142712911,0.));
#8155=CARTESIAN_POINT('Ctrl Pts',(16.6380914029057,-9.97913546489642,0.));
#8156=CARTESIAN_POINT('Ctrl Pts',(16.6716062376276,-10.0135950379525,0.));
#8157=CARTESIAN_POINT('Ctrl Pts',(16.7048506904207,-10.0484259314257,0.));
#8158=CARTESIAN_POINT('Ctrl Pts',(16.7378607357337,-10.0835742491038,0.));
#8159=CARTESIAN_POINT('Ctrl Pts',(16.7706479198888,-10.1190207721353,0.));
#8160=CARTESIAN_POINT('Ctrl Pts',(16.8032089941901,-10.1547673397274,0.));
#8161=CARTESIAN_POINT('Ctrl Pts',(16.8355319435837,-10.1908283166713,0.));
#8162=CARTESIAN_POINT('Ctrl Pts',(16.8676029947679,-10.2272206796636,0.));
#8163=CARTESIAN_POINT('Ctrl Pts',(16.8994142530447,-10.2639532144219,0.));
#8164=CARTESIAN_POINT('Ctrl Pts',(16.9309675442425,-10.3010210756062,0.));
#8165=CARTESIAN_POINT('Ctrl Pts',(16.9622702798438,-10.3384116178624,0.));
#8166=CARTESIAN_POINT('Ctrl Pts',(16.9933329788855,-10.3761078860454,0.));
#8167=CARTESIAN_POINT('Ctrl Pts',(17.0241663361802,-10.4140927470882,0.));
#8168=CARTESIAN_POINT('Ctrl Pts',(17.0547779975888,-10.452353435089,0.));
#8169=CARTESIAN_POINT('Ctrl Pts',(17.0851711712016,-10.4908835057575,0.));
#8170=CARTESIAN_POINT('Ctrl Pts',(17.1153464189932,-10.5296803023445,0.));
#8171=CARTESIAN_POINT('Ctrl Pts',(17.1453027387554,-10.5687434234512,0.));
#8172=CARTESIAN_POINT('Ctrl Pts',(17.1750388395657,-10.6080729180997,0.));
#8173=CARTESIAN_POINT('Ctrl Pts',(17.2045545572011,-10.6476672831754,0.));
#8174=CARTESIAN_POINT('Ctrl Pts',(17.2338514174708,-10.6875226650217,0.));
#8175=CARTESIAN_POINT('Ctrl Pts',(17.2629318816279,-10.7276339231608,0.));
#8176=CARTESIAN_POINT('Ctrl Pts',(17.2917988998581,-10.7679952591482,0.));
#8177=CARTESIAN_POINT('Ctrl Pts',(17.3204553814537,-10.8086009632423,0.));
#8178=CARTESIAN_POINT('Ctrl Pts',(17.3489036079991,-10.8494462423128,0.));
#8179=CARTESIAN_POINT('Ctrl Pts',(17.377145012528,-10.8905275295837,0.));
#8180=CARTESIAN_POINT('Ctrl Pts',(17.4051805054129,-10.9318420203801,0.));
#8181=CARTESIAN_POINT('Ctrl Pts',(17.4330106728622,-10.9733873885115,0.));
#8182=CARTESIAN_POINT('Ctrl Pts',(17.460636011184,-11.0151614525643,0.));
#8183=CARTESIAN_POINT('Ctrl Pts',(17.4880571878157,-11.0571618040371,0.));
#8184=CARTESIAN_POINT('Ctrl Pts',(17.5152751467292,-11.0993856581394,0.));
#8185=CARTESIAN_POINT('Ctrl Pts',(17.5422909714139,-11.1418300507683,0.));
#8186=CARTESIAN_POINT('Ctrl Pts',(17.5691058058227,-11.1844919535058,0.));
#8187=CARTESIAN_POINT('Ctrl Pts',(17.5957207597803,-11.2273684103052,0.));
#8188=CARTESIAN_POINT('Ctrl Pts',(17.6221368072528,-11.2704566868205,0.));
#8189=CARTESIAN_POINT('Ctrl Pts',(17.6483547422688,-11.3137543310722,0.));
#8190=CARTESIAN_POINT('Ctrl Pts',(17.674375235974,-11.3572590796967,0.));
#8191=CARTESIAN_POINT('Ctrl Pts',(17.700198872213,-11.4009687970126,0.));
#8192=CARTESIAN_POINT('Ctrl Pts',(17.725826190457,-11.4448814046804,0.));
#8193=CARTESIAN_POINT('Ctrl Pts',(17.7512577332768,-11.4889948016216,0.));
#8194=CARTESIAN_POINT('Ctrl Pts',(17.7764940721306,-11.5333068279912,0.));
#8195=CARTESIAN_POINT('Ctrl Pts',(17.8015357852426,-11.5778153222435,0.));
#8196=CARTESIAN_POINT('Ctrl Pts',(17.8263834470057,-11.6225181583564,0.));
#8197=CARTESIAN_POINT('Ctrl Pts',(17.8510376144926,-11.6674132861792,0.));
#8198=CARTESIAN_POINT('Ctrl Pts',(17.8754988158862,-11.7124987772363,0.));
#8199=CARTESIAN_POINT('Ctrl Pts',(17.8997675418752,-11.7577728408871,0.));
#8200=CARTESIAN_POINT('Ctrl Pts',(17.9238442458356,-11.8032337607271,0.));
#8201=CARTESIAN_POINT('Ctrl Pts',(17.9477293432951,-11.8488798430201,0.));
#8202=CARTESIAN_POINT('Ctrl Pts',(17.9714232133203,-11.8947093631895,0.));
#8203=CARTESIAN_POINT('Ctrl Pts',(17.9949261997754,-11.9407205019619,0.));
#8204=CARTESIAN_POINT('Ctrl Pts',(18.0182386160553,-11.986911314246,0.));
#8205=CARTESIAN_POINT('Ctrl Pts',(18.0413607600052,-12.0332798395991,0.));
#8206=CARTESIAN_POINT('Ctrl Pts',(18.0642929289333,-12.0798241915081,0.));
#8207=CARTESIAN_POINT('Ctrl Pts',(18.0870354350127,-12.1265426519718,0.));
#8208=CARTESIAN_POINT('Ctrl Pts',(18.109588624154,-12.1734337668195,0.));
#8209=CARTESIAN_POINT('Ctrl Pts',(18.1364257412858,-12.2299089600472,0.));
#8210=CARTESIAN_POINT('Ctrl Pts',(18.1585543320743,-12.2771850498068,0.));
#8211=CARTESIAN_POINT('Ctrl Pts',(18.1761067306718,-12.3151419520839,0.));
#8212=CARTESIAN_POINT('Ctrl Pts',(18.1891864723772,-12.3436860694314,0.));
#8213=CARTESIAN_POINT('Ctrl Pts',(18.1978687191668,-12.3627494547115,0.));
#8214=CARTESIAN_POINT('',(18.1978687191669,-12.3627494547114,13.));
#8215=CARTESIAN_POINT('Ctrl Pts',(18.1978687191668,-12.3627494547115,13.));
#8216=CARTESIAN_POINT('Ctrl Pts',(18.1551298837072,-12.2689088964153,13.));
#8217=CARTESIAN_POINT('Ctrl Pts',(18.1112996376559,-12.1760519707549,13.));
#8218=CARTESIAN_POINT('Ctrl Pts',(18.0663670681848,-12.0842021157222,13.));
#8219=CARTESIAN_POINT('Ctrl Pts',(17.9919118458474,-11.9320029101433,13.));
#8220=CARTESIAN_POINT('Ctrl Pts',(17.9144310030486,-11.7825824056667,13.));
#8221=CARTESIAN_POINT('Ctrl Pts',(17.8338669541097,-11.6362239749613,13.));
#8222=CARTESIAN_POINT('Ctrl Pts',(17.7719407006024,-11.5237243004517,13.));
#8223=CARTESIAN_POINT('Ctrl Pts',(17.7081904548334,-11.4130324622867,13.));
#8224=CARTESIAN_POINT('Ctrl Pts',(17.6425762040179,-11.3042990955942,13.));
#8225=CARTESIAN_POINT('Ctrl Pts',(17.5719440403086,-11.1872502401787,13.));
#8226=CARTESIAN_POINT('Ctrl Pts',(17.4991548062463,-11.0724652177424,13.));
#8227=CARTESIAN_POINT('Ctrl Pts',(17.4241207676042,-10.9601920950805,13.));
#8228=CARTESIAN_POINT('Ctrl Pts',(17.3825798893999,-10.8980346502925,13.));
#8229=CARTESIAN_POINT('Ctrl Pts',(17.3403540622895,-10.836643006144,13.));
#8230=CARTESIAN_POINT('Ctrl Pts',(17.2974271280105,-10.7760628579409,13.));
#8231=CARTESIAN_POINT('Ctrl Pts',(17.2560610445451,-10.7176854427117,13.));
#8232=CARTESIAN_POINT('Ctrl Pts',(17.2140399830246,-10.6600671042728,13.));
#8233=CARTESIAN_POINT('Ctrl Pts',(17.1713305020871,-10.6032772263326,13.));
#8234=CARTESIAN_POINT('Ctrl Pts',(17.1344164164088,-10.5541933607851,13.));
#8235=CARTESIAN_POINT('Ctrl Pts',(17.09698995673,-10.5057257117512,13.));
#8236=CARTESIAN_POINT('Ctrl Pts',(17.0590571089409,-10.4578814195699,13.));
#8237=CARTESIAN_POINT('Ctrl Pts',(17.0318344202099,-10.4235457356041,13.));
#8238=CARTESIAN_POINT('Ctrl Pts',(17.0043525707778,-10.3895287991213,13.));
#8239=CARTESIAN_POINT('Ctrl Pts',(16.9765917309458,-10.3558648806384,13.));
#8240=CARTESIAN_POINT('Ctrl Pts',(16.9492829424395,-10.3227491378977,13.));
#8241=CARTESIAN_POINT('Ctrl Pts',(16.9217004805397,-10.2899802176756,13.));
#8242=CARTESIAN_POINT('Ctrl Pts',(16.8938171690435,-10.2576030035887,13.));
#8243=CARTESIAN_POINT('Ctrl Pts',(16.8696406997029,-10.2295300566645,13.));
#8244=CARTESIAN_POINT('Ctrl Pts',(16.8452366239146,-10.2017536139349,13.));
#8245=CARTESIAN_POINT('Ctrl Pts',(16.8206160303422,-10.1742626911979,13.));
#8246=CARTESIAN_POINT('Ctrl Pts',(16.7983154207592,-10.149362221872,13.));
#8247=CARTESIAN_POINT('Ctrl Pts',(16.7758403908295,-10.1246914567643,13.));
#8248=CARTESIAN_POINT('Ctrl Pts',(16.7532063446108,-10.1002324983347,13.));
#8249=CARTESIAN_POINT('Ctrl Pts',(16.7341406199811,-10.0796295640807,13.));
#8250=CARTESIAN_POINT('Ctrl Pts',(16.7149630711762,-10.0591755007626,13.));
#8251=CARTESIAN_POINT('Ctrl Pts',(16.6956634330448,-10.0388873690432,13.));
#8252=CARTESIAN_POINT('Ctrl Pts',(16.6677347575979,-10.0095282358636,13.));
#8253=CARTESIAN_POINT('Ctrl Pts',(16.6395499069818,-9.98051721199954,13.));
#8254=CARTESIAN_POINT('Ctrl Pts',(16.6109867035167,-9.95203577348376,13.));
#8255=CARTESIAN_POINT('Ctrl Pts',(16.5937277072624,-9.93482618278573,13.));
#8256=CARTESIAN_POINT('Ctrl Pts',(16.5763285719921,-9.91781279927099,13.));
#8257=CARTESIAN_POINT('Ctrl Pts',(16.5587751448726,-9.90101792967191,13.));
#8258=CARTESIAN_POINT('Ctrl Pts',(16.5425859470632,-9.8855283352884,13.));
#8259=CARTESIAN_POINT('Ctrl Pts',(16.5262647431237,-9.87022569059541,13.));
#8260=CARTESIAN_POINT('Ctrl Pts',(16.5098269901612,-9.85509024386431,13.));
#8261=CARTESIAN_POINT('Ctrl Pts',(16.4872151945017,-9.83426990245398,13.));
#8262=CARTESIAN_POINT('Ctrl Pts',(16.4643869859048,-9.81375991308894,13.));
#8263=CARTESIAN_POINT('Ctrl Pts',(16.4414328803058,-9.79343968032572,13.));
#8264=CARTESIAN_POINT('Ctrl Pts',(16.4268703866426,-9.78054816252851,13.));
#8265=CARTESIAN_POINT('Ctrl Pts',(16.4122582104797,-9.7677316676722,13.));
#8266=CARTESIAN_POINT('Ctrl Pts',(16.3976025797345,-9.75498419487195,13.));
#8267=CARTESIAN_POINT('Ctrl Pts',(16.3844498332853,-9.74354393136336,13.));
#8268=CARTESIAN_POINT('Ctrl Pts',(16.3712625080567,-9.73215866505371,13.));
#8269=CARTESIAN_POINT('Ctrl Pts',(16.35802194704,-9.7208575105204,13.));
#8270=CARTESIAN_POINT('Ctrl Pts',(16.3441034803567,-9.70897774631286,13.));
#8271=CARTESIAN_POINT('Ctrl Pts',(16.3301262834583,-9.69719080125421,13.));
#8272=CARTESIAN_POINT('Ctrl Pts',(16.3160331240261,-9.68558166516946,13.));
#8273=CARTESIAN_POINT('Ctrl Pts',(16.2926244175233,-9.66629891592753,13.));
#8274=CARTESIAN_POINT('Ctrl Pts',(16.2688910940391,-9.6475137315389,13.));
#8275=CARTESIAN_POINT('Ctrl Pts',(16.2444806682505,-9.62974342619985,13.));
#8276=CARTESIAN_POINT('Ctrl Pts',(16.2310198906751,-9.61994424737003,13.));
#8277=CARTESIAN_POINT('Ctrl Pts',(16.2173524098891,-9.61045478087667,13.));
#8278=CARTESIAN_POINT('Ctrl Pts',(16.2034347660458,-9.60133856557799,13.));
#8279=CARTESIAN_POINT('Ctrl Pts',(16.19211348069,-9.59392299467219,13.));
#8280=CARTESIAN_POINT('Ctrl Pts',(16.1806266997874,-9.58675434325645,13.));
#8281=CARTESIAN_POINT('Ctrl Pts',(16.1689656784104,-9.57984538049455,13.));
#8282=CARTESIAN_POINT('',(18.1978687191669,-12.3627494547114,0.));
#8283=CARTESIAN_POINT('Origin',(4.58435815896522E-12,-3.3307311660966E-12,
0.));
#8284=CARTESIAN_POINT('',(17.3811241238545,-13.4869019493419,0.));
#8285=CARTESIAN_POINT('Origin',(4.58435815896522E-12,-3.3307311660966E-12,
0.));
#8286=CARTESIAN_POINT('',(17.3811241238545,-13.4869019493419,13.));
#8287=CARTESIAN_POINT('Origin',(4.58435815896522E-12,-3.3307311660966E-12,
13.));
#8288=CARTESIAN_POINT('',(17.3811241238545,-13.4869019493419,0.));
#8289=CARTESIAN_POINT('Ctrl Pts',(14.1074595503134,-12.4172651441477,0.));
#8290=CARTESIAN_POINT('Ctrl Pts',(14.1074595503134,-12.4172651441477,21.));
#8291=CARTESIAN_POINT('Ctrl Pts',(14.1145347042316,-12.4234926340671,0.));
#8292=CARTESIAN_POINT('Ctrl Pts',(14.1145347042316,-12.4234926340671,21.));
#8293=CARTESIAN_POINT('Ctrl Pts',(14.1288394445866,-12.4357509724316,0.));
#8294=CARTESIAN_POINT('Ctrl Pts',(14.1288394445866,-12.4357509724316,21.));
#8295=CARTESIAN_POINT('Ctrl Pts',(14.1507598477672,-12.4535485619997,0.));
#8296=CARTESIAN_POINT('Ctrl Pts',(14.1507598477672,-12.4535485619997,21.));
#8297=CARTESIAN_POINT('Ctrl Pts',(14.1808688343892,-12.4761570639125,0.));
#8298=CARTESIAN_POINT('Ctrl Pts',(14.1808688343892,-12.4761570639125,21.));
#8299=CARTESIAN_POINT('Ctrl Pts',(14.2197144660135,-12.5028859651751,0.));
#8300=CARTESIAN_POINT('Ctrl Pts',(14.2197144660135,-12.5028859651751,21.));
#8301=CARTESIAN_POINT('Ctrl Pts',(14.2594378207584,-12.5285125321527,0.));
#8302=CARTESIAN_POINT('Ctrl Pts',(14.2594378207584,-12.5285125321527,21.));
#8303=CARTESIAN_POINT('Ctrl Pts',(14.2997103098726,-12.5534605602317,0.));
#8304=CARTESIAN_POINT('Ctrl Pts',(14.2997103098726,-12.5534605602317,21.));
#8305=CARTESIAN_POINT('Ctrl Pts',(14.3402859058353,-12.5780443898087,0.));
#8306=CARTESIAN_POINT('Ctrl Pts',(14.3402859058353,-12.5780443898087,21.));
#8307=CARTESIAN_POINT('Ctrl Pts',(14.3810669346235,-12.6023830189244,0.));
#8308=CARTESIAN_POINT('Ctrl Pts',(14.3810669346235,-12.6023830189244,21.));
#8309=CARTESIAN_POINT('Ctrl Pts',(14.4220553460485,-12.6264646143111,0.));
#8310=CARTESIAN_POINT('Ctrl Pts',(14.4220553460485,-12.6264646143111,21.));
#8311=CARTESIAN_POINT('Ctrl Pts',(14.463313553928,-12.6501984687124,0.));
#8312=CARTESIAN_POINT('Ctrl Pts',(14.463313553928,-12.6501984687124,21.));
#8313=CARTESIAN_POINT('Ctrl Pts',(14.5049233087958,-12.6734695081852,0.));
#8314=CARTESIAN_POINT('Ctrl Pts',(14.5049233087958,-12.6734695081852,21.));
#8315=CARTESIAN_POINT('Ctrl Pts',(14.5469417071951,-12.6961966430455,0.));
#8316=CARTESIAN_POINT('Ctrl Pts',(14.5469417071951,-12.6961966430455,21.));
#8317=CARTESIAN_POINT('Ctrl Pts',(14.5893698147583,-12.7183743139638,0.));
#8318=CARTESIAN_POINT('Ctrl Pts',(14.5893698147583,-12.7183743139638,21.));
#8319=CARTESIAN_POINT('Ctrl Pts',(14.6321748083434,-12.7400427996252,0.));
#8320=CARTESIAN_POINT('Ctrl Pts',(14.6321748083434,-12.7400427996252,21.));
#8321=CARTESIAN_POINT('Ctrl Pts',(14.6753044633399,-12.7612687078867,0.));
#8322=CARTESIAN_POINT('Ctrl Pts',(14.6753044633399,-12.7612687078867,21.));
#8323=CARTESIAN_POINT('Ctrl Pts',(14.7187037124277,-12.7821227233337,0.));
#8324=CARTESIAN_POINT('Ctrl Pts',(14.7187037124277,-12.7821227233337,21.));
#8325=CARTESIAN_POINT('Ctrl Pts',(14.7623324139791,-12.8026557145457,0.));
#8326=CARTESIAN_POINT('Ctrl Pts',(14.7623324139791,-12.8026557145457,21.));
#8327=CARTESIAN_POINT('Ctrl Pts',(14.8061758577898,-12.8228846016791,0.));
#8328=CARTESIAN_POINT('Ctrl Pts',(14.8061758577898,-12.8228846016791,21.));
#8329=CARTESIAN_POINT('Ctrl Pts',(14.8502347891476,-12.8428057266944,0.));
#8330=CARTESIAN_POINT('Ctrl Pts',(14.8502347891476,-12.8428057266944,21.));
#8331=CARTESIAN_POINT('Ctrl Pts',(14.8945191569251,-12.8624032236317,0.));
#8332=CARTESIAN_POINT('Ctrl Pts',(14.8945191569251,-12.8624032236317,21.));
#8333=CARTESIAN_POINT('Ctrl Pts',(14.9390408507356,-12.8816587472148,0.));
#8334=CARTESIAN_POINT('Ctrl Pts',(14.9390408507356,-12.8816587472148,21.));
#8335=CARTESIAN_POINT('Ctrl Pts',(14.9838057866976,-12.9005620742036,0.));
#8336=CARTESIAN_POINT('Ctrl Pts',(14.9838057866976,-12.9005620742036,21.));
#8337=CARTESIAN_POINT('Ctrl Pts',(15.0288099208306,-12.9191164383568,0.));
#8338=CARTESIAN_POINT('Ctrl Pts',(15.0288099208306,-12.9191164383568,21.));
#8339=CARTESIAN_POINT('Ctrl Pts',(15.0740435169624,-12.9373327960422,0.));
#8340=CARTESIAN_POINT('Ctrl Pts',(15.0740435169624,-12.9373327960422,21.));
#8341=CARTESIAN_POINT('Ctrl Pts',(15.1194937003528,-12.9552263908864,0.));
#8342=CARTESIAN_POINT('Ctrl Pts',(15.1194937003528,-12.9552263908864,21.));
#8343=CARTESIAN_POINT('Ctrl Pts',(15.1651474813659,-12.9728126886697,0.));
#8344=CARTESIAN_POINT('Ctrl Pts',(15.1651474813659,-12.9728126886697,21.));
#8345=CARTESIAN_POINT('Ctrl Pts',(15.2109950816083,-12.9901029059182,0.));
#8346=CARTESIAN_POINT('Ctrl Pts',(15.2109950816083,-12.9901029059182,21.));
#8347=CARTESIAN_POINT('Ctrl Pts',(15.2570313635503,-13.0071020851025,0.));
#8348=CARTESIAN_POINT('Ctrl Pts',(15.2570313635503,-13.0071020851025,21.));
#8349=CARTESIAN_POINT('Ctrl Pts',(15.3032539741328,-13.0238115816729,0.));
#8350=CARTESIAN_POINT('Ctrl Pts',(15.3032539741328,-13.0238115816729,21.));
#8351=CARTESIAN_POINT('Ctrl Pts',(15.3496622219036,-13.0402305665115,0.));
#8352=CARTESIAN_POINT('Ctrl Pts',(15.3496622219036,-13.0402305665115,21.));
#8353=CARTESIAN_POINT('Ctrl Pts',(15.3962557545684,-13.0563577967298,0.));
#8354=CARTESIAN_POINT('Ctrl Pts',(15.3962557545684,-13.0563577967298,21.));
#8355=CARTESIAN_POINT('Ctrl Pts',(15.4430330918328,-13.0721935806302,0.));
#8356=CARTESIAN_POINT('Ctrl Pts',(15.4430330918328,-13.0721935806302,21.));
#8357=CARTESIAN_POINT('Ctrl Pts',(15.4899910401523,-13.087740560189,0.));
#8358=CARTESIAN_POINT('Ctrl Pts',(15.4899910401523,-13.087740560189,21.));
#8359=CARTESIAN_POINT('Ctrl Pts',(15.5371254712111,-13.1030026646917,0.));
#8360=CARTESIAN_POINT('Ctrl Pts',(15.5371254712111,-13.1030026646917,21.));
#8361=CARTESIAN_POINT('Ctrl Pts',(15.5844317820184,-13.1179844917497,0.));
#8362=CARTESIAN_POINT('Ctrl Pts',(15.5844317820184,-13.1179844917497,21.));
#8363=CARTESIAN_POINT('Ctrl Pts',(15.6319054413079,-13.1326905726717,0.));
#8364=CARTESIAN_POINT('Ctrl Pts',(15.6319054413079,-13.1326905726717,21.));
#8365=CARTESIAN_POINT('Ctrl Pts',(15.6795425955901,-13.147124558532,0.));
#8366=CARTESIAN_POINT('Ctrl Pts',(15.6795425955901,-13.147124558532,21.));
#8367=CARTESIAN_POINT('Ctrl Pts',(15.7273402954914,-13.161288914421,0.));
#8368=CARTESIAN_POINT('Ctrl Pts',(15.7273402954914,-13.161288914421,21.));
#8369=CARTESIAN_POINT('Ctrl Pts',(15.7752961549278,-13.1751853728467,0.));
#8370=CARTESIAN_POINT('Ctrl Pts',(15.7752961549278,-13.1751853728467,21.));
#8371=CARTESIAN_POINT('Ctrl Pts',(15.8234081427091,-13.1888152101588,0.));
#8372=CARTESIAN_POINT('Ctrl Pts',(15.8234081427091,-13.1888152101588,21.));
#8373=CARTESIAN_POINT('Ctrl Pts',(15.8716743375555,-13.2021795724682,0.));
#8374=CARTESIAN_POINT('Ctrl Pts',(15.8716743375555,-13.2021795724682,21.));
#8375=CARTESIAN_POINT('Ctrl Pts',(15.9200926550954,-13.2152798388134,0.));
#8376=CARTESIAN_POINT('Ctrl Pts',(15.9200926550954,-13.2152798388134,21.));
#8377=CARTESIAN_POINT('Ctrl Pts',(15.9686607385389,-13.2281177675127,0.));
#8378=CARTESIAN_POINT('Ctrl Pts',(15.9686607385389,-13.2281177675127,21.));
#8379=CARTESIAN_POINT('Ctrl Pts',(16.0173761036734,-13.240695304984,0.));
#8380=CARTESIAN_POINT('Ctrl Pts',(16.0173761036734,-13.240695304984,21.));
#8381=CARTESIAN_POINT('Ctrl Pts',(16.0662362238032,-13.2530144750236,0.));
#8382=CARTESIAN_POINT('Ctrl Pts',(16.0662362238032,-13.2530144750236,21.));
#8383=CARTESIAN_POINT('Ctrl Pts',(16.1152386305152,-13.2650772466062,0.));
#8384=CARTESIAN_POINT('Ctrl Pts',(16.1152386305152,-13.2650772466062,21.));
#8385=CARTESIAN_POINT('Ctrl Pts',(16.1643810242643,-13.2768853909882,0.));
#8386=CARTESIAN_POINT('Ctrl Pts',(16.1643810242643,-13.2768853909882,21.));
#8387=CARTESIAN_POINT('Ctrl Pts',(16.2136613184475,-13.2884404210388,0.));
#8388=CARTESIAN_POINT('Ctrl Pts',(16.2136613184475,-13.2884404210388,21.));
#8389=CARTESIAN_POINT('Ctrl Pts',(16.2630775678735,-13.2997436744733,0.));
#8390=CARTESIAN_POINT('Ctrl Pts',(16.2630775678735,-13.2997436744733,21.));
#8391=CARTESIAN_POINT('Ctrl Pts',(16.3126279218067,-13.3107963665229,0.));
#8392=CARTESIAN_POINT('Ctrl Pts',(16.3126279218067,-13.3107963665229,21.));
#8393=CARTESIAN_POINT('Ctrl Pts',(16.3623105703343,-13.3215996524974,0.));
#8394=CARTESIAN_POINT('Ctrl Pts',(16.3623105703343,-13.3215996524974,21.));
#8395=CARTESIAN_POINT('Ctrl Pts',(16.4121236828756,-13.3321546976812,0.));
#8396=CARTESIAN_POINT('Ctrl Pts',(16.4121236828756,-13.3321546976812,21.));
#8397=CARTESIAN_POINT('Ctrl Pts',(16.4620653818862,-13.3424627129921,0.));
#8398=CARTESIAN_POINT('Ctrl Pts',(16.4620653818862,-13.3424627129921,21.));
#8399=CARTESIAN_POINT('Ctrl Pts',(16.5121337902953,-13.3525249163084,0.));
#8400=CARTESIAN_POINT('Ctrl Pts',(16.5121337902953,-13.3525249163084,21.));
#8401=CARTESIAN_POINT('Ctrl Pts',(16.5623270636327,-13.3623425108873,0.));
#8402=CARTESIAN_POINT('Ctrl Pts',(16.5623270636327,-13.3623425108873,21.));
#8403=CARTESIAN_POINT('Ctrl Pts',(16.612643424234,-13.3719166600676,0.));
#8404=CARTESIAN_POINT('Ctrl Pts',(16.612643424234,-13.3719166600676,21.));
#8405=CARTESIAN_POINT('Ctrl Pts',(16.6630812012276,-13.3812484621131,0.));
#8406=CARTESIAN_POINT('Ctrl Pts',(16.6630812012276,-13.3812484621131,21.));
#8407=CARTESIAN_POINT('Ctrl Pts',(16.7136388432444,-13.3903389370346,0.));
#8408=CARTESIAN_POINT('Ctrl Pts',(16.7136388432444,-13.3903389370346,21.));
#8409=CARTESIAN_POINT('Ctrl Pts',(16.7643148579872,-13.3991890464165,0.));
#8410=CARTESIAN_POINT('Ctrl Pts',(16.7643148579872,-13.3991890464165,21.));
#8411=CARTESIAN_POINT('Ctrl Pts',(16.8151077630226,-13.4077997088426,0.));
#8412=CARTESIAN_POINT('Ctrl Pts',(16.8151077630226,-13.4077997088426,21.));
#8413=CARTESIAN_POINT('Ctrl Pts',(16.8660160353187,-13.4161718177499,0.));
#8414=CARTESIAN_POINT('Ctrl Pts',(16.8660160353187,-13.4161718177499,21.));
#8415=CARTESIAN_POINT('Ctrl Pts',(16.9170380509036,-13.4243062623592,0.));
#8416=CARTESIAN_POINT('Ctrl Pts',(16.9170380509036,-13.4243062623592,21.));
#8417=CARTESIAN_POINT('Ctrl Pts',(16.9681720567298,-13.432203941793,0.));
#8418=CARTESIAN_POINT('Ctrl Pts',(16.9681720567298,-13.432203941793,21.));
#8419=CARTESIAN_POINT('Ctrl Pts',(17.0194162803447,-13.4398657451291,0.));
#8420=CARTESIAN_POINT('Ctrl Pts',(17.0194162803447,-13.4398657451291,21.));
#8421=CARTESIAN_POINT('Ctrl Pts',(17.0707690194411,-13.4472925380889,0.));
#8422=CARTESIAN_POINT('Ctrl Pts',(17.0707690194411,-13.4472925380889,21.));
#8423=CARTESIAN_POINT('Ctrl Pts',(17.1222287365697,-13.4544851484583,0.));
#8424=CARTESIAN_POINT('Ctrl Pts',(17.1222287365697,-13.4544851484583,21.));
#8425=CARTESIAN_POINT('Ctrl Pts',(17.1737941556239,-13.4614443545811,0.));
#8426=CARTESIAN_POINT('Ctrl Pts',(17.1737941556239,-13.4614443545811,21.));
#8427=CARTESIAN_POINT('Ctrl Pts',(17.2254643437923,-13.4681708717969,0.));
#8428=CARTESIAN_POINT('Ctrl Pts',(17.2254643437923,-13.4681708717969,21.));
#8429=CARTESIAN_POINT('Ctrl Pts',(17.2772386565028,-13.474665315482,0.));
#8430=CARTESIAN_POINT('Ctrl Pts',(17.2772386565028,-13.474665315482,21.));
#8431=CARTESIAN_POINT('Ctrl Pts',(17.3187410868027,-13.4796755969465,0.));
#8432=CARTESIAN_POINT('Ctrl Pts',(17.3187410868027,-13.4796755969465,21.));
#8433=CARTESIAN_POINT('Ctrl Pts',(17.3499144948292,-13.4833292332349,0.));
#8434=CARTESIAN_POINT('Ctrl Pts',(17.3499144948292,-13.4833292332349,21.));
#8435=CARTESIAN_POINT('Ctrl Pts',(17.3707174645609,-13.485718750657,0.));
#8436=CARTESIAN_POINT('Ctrl Pts',(17.3707174645609,-13.485718750657,21.));
#8437=CARTESIAN_POINT('Ctrl Pts',(17.3811241238545,-13.4869019493419,0.));
#8438=CARTESIAN_POINT('Ctrl Pts',(17.3811241238545,-13.4869019493419,21.));
#8439=CARTESIAN_POINT('Ctrl Pts',(14.1074595503134,-12.4172651441477,0.));
#8440=CARTESIAN_POINT('Ctrl Pts',(14.1145347042316,-12.4234926340671,0.));
#8441=CARTESIAN_POINT('Ctrl Pts',(14.1288394445866,-12.4357509724316,0.));
#8442=CARTESIAN_POINT('Ctrl Pts',(14.1507598477672,-12.4535485619997,0.));
#8443=CARTESIAN_POINT('Ctrl Pts',(14.1808688343892,-12.4761570639125,0.));
#8444=CARTESIAN_POINT('Ctrl Pts',(14.2197144660135,-12.5028859651751,0.));
#8445=CARTESIAN_POINT('Ctrl Pts',(14.2594378207584,-12.5285125321527,0.));
#8446=CARTESIAN_POINT('Ctrl Pts',(14.2997103098726,-12.5534605602317,0.));
#8447=CARTESIAN_POINT('Ctrl Pts',(14.3402859058353,-12.5780443898087,0.));
#8448=CARTESIAN_POINT('Ctrl Pts',(14.3810669346235,-12.6023830189244,0.));
#8449=CARTESIAN_POINT('Ctrl Pts',(14.4220553460485,-12.6264646143111,0.));
#8450=CARTESIAN_POINT('Ctrl Pts',(14.463313553928,-12.6501984687124,0.));
#8451=CARTESIAN_POINT('Ctrl Pts',(14.5049233087958,-12.6734695081852,0.));
#8452=CARTESIAN_POINT('Ctrl Pts',(14.5469417071951,-12.6961966430455,0.));
#8453=CARTESIAN_POINT('Ctrl Pts',(14.5893698147583,-12.7183743139638,0.));
#8454=CARTESIAN_POINT('Ctrl Pts',(14.6321748083434,-12.7400427996252,0.));
#8455=CARTESIAN_POINT('Ctrl Pts',(14.6753044633399,-12.7612687078867,0.));
#8456=CARTESIAN_POINT('Ctrl Pts',(14.7187037124277,-12.7821227233337,0.));
#8457=CARTESIAN_POINT('Ctrl Pts',(14.7623324139791,-12.8026557145457,0.));
#8458=CARTESIAN_POINT('Ctrl Pts',(14.8061758577898,-12.8228846016791,0.));
#8459=CARTESIAN_POINT('Ctrl Pts',(14.8502347891476,-12.8428057266944,0.));
#8460=CARTESIAN_POINT('Ctrl Pts',(14.8945191569251,-12.8624032236317,0.));
#8461=CARTESIAN_POINT('Ctrl Pts',(14.9390408507356,-12.8816587472148,0.));
#8462=CARTESIAN_POINT('Ctrl Pts',(14.9838057866976,-12.9005620742036,0.));
#8463=CARTESIAN_POINT('Ctrl Pts',(15.0288099208306,-12.9191164383568,0.));
#8464=CARTESIAN_POINT('Ctrl Pts',(15.0740435169624,-12.9373327960422,0.));
#8465=CARTESIAN_POINT('Ctrl Pts',(15.1194937003528,-12.9552263908864,0.));
#8466=CARTESIAN_POINT('Ctrl Pts',(15.1651474813659,-12.9728126886697,0.));
#8467=CARTESIAN_POINT('Ctrl Pts',(15.2109950816083,-12.9901029059182,0.));
#8468=CARTESIAN_POINT('Ctrl Pts',(15.2570313635503,-13.0071020851025,0.));
#8469=CARTESIAN_POINT('Ctrl Pts',(15.3032539741328,-13.0238115816729,0.));
#8470=CARTESIAN_POINT('Ctrl Pts',(15.3496622219036,-13.0402305665115,0.));
#8471=CARTESIAN_POINT('Ctrl Pts',(15.3962557545684,-13.0563577967298,0.));
#8472=CARTESIAN_POINT('Ctrl Pts',(15.4430330918328,-13.0721935806302,0.));
#8473=CARTESIAN_POINT('Ctrl Pts',(15.4899910401523,-13.087740560189,0.));
#8474=CARTESIAN_POINT('Ctrl Pts',(15.5371254712111,-13.1030026646917,0.));
#8475=CARTESIAN_POINT('Ctrl Pts',(15.5844317820184,-13.1179844917497,0.));
#8476=CARTESIAN_POINT('Ctrl Pts',(15.6319054413079,-13.1326905726717,0.));
#8477=CARTESIAN_POINT('Ctrl Pts',(15.6795425955901,-13.147124558532,0.));
#8478=CARTESIAN_POINT('Ctrl Pts',(15.7273402954914,-13.161288914421,0.));
#8479=CARTESIAN_POINT('Ctrl Pts',(15.7752961549278,-13.1751853728467,0.));
#8480=CARTESIAN_POINT('Ctrl Pts',(15.8234081427091,-13.1888152101588,0.));
#8481=CARTESIAN_POINT('Ctrl Pts',(15.8716743375555,-13.2021795724682,0.));
#8482=CARTESIAN_POINT('Ctrl Pts',(15.9200926550954,-13.2152798388134,0.));
#8483=CARTESIAN_POINT('Ctrl Pts',(15.9686607385389,-13.2281177675127,0.));
#8484=CARTESIAN_POINT('Ctrl Pts',(16.0173761036734,-13.240695304984,0.));
#8485=CARTESIAN_POINT('Ctrl Pts',(16.0662362238032,-13.2530144750236,0.));
#8486=CARTESIAN_POINT('Ctrl Pts',(16.1152386305152,-13.2650772466062,0.));
#8487=CARTESIAN_POINT('Ctrl Pts',(16.1643810242643,-13.2768853909882,0.));
#8488=CARTESIAN_POINT('Ctrl Pts',(16.2136613184475,-13.2884404210388,0.));
#8489=CARTESIAN_POINT('Ctrl Pts',(16.2630775678735,-13.2997436744733,0.));
#8490=CARTESIAN_POINT('Ctrl Pts',(16.3126279218067,-13.3107963665229,0.));
#8491=CARTESIAN_POINT('Ctrl Pts',(16.3623105703343,-13.3215996524974,0.));
#8492=CARTESIAN_POINT('Ctrl Pts',(16.4121236828756,-13.3321546976812,0.));
#8493=CARTESIAN_POINT('Ctrl Pts',(16.4620653818862,-13.3424627129921,0.));
#8494=CARTESIAN_POINT('Ctrl Pts',(16.5121337902953,-13.3525249163084,0.));
#8495=CARTESIAN_POINT('Ctrl Pts',(16.5623270636327,-13.3623425108873,0.));
#8496=CARTESIAN_POINT('Ctrl Pts',(16.612643424234,-13.3719166600676,0.));
#8497=CARTESIAN_POINT('Ctrl Pts',(16.6630812012276,-13.3812484621131,0.));
#8498=CARTESIAN_POINT('Ctrl Pts',(16.7136388432444,-13.3903389370346,0.));
#8499=CARTESIAN_POINT('Ctrl Pts',(16.7643148579872,-13.3991890464165,0.));
#8500=CARTESIAN_POINT('Ctrl Pts',(16.8151077630226,-13.4077997088426,0.));
#8501=CARTESIAN_POINT('Ctrl Pts',(16.8660160353187,-13.4161718177499,0.));
#8502=CARTESIAN_POINT('Ctrl Pts',(16.9170380509036,-13.4243062623592,0.));
#8503=CARTESIAN_POINT('Ctrl Pts',(16.9681720567298,-13.432203941793,0.));
#8504=CARTESIAN_POINT('Ctrl Pts',(17.0194162803447,-13.4398657451291,0.));
#8505=CARTESIAN_POINT('Ctrl Pts',(17.0707690194411,-13.4472925380889,0.));
#8506=CARTESIAN_POINT('Ctrl Pts',(17.1222287365697,-13.4544851484583,0.));
#8507=CARTESIAN_POINT('Ctrl Pts',(17.1737941556239,-13.4614443545811,0.));
#8508=CARTESIAN_POINT('Ctrl Pts',(17.235798381426,-13.4695161752401,0.));
#8509=CARTESIAN_POINT('Ctrl Pts',(17.287598725272,-13.4759526005425,0.));
#8510=CARTESIAN_POINT('Ctrl Pts',(17.3291218739796,-13.4809165957478,0.));
#8511=CARTESIAN_POINT('Ctrl Pts',(17.360310805254,-13.4845355519784,0.));
#8512=CARTESIAN_POINT('Ctrl Pts',(17.3811241238545,-13.4869019493419,0.));
#8513=CARTESIAN_POINT('Ctrl Pts',(14.1074595503134,-12.4172651441477,13.));
#8514=CARTESIAN_POINT('Ctrl Pts',(14.1180860484761,-12.4266184968736,13.));
#8515=CARTESIAN_POINT('Ctrl Pts',(14.1292464564073,-12.4359861199749,13.));
#8516=CARTESIAN_POINT('Ctrl Pts',(14.1409284550598,-12.445307812124,13.));
#8517=CARTESIAN_POINT('Ctrl Pts',(14.1528807347634,-12.4548451759939,13.));
#8518=CARTESIAN_POINT('Ctrl Pts',(14.1653792068345,-12.4643342258775,13.));
#8519=CARTESIAN_POINT('Ctrl Pts',(14.1783758854621,-12.4737554908686,13.));
#8520=CARTESIAN_POINT('Ctrl Pts',(14.1924534932842,-12.4839603191584,13.));
#8521=CARTESIAN_POINT('Ctrl Pts',(14.2071153071741,-12.4940860551492,13.));
#8522=CARTESIAN_POINT('Ctrl Pts',(14.2222596346423,-12.5041603567402,13.));
#8523=CARTESIAN_POINT('Ctrl Pts',(14.2425470972603,-12.5176559720034,13.));
#8524=CARTESIAN_POINT('Ctrl Pts',(14.263696154001,-12.5310650489192,13.));
#8525=CARTESIAN_POINT('Ctrl Pts',(14.2854153020687,-12.5445127338131,13.));
#8526=CARTESIAN_POINT('Ctrl Pts',(14.3006710264832,-12.5539585083028,13.));
#8527=CARTESIAN_POINT('Ctrl Pts',(14.3162064779772,-12.5634252742744,13.));
#8528=CARTESIAN_POINT('Ctrl Pts',(14.3319443081693,-12.5729244441011,13.));
#8529=CARTESIAN_POINT('Ctrl Pts',(14.3490377565112,-12.5832418491526,13.));
#8530=CARTESIAN_POINT('Ctrl Pts',(14.3663701856948,-12.5935971521702,13.));
#8531=CARTESIAN_POINT('Ctrl Pts',(14.3838818725371,-12.603952675227,13.));
#8532=CARTESIAN_POINT('Ctrl Pts',(14.4097088777849,-12.6192254556702,13.));
#8533=CARTESIAN_POINT('Ctrl Pts',(14.4359272218094,-12.6344967052057,13.));
#8534=CARTESIAN_POINT('Ctrl Pts',(14.4624310404448,-12.6495328172899,13.));
#8535=CARTESIAN_POINT('Ctrl Pts',(14.4814589433508,-12.6603277025386,13.));
#8536=CARTESIAN_POINT('Ctrl Pts',(14.50063705981,-12.6709973404779,13.));
#8537=CARTESIAN_POINT('Ctrl Pts',(14.5199130488615,-12.6814735010565,13.));
#8538=CARTESIAN_POINT('Ctrl Pts',(14.5408480305397,-12.6928512949111,13.));
#8539=CARTESIAN_POINT('Ctrl Pts',(14.561898127647,-12.7040013081349,13.));
#8540=CARTESIAN_POINT('Ctrl Pts',(14.5829561351059,-12.7148903419541,13.));
#8541=CARTESIAN_POINT('Ctrl Pts',(14.6211007133001,-12.7346147913249,13.));
#8542=CARTESIAN_POINT('Ctrl Pts',(14.6592670224042,-12.7534882591773,13.));
#8543=CARTESIAN_POINT('Ctrl Pts',(14.6966913606211,-12.7714870012811,13.));
#8544=CARTESIAN_POINT('Ctrl Pts',(14.7236044494553,-12.7844304965631,13.));
#8545=CARTESIAN_POINT('Ctrl Pts',(14.7501320324422,-12.7969241359761,13.));
#8546=CARTESIAN_POINT('Ctrl Pts',(14.7760241380399,-12.8089152121945,13.));
#8547=CARTESIAN_POINT('Ctrl Pts',(14.79015789262,-12.815460795279,13.));
#8548=CARTESIAN_POINT('Ctrl Pts',(14.804103015233,-12.8218556822256,13.));
#8549=CARTESIAN_POINT('Ctrl Pts',(14.817821671297,-12.8280877109818,13.));
#8550=CARTESIAN_POINT('Ctrl Pts',(14.8203721510302,-12.8292463276105,13.));
#8551=CARTESIAN_POINT('Ctrl Pts',(14.8229148051886,-12.8303993130268,13.));
#8552=CARTESIAN_POINT('Ctrl Pts',(14.8254493925092,-12.8315465871292,13.));
#8553=CARTESIAN_POINT('Ctrl Pts',(14.8277305341092,-12.832579139711,13.));
#8554=CARTESIAN_POINT('Ctrl Pts',(14.8300032273041,-12.8336062098177,13.));
#8555=CARTESIAN_POINT('Ctrl Pts',(14.8322881977108,-12.8346371473846,13.));
#8556=CARTESIAN_POINT('Ctrl Pts',(14.8691293241314,-12.8512592012736,13.));
#8557=CARTESIAN_POINT('Ctrl Pts',(14.9079857431047,-12.8683541689141,13.));
#8558=CARTESIAN_POINT('Ctrl Pts',(14.9490190997324,-12.8857980615984,13.));
#8559=CARTESIAN_POINT('Ctrl Pts',(14.9855964769819,-12.9013476509045,13.));
#8560=CARTESIAN_POINT('Ctrl Pts',(15.0239050647886,-12.9171725830662,13.));
#8561=CARTESIAN_POINT('Ctrl Pts',(15.064023510322,-12.9332300933654,13.));
#8562=CARTESIAN_POINT('Ctrl Pts',(15.1048519750733,-12.9495717906701,13.));
#8563=CARTESIAN_POINT('Ctrl Pts',(15.1475508470956,-12.9661598906376,13.));
#8564=CARTESIAN_POINT('Ctrl Pts',(15.1921895453309,-12.9829638510743,13.));
#8565=CARTESIAN_POINT('Ctrl Pts',(15.2412011844821,-13.0014139779327,13.));
#8566=CARTESIAN_POINT('Ctrl Pts',(15.2925510989723,-13.0201247782342,13.));
#8567=CARTESIAN_POINT('Ctrl Pts',(15.346375635884,-13.0389903700256,13.));
#8568=CARTESIAN_POINT('Ctrl Pts',(15.4033983407683,-13.0589769251344,13.));
#8569=CARTESIAN_POINT('Ctrl Pts',(15.463204290969,-13.0791295844046,13.));
#8570=CARTESIAN_POINT('Ctrl Pts',(15.5259445689097,-13.0993286205218,13.));
#8571=CARTESIAN_POINT('Ctrl Pts',(15.5603875849943,-13.1104174417498,13.));
#8572=CARTESIAN_POINT('Ctrl Pts',(15.5957139525594,-13.1215213991741,13.));
#8573=CARTESIAN_POINT('Ctrl Pts',(15.6319463225903,-13.1326225390231,13.));
#8574=CARTESIAN_POINT('Ctrl Pts',(15.7414124455009,-13.1661615743695,13.));
#8575=CARTESIAN_POINT('Ctrl Pts',(15.8520448442677,-13.1975021501202,13.));
#8576=CARTESIAN_POINT('Ctrl Pts',(15.9635479480078,-13.2267056266809,13.));
#8577=CARTESIAN_POINT('Ctrl Pts',(16.0693084576609,-13.2544050759436,13.));
#8578=CARTESIAN_POINT('Ctrl Pts',(16.1758473117503,-13.2801884271853,13.));
#8579=CARTESIAN_POINT('Ctrl Pts',(16.2829053991411,-13.3041300678694,13.));
#8580=CARTESIAN_POINT('Ctrl Pts',(16.4340206583829,-13.337924312908,13.));
#8581=CARTESIAN_POINT('Ctrl Pts',(16.5861745378189,-13.3680402223278,13.));
#8582=CARTESIAN_POINT('Ctrl Pts',(16.7386734005371,-13.394678434022,13.));
#8583=CARTESIAN_POINT('Ctrl Pts',(16.8568706863481,-13.415324911412,13.));
#8584=CARTESIAN_POINT('Ctrl Pts',(16.9752796560061,-13.4338812595667,13.));
#8585=CARTESIAN_POINT('Ctrl Pts',(17.0935769510192,-13.4504489425771,13.));
#8586=CARTESIAN_POINT('Ctrl Pts',(17.1895488140305,-13.4638899211228,13.));
#8587=CARTESIAN_POINT('Ctrl Pts',(17.2854448391807,-13.4760235684317,13.));
#8588=CARTESIAN_POINT('Ctrl Pts',(17.3811241238545,-13.4869019493419,13.));
#8589=CARTESIAN_POINT('Ctrl Pts',(13.4869019493419,-17.3811241238545,0.));
#8590=CARTESIAN_POINT('Ctrl Pts',(13.4869019493419,-17.3811241238545,21.));
#8591=CARTESIAN_POINT('Ctrl Pts',(13.485718750657,-17.3707174645609,0.));
#8592=CARTESIAN_POINT('Ctrl Pts',(13.485718750657,-17.3707174645609,21.));
#8593=CARTESIAN_POINT('Ctrl Pts',(13.4833292332349,-17.3499144948292,0.));
#8594=CARTESIAN_POINT('Ctrl Pts',(13.4833292332349,-17.3499144948292,21.));
#8595=CARTESIAN_POINT('Ctrl Pts',(13.4796755969465,-17.3187410868027,0.));
#8596=CARTESIAN_POINT('Ctrl Pts',(13.4796755969465,-17.3187410868027,21.));
#8597=CARTESIAN_POINT('Ctrl Pts',(13.474665315482,-17.2772386565028,0.));
#8598=CARTESIAN_POINT('Ctrl Pts',(13.474665315482,-17.2772386565028,21.));
#8599=CARTESIAN_POINT('Ctrl Pts',(13.4681708717968,-17.2254643437923,0.));
#8600=CARTESIAN_POINT('Ctrl Pts',(13.4681708717968,-17.2254643437923,21.));
#8601=CARTESIAN_POINT('Ctrl Pts',(13.4614443545811,-17.173794155624,0.));
#8602=CARTESIAN_POINT('Ctrl Pts',(13.4614443545811,-17.173794155624,21.));
#8603=CARTESIAN_POINT('Ctrl Pts',(13.4544851484583,-17.1222287365697,0.));
#8604=CARTESIAN_POINT('Ctrl Pts',(13.4544851484583,-17.1222287365697,21.));
#8605=CARTESIAN_POINT('Ctrl Pts',(13.4472925380889,-17.0707690194412,0.));
#8606=CARTESIAN_POINT('Ctrl Pts',(13.4472925380889,-17.0707690194412,21.));
#8607=CARTESIAN_POINT('Ctrl Pts',(13.4398657451291,-17.0194162803447,0.));
#8608=CARTESIAN_POINT('Ctrl Pts',(13.4398657451291,-17.0194162803447,21.));
#8609=CARTESIAN_POINT('Ctrl Pts',(13.432203941793,-16.9681720567298,0.));
#8610=CARTESIAN_POINT('Ctrl Pts',(13.432203941793,-16.9681720567298,21.));
#8611=CARTESIAN_POINT('Ctrl Pts',(13.4243062623592,-16.9170380509036,0.));
#8612=CARTESIAN_POINT('Ctrl Pts',(13.4243062623592,-16.9170380509036,21.));
#8613=CARTESIAN_POINT('Ctrl Pts',(13.4161718177499,-16.8660160353187,0.));
#8614=CARTESIAN_POINT('Ctrl Pts',(13.4161718177499,-16.8660160353187,21.));
#8615=CARTESIAN_POINT('Ctrl Pts',(13.4077997088426,-16.8151077630226,0.));
#8616=CARTESIAN_POINT('Ctrl Pts',(13.4077997088426,-16.8151077630226,21.));
#8617=CARTESIAN_POINT('Ctrl Pts',(13.3991890464165,-16.7643148579873,0.));
#8618=CARTESIAN_POINT('Ctrl Pts',(13.3991890464165,-16.7643148579873,21.));
#8619=CARTESIAN_POINT('Ctrl Pts',(13.3903389370346,-16.7136388432444,0.));
#8620=CARTESIAN_POINT('Ctrl Pts',(13.3903389370346,-16.7136388432444,21.));
#8621=CARTESIAN_POINT('Ctrl Pts',(13.381248462113,-16.6630812012276,0.));
#8622=CARTESIAN_POINT('Ctrl Pts',(13.381248462113,-16.6630812012276,21.));
#8623=CARTESIAN_POINT('Ctrl Pts',(13.3719166600676,-16.612643424234,0.));
#8624=CARTESIAN_POINT('Ctrl Pts',(13.3719166600676,-16.612643424234,21.));
#8625=CARTESIAN_POINT('Ctrl Pts',(13.3623425108873,-16.5623270636327,0.));
#8626=CARTESIAN_POINT('Ctrl Pts',(13.3623425108873,-16.5623270636327,21.));
#8627=CARTESIAN_POINT('Ctrl Pts',(13.3525249163084,-16.5121337902953,0.));
#8628=CARTESIAN_POINT('Ctrl Pts',(13.3525249163084,-16.5121337902953,21.));
#8629=CARTESIAN_POINT('Ctrl Pts',(13.3424627129921,-16.4620653818862,0.));
#8630=CARTESIAN_POINT('Ctrl Pts',(13.3424627129921,-16.4620653818862,21.));
#8631=CARTESIAN_POINT('Ctrl Pts',(13.3321546976812,-16.4121236828756,0.));
#8632=CARTESIAN_POINT('Ctrl Pts',(13.3321546976812,-16.4121236828756,21.));
#8633=CARTESIAN_POINT('Ctrl Pts',(13.3215996524974,-16.3623105703343,0.));
#8634=CARTESIAN_POINT('Ctrl Pts',(13.3215996524974,-16.3623105703343,21.));
#8635=CARTESIAN_POINT('Ctrl Pts',(13.3107963665229,-16.3126279218067,0.));
#8636=CARTESIAN_POINT('Ctrl Pts',(13.3107963665229,-16.3126279218067,21.));
#8637=CARTESIAN_POINT('Ctrl Pts',(13.2997436744733,-16.2630775678735,0.));
#8638=CARTESIAN_POINT('Ctrl Pts',(13.2997436744733,-16.2630775678735,21.));
#8639=CARTESIAN_POINT('Ctrl Pts',(13.2884404210387,-16.2136613184475,0.));
#8640=CARTESIAN_POINT('Ctrl Pts',(13.2884404210387,-16.2136613184475,21.));
#8641=CARTESIAN_POINT('Ctrl Pts',(13.2768853909882,-16.1643810242643,0.));
#8642=CARTESIAN_POINT('Ctrl Pts',(13.2768853909882,-16.1643810242643,21.));
#8643=CARTESIAN_POINT('Ctrl Pts',(13.2650772466062,-16.1152386305152,0.));
#8644=CARTESIAN_POINT('Ctrl Pts',(13.2650772466062,-16.1152386305152,21.));
#8645=CARTESIAN_POINT('Ctrl Pts',(13.2530144750236,-16.0662362238032,0.));
#8646=CARTESIAN_POINT('Ctrl Pts',(13.2530144750236,-16.0662362238032,21.));
#8647=CARTESIAN_POINT('Ctrl Pts',(13.240695304984,-16.0173761036734,0.));
#8648=CARTESIAN_POINT('Ctrl Pts',(13.240695304984,-16.0173761036734,21.));
#8649=CARTESIAN_POINT('Ctrl Pts',(13.2281177675127,-15.9686607385389,0.));
#8650=CARTESIAN_POINT('Ctrl Pts',(13.2281177675127,-15.9686607385389,21.));
#8651=CARTESIAN_POINT('Ctrl Pts',(13.2152798388134,-15.9200926550954,0.));
#8652=CARTESIAN_POINT('Ctrl Pts',(13.2152798388134,-15.9200926550954,21.));
#8653=CARTESIAN_POINT('Ctrl Pts',(13.2021795724682,-15.8716743375555,0.));
#8654=CARTESIAN_POINT('Ctrl Pts',(13.2021795724682,-15.8716743375555,21.));
#8655=CARTESIAN_POINT('Ctrl Pts',(13.1888152101588,-15.8234081427091,0.));
#8656=CARTESIAN_POINT('Ctrl Pts',(13.1888152101588,-15.8234081427091,21.));
#8657=CARTESIAN_POINT('Ctrl Pts',(13.1751853728467,-15.7752961549278,0.));
#8658=CARTESIAN_POINT('Ctrl Pts',(13.1751853728467,-15.7752961549278,21.));
#8659=CARTESIAN_POINT('Ctrl Pts',(13.161288914421,-15.7273402954914,0.));
#8660=CARTESIAN_POINT('Ctrl Pts',(13.161288914421,-15.7273402954914,21.));
#8661=CARTESIAN_POINT('Ctrl Pts',(13.147124558532,-15.6795425955901,0.));
#8662=CARTESIAN_POINT('Ctrl Pts',(13.147124558532,-15.6795425955901,21.));
#8663=CARTESIAN_POINT('Ctrl Pts',(13.1326905726717,-15.6319054413079,0.));
#8664=CARTESIAN_POINT('Ctrl Pts',(13.1326905726717,-15.6319054413079,21.));
#8665=CARTESIAN_POINT('Ctrl Pts',(13.1179844917497,-15.5844317820184,0.));
#8666=CARTESIAN_POINT('Ctrl Pts',(13.1179844917497,-15.5844317820184,21.));
#8667=CARTESIAN_POINT('Ctrl Pts',(13.1030026646917,-15.5371254712111,0.));
#8668=CARTESIAN_POINT('Ctrl Pts',(13.1030026646917,-15.5371254712111,21.));
#8669=CARTESIAN_POINT('Ctrl Pts',(13.087740560189,-15.4899910401523,0.));
#8670=CARTESIAN_POINT('Ctrl Pts',(13.087740560189,-15.4899910401523,21.));
#8671=CARTESIAN_POINT('Ctrl Pts',(13.0721935806302,-15.4430330918328,0.));
#8672=CARTESIAN_POINT('Ctrl Pts',(13.0721935806302,-15.4430330918328,21.));
#8673=CARTESIAN_POINT('Ctrl Pts',(13.0563577967298,-15.3962557545684,0.));
#8674=CARTESIAN_POINT('Ctrl Pts',(13.0563577967298,-15.3962557545684,21.));
#8675=CARTESIAN_POINT('Ctrl Pts',(13.0402305665115,-15.3496622219036,0.));
#8676=CARTESIAN_POINT('Ctrl Pts',(13.0402305665115,-15.3496622219036,21.));
#8677=CARTESIAN_POINT('Ctrl Pts',(13.0238115816728,-15.3032539741328,0.));
#8678=CARTESIAN_POINT('Ctrl Pts',(13.0238115816728,-15.3032539741328,21.));
#8679=CARTESIAN_POINT('Ctrl Pts',(13.0071020851025,-15.2570313635503,0.));
#8680=CARTESIAN_POINT('Ctrl Pts',(13.0071020851025,-15.2570313635503,21.));
#8681=CARTESIAN_POINT('Ctrl Pts',(12.9901029059182,-15.2109950816083,0.));
#8682=CARTESIAN_POINT('Ctrl Pts',(12.9901029059182,-15.2109950816083,21.));
#8683=CARTESIAN_POINT('Ctrl Pts',(12.9728126886697,-15.1651474813659,0.));
#8684=CARTESIAN_POINT('Ctrl Pts',(12.9728126886697,-15.1651474813659,21.));
#8685=CARTESIAN_POINT('Ctrl Pts',(12.9552263908864,-15.1194937003528,0.));
#8686=CARTESIAN_POINT('Ctrl Pts',(12.9552263908864,-15.1194937003528,21.));
#8687=CARTESIAN_POINT('Ctrl Pts',(12.9373327960422,-15.0740435169624,0.));
#8688=CARTESIAN_POINT('Ctrl Pts',(12.9373327960422,-15.0740435169624,21.));
#8689=CARTESIAN_POINT('Ctrl Pts',(12.9191164383568,-15.0288099208306,0.));
#8690=CARTESIAN_POINT('Ctrl Pts',(12.9191164383568,-15.0288099208306,21.));
#8691=CARTESIAN_POINT('Ctrl Pts',(12.9005620742036,-14.9838057866976,0.));
#8692=CARTESIAN_POINT('Ctrl Pts',(12.9005620742036,-14.9838057866976,21.));
#8693=CARTESIAN_POINT('Ctrl Pts',(12.8816587472147,-14.9390408507356,0.));
#8694=CARTESIAN_POINT('Ctrl Pts',(12.8816587472147,-14.9390408507356,21.));
#8695=CARTESIAN_POINT('Ctrl Pts',(12.8624032236317,-14.8945191569251,0.));
#8696=CARTESIAN_POINT('Ctrl Pts',(12.8624032236317,-14.8945191569251,21.));
#8697=CARTESIAN_POINT('Ctrl Pts',(12.8428057266944,-14.8502347891476,0.));
#8698=CARTESIAN_POINT('Ctrl Pts',(12.8428057266944,-14.8502347891476,21.));
#8699=CARTESIAN_POINT('Ctrl Pts',(12.822884601679,-14.8061758577898,0.));
#8700=CARTESIAN_POINT('Ctrl Pts',(12.822884601679,-14.8061758577898,21.));
#8701=CARTESIAN_POINT('Ctrl Pts',(12.8026557145457,-14.7623324139791,0.));
#8702=CARTESIAN_POINT('Ctrl Pts',(12.8026557145457,-14.7623324139791,21.));
#8703=CARTESIAN_POINT('Ctrl Pts',(12.7821227233337,-14.7187037124277,0.));
#8704=CARTESIAN_POINT('Ctrl Pts',(12.7821227233337,-14.7187037124277,21.));
#8705=CARTESIAN_POINT('Ctrl Pts',(12.7612687078867,-14.6753044633399,0.));
#8706=CARTESIAN_POINT('Ctrl Pts',(12.7612687078867,-14.6753044633399,21.));
#8707=CARTESIAN_POINT('Ctrl Pts',(12.7400427996251,-14.6321748083434,0.));
#8708=CARTESIAN_POINT('Ctrl Pts',(12.7400427996251,-14.6321748083434,21.));
#8709=CARTESIAN_POINT('Ctrl Pts',(12.7183743139638,-14.5893698147583,0.));
#8710=CARTESIAN_POINT('Ctrl Pts',(12.7183743139638,-14.5893698147583,21.));
#8711=CARTESIAN_POINT('Ctrl Pts',(12.6961966430455,-14.5469417071952,0.));
#8712=CARTESIAN_POINT('Ctrl Pts',(12.6961966430455,-14.5469417071952,21.));
#8713=CARTESIAN_POINT('Ctrl Pts',(12.6734695081852,-14.5049233087958,0.));
#8714=CARTESIAN_POINT('Ctrl Pts',(12.6734695081852,-14.5049233087958,21.));
#8715=CARTESIAN_POINT('Ctrl Pts',(12.6501984687124,-14.463313553928,0.));
#8716=CARTESIAN_POINT('Ctrl Pts',(12.6501984687124,-14.463313553928,21.));
#8717=CARTESIAN_POINT('Ctrl Pts',(12.626464614311,-14.4220553460485,0.));
#8718=CARTESIAN_POINT('Ctrl Pts',(12.626464614311,-14.4220553460485,21.));
#8719=CARTESIAN_POINT('Ctrl Pts',(12.6023830189244,-14.3810669346235,0.));
#8720=CARTESIAN_POINT('Ctrl Pts',(12.6023830189244,-14.3810669346235,21.));
#8721=CARTESIAN_POINT('Ctrl Pts',(12.5780443898087,-14.3402859058353,0.));
#8722=CARTESIAN_POINT('Ctrl Pts',(12.5780443898087,-14.3402859058353,21.));
#8723=CARTESIAN_POINT('Ctrl Pts',(12.5534605602317,-14.2997103098726,0.));
#8724=CARTESIAN_POINT('Ctrl Pts',(12.5534605602317,-14.2997103098726,21.));
#8725=CARTESIAN_POINT('Ctrl Pts',(12.5285125321527,-14.2594378207584,0.));
#8726=CARTESIAN_POINT('Ctrl Pts',(12.5285125321527,-14.2594378207584,21.));
#8727=CARTESIAN_POINT('Ctrl Pts',(12.502885965175,-14.2197144660135,0.));
#8728=CARTESIAN_POINT('Ctrl Pts',(12.502885965175,-14.2197144660135,21.));
#8729=CARTESIAN_POINT('Ctrl Pts',(12.4761570639125,-14.1808688343892,0.));
#8730=CARTESIAN_POINT('Ctrl Pts',(12.4761570639125,-14.1808688343892,21.));
#8731=CARTESIAN_POINT('Ctrl Pts',(12.4535485619996,-14.1507598477672,0.));
#8732=CARTESIAN_POINT('Ctrl Pts',(12.4535485619996,-14.1507598477672,21.));
#8733=CARTESIAN_POINT('Ctrl Pts',(12.4357509724316,-14.1288394445866,0.));
#8734=CARTESIAN_POINT('Ctrl Pts',(12.4357509724316,-14.1288394445866,21.));
#8735=CARTESIAN_POINT('Ctrl Pts',(12.4234926340671,-14.1145347042316,0.));
#8736=CARTESIAN_POINT('Ctrl Pts',(12.4234926340671,-14.1145347042316,21.));
#8737=CARTESIAN_POINT('Ctrl Pts',(12.4172651441477,-14.1074595503134,0.));
#8738=CARTESIAN_POINT('Ctrl Pts',(12.4172651441477,-14.1074595503134,21.));
#8739=CARTESIAN_POINT('',(13.4869019493419,-17.3811241238545,0.));
#8740=CARTESIAN_POINT('Ctrl Pts',(12.4172651441477,-14.1074595503134,0.));
#8741=CARTESIAN_POINT('Ctrl Pts',(12.4234926340671,-14.1145347042316,0.));
#8742=CARTESIAN_POINT('Ctrl Pts',(12.4357509724316,-14.1288394445866,0.));
#8743=CARTESIAN_POINT('Ctrl Pts',(12.4535485619996,-14.1507598477672,0.));
#8744=CARTESIAN_POINT('Ctrl Pts',(12.4761570639125,-14.1808688343892,0.));
#8745=CARTESIAN_POINT('Ctrl Pts',(12.502885965175,-14.2197144660135,0.));
#8746=CARTESIAN_POINT('Ctrl Pts',(12.5285125321527,-14.2594378207584,0.));
#8747=CARTESIAN_POINT('Ctrl Pts',(12.5534605602317,-14.2997103098726,0.));
#8748=CARTESIAN_POINT('Ctrl Pts',(12.5780443898087,-14.3402859058353,0.));
#8749=CARTESIAN_POINT('Ctrl Pts',(12.6023830189244,-14.3810669346235,0.));
#8750=CARTESIAN_POINT('Ctrl Pts',(12.626464614311,-14.4220553460485,0.));
#8751=CARTESIAN_POINT('Ctrl Pts',(12.6501984687124,-14.463313553928,0.));
#8752=CARTESIAN_POINT('Ctrl Pts',(12.6734695081852,-14.5049233087958,0.));
#8753=CARTESIAN_POINT('Ctrl Pts',(12.6961966430455,-14.5469417071952,0.));
#8754=CARTESIAN_POINT('Ctrl Pts',(12.7183743139638,-14.5893698147583,0.));
#8755=CARTESIAN_POINT('Ctrl Pts',(12.7400427996251,-14.6321748083434,0.));
#8756=CARTESIAN_POINT('Ctrl Pts',(12.7612687078867,-14.6753044633399,0.));
#8757=CARTESIAN_POINT('Ctrl Pts',(12.7821227233337,-14.7187037124277,0.));
#8758=CARTESIAN_POINT('Ctrl Pts',(12.8026557145457,-14.7623324139791,0.));
#8759=CARTESIAN_POINT('Ctrl Pts',(12.822884601679,-14.8061758577898,0.));
#8760=CARTESIAN_POINT('Ctrl Pts',(12.8428057266944,-14.8502347891476,0.));
#8761=CARTESIAN_POINT('Ctrl Pts',(12.8624032236317,-14.8945191569251,0.));
#8762=CARTESIAN_POINT('Ctrl Pts',(12.8816587472147,-14.9390408507356,0.));
#8763=CARTESIAN_POINT('Ctrl Pts',(12.9005620742036,-14.9838057866976,0.));
#8764=CARTESIAN_POINT('Ctrl Pts',(12.9191164383568,-15.0288099208306,0.));
#8765=CARTESIAN_POINT('Ctrl Pts',(12.9373327960422,-15.0740435169624,0.));
#8766=CARTESIAN_POINT('Ctrl Pts',(12.9552263908864,-15.1194937003528,0.));
#8767=CARTESIAN_POINT('Ctrl Pts',(12.9728126886697,-15.1651474813659,0.));
#8768=CARTESIAN_POINT('Ctrl Pts',(12.9901029059182,-15.2109950816083,0.));
#8769=CARTESIAN_POINT('Ctrl Pts',(13.0071020851025,-15.2570313635503,0.));
#8770=CARTESIAN_POINT('Ctrl Pts',(13.0238115816728,-15.3032539741328,0.));
#8771=CARTESIAN_POINT('Ctrl Pts',(13.0402305665115,-15.3496622219036,0.));
#8772=CARTESIAN_POINT('Ctrl Pts',(13.0563577967298,-15.3962557545684,0.));
#8773=CARTESIAN_POINT('Ctrl Pts',(13.0721935806302,-15.4430330918328,0.));
#8774=CARTESIAN_POINT('Ctrl Pts',(13.087740560189,-15.4899910401523,0.));
#8775=CARTESIAN_POINT('Ctrl Pts',(13.1030026646917,-15.5371254712111,0.));
#8776=CARTESIAN_POINT('Ctrl Pts',(13.1179844917497,-15.5844317820184,0.));
#8777=CARTESIAN_POINT('Ctrl Pts',(13.1326905726717,-15.6319054413079,0.));
#8778=CARTESIAN_POINT('Ctrl Pts',(13.147124558532,-15.6795425955901,0.));
#8779=CARTESIAN_POINT('Ctrl Pts',(13.161288914421,-15.7273402954914,0.));
#8780=CARTESIAN_POINT('Ctrl Pts',(13.1751853728467,-15.7752961549278,0.));
#8781=CARTESIAN_POINT('Ctrl Pts',(13.1888152101588,-15.8234081427091,0.));
#8782=CARTESIAN_POINT('Ctrl Pts',(13.2021795724682,-15.8716743375555,0.));
#8783=CARTESIAN_POINT('Ctrl Pts',(13.2152798388134,-15.9200926550954,0.));
#8784=CARTESIAN_POINT('Ctrl Pts',(13.2281177675127,-15.9686607385389,0.));
#8785=CARTESIAN_POINT('Ctrl Pts',(13.240695304984,-16.0173761036734,0.));
#8786=CARTESIAN_POINT('Ctrl Pts',(13.2530144750236,-16.0662362238032,0.));
#8787=CARTESIAN_POINT('Ctrl Pts',(13.2650772466062,-16.1152386305152,0.));
#8788=CARTESIAN_POINT('Ctrl Pts',(13.2768853909882,-16.1643810242643,0.));
#8789=CARTESIAN_POINT('Ctrl Pts',(13.2884404210387,-16.2136613184475,0.));
#8790=CARTESIAN_POINT('Ctrl Pts',(13.2997436744733,-16.2630775678735,0.));
#8791=CARTESIAN_POINT('Ctrl Pts',(13.3107963665229,-16.3126279218067,0.));
#8792=CARTESIAN_POINT('Ctrl Pts',(13.3215996524974,-16.3623105703343,0.));
#8793=CARTESIAN_POINT('Ctrl Pts',(13.3321546976812,-16.4121236828756,0.));
#8794=CARTESIAN_POINT('Ctrl Pts',(13.3424627129921,-16.4620653818862,0.));
#8795=CARTESIAN_POINT('Ctrl Pts',(13.3525249163084,-16.5121337902953,0.));
#8796=CARTESIAN_POINT('Ctrl Pts',(13.3623425108873,-16.5623270636327,0.));
#8797=CARTESIAN_POINT('Ctrl Pts',(13.3719166600676,-16.612643424234,0.));
#8798=CARTESIAN_POINT('Ctrl Pts',(13.381248462113,-16.6630812012276,0.));
#8799=CARTESIAN_POINT('Ctrl Pts',(13.3903389370346,-16.7136388432444,0.));
#8800=CARTESIAN_POINT('Ctrl Pts',(13.3991890464165,-16.7643148579873,0.));
#8801=CARTESIAN_POINT('Ctrl Pts',(13.4077997088426,-16.8151077630226,0.));
#8802=CARTESIAN_POINT('Ctrl Pts',(13.4161718177499,-16.8660160353187,0.));
#8803=CARTESIAN_POINT('Ctrl Pts',(13.4243062623592,-16.9170380509036,0.));
#8804=CARTESIAN_POINT('Ctrl Pts',(13.432203941793,-16.9681720567298,0.));
#8805=CARTESIAN_POINT('Ctrl Pts',(13.4398657451291,-17.0194162803447,0.));
#8806=CARTESIAN_POINT('Ctrl Pts',(13.4472925380889,-17.0707690194412,0.));
#8807=CARTESIAN_POINT('Ctrl Pts',(13.4544851484583,-17.1222287365697,0.));
#8808=CARTESIAN_POINT('Ctrl Pts',(13.4614443545811,-17.173794155624,0.));
#8809=CARTESIAN_POINT('Ctrl Pts',(13.4695161752399,-17.235798381426,0.));
#8810=CARTESIAN_POINT('Ctrl Pts',(13.4759526005425,-17.287598725272,0.));
#8811=CARTESIAN_POINT('Ctrl Pts',(13.4809165957478,-17.3291218739796,0.));
#8812=CARTESIAN_POINT('Ctrl Pts',(13.4845355519784,-17.360310805254,0.));
#8813=CARTESIAN_POINT('Ctrl Pts',(13.4869019493419,-17.3811241238545,0.));
#8814=CARTESIAN_POINT('',(13.4869019493419,-17.3811241238545,13.));
#8815=CARTESIAN_POINT('Ctrl Pts',(13.4869019493419,-17.3811241238545,13.));
#8816=CARTESIAN_POINT('Ctrl Pts',(13.475253226354,-17.2786694026925,13.));
#8817=CARTESIAN_POINT('Ctrl Pts',(13.4622625504827,-17.1768129075703,13.));
#8818=CARTESIAN_POINT('Ctrl Pts',(13.4479123002588,-17.0755735571127,13.));
#8819=CARTESIAN_POINT('Ctrl Pts',(13.4241333152838,-16.9078155768783,13.));
#8820=CARTESIAN_POINT('Ctrl Pts',(13.3966181281356,-16.7417653304334,13.));
#8821=CARTESIAN_POINT('Ctrl Pts',(13.365224404591,-16.5776745262699,13.));
#8822=CARTESIAN_POINT('Ctrl Pts',(13.341093348038,-16.4515447134285,13.));
#8823=CARTESIAN_POINT('Ctrl Pts',(13.3146689195875,-16.3265706105421,13.));
#8824=CARTESIAN_POINT('Ctrl Pts',(13.2858665160046,-16.2028831155018,13.));
#8825=CARTESIAN_POINT('Ctrl Pts',(13.2548614253322,-16.0697365193248,13.));
#8826=CARTESIAN_POINT('Ctrl Pts',(13.2211052767355,-15.9380763844706,13.));
#8827=CARTESIAN_POINT('Ctrl Pts',(13.1844379732149,-15.8081115250302,13.));
#8828=CARTESIAN_POINT('Ctrl Pts',(13.1641379552979,-15.7361594390595,13.));
#8829=CARTESIAN_POINT('Ctrl Pts',(13.1429498667048,-15.6647240120097,13.));
#8830=CARTESIAN_POINT('Ctrl Pts',(13.1208442193763,-15.5938437095349,13.));
#8831=CARTESIAN_POINT('Ctrl Pts',(13.0995423541622,-15.5255406814797,13.));
#8832=CARTESIAN_POINT('Ctrl Pts',(13.0773830005582,-15.4577571787722,13.));
#8833=CARTESIAN_POINT('Ctrl Pts',(13.0543129132306,-15.3905488552535,13.));
#8834=CARTESIAN_POINT('Ctrl Pts',(13.0343732800162,-15.3324602446263,13.));
#8835=CARTESIAN_POINT('Ctrl Pts',(13.0137559287811,-15.2747993584641,13.));
#8836=CARTESIAN_POINT('Ctrl Pts',(12.9924643459599,-15.2175748373743,13.));
#8837=CARTESIAN_POINT('Ctrl Pts',(12.9771843404788,-15.1765073881741,13.));
#8838=CARTESIAN_POINT('Ctrl Pts',(12.9615593601403,-15.1356630007799,13.));
#8839=CARTESIAN_POINT('Ctrl Pts',(12.9455599556129,-15.0950681406725,13.));
#8840=CARTESIAN_POINT('Ctrl Pts',(12.9298210808532,-15.055134315759,13.));
#8841=CARTESIAN_POINT('Ctrl Pts',(12.9137147531419,-15.0154457689548,13.));
#8842=CARTESIAN_POINT('Ctrl Pts',(12.8972012565652,-14.9760367892145,13.));
#8843=CARTESIAN_POINT('Ctrl Pts',(12.882883085059,-14.9418668889644,13.));
#8844=CARTESIAN_POINT('Ctrl Pts',(12.8682568221008,-14.9079086467153,13.));
#8845=CARTESIAN_POINT('Ctrl Pts',(12.8533364079406,-14.8741550424562,13.));
#8846=CARTESIAN_POINT('Ctrl Pts',(12.839821936482,-14.8435820223986,13.));
#8847=CARTESIAN_POINT('Ctrl Pts',(12.8260705989223,-14.8131735651743,13.));
#8848=CARTESIAN_POINT('Ctrl Pts',(12.8121025760339,-14.7829174093268,13.));
#8849=CARTESIAN_POINT('Ctrl Pts',(12.8003366511334,-14.7574312213154,13.));
#8850=CARTESIAN_POINT('Ctrl Pts',(12.7884183714705,-14.7320520624089,13.));
#8851=CARTESIAN_POINT('Ctrl Pts',(12.7763327022737,-14.7067929861541,13.));
#8852=CARTESIAN_POINT('Ctrl Pts',(12.7588434233209,-14.6702403531541,13.));
#8853=CARTESIAN_POINT('Ctrl Pts',(12.7410029355634,-14.6339396293391,13.));
#8854=CARTESIAN_POINT('Ctrl Pts',(12.7226389619075,-14.5980256537221,13.));
#8855=CARTESIAN_POINT('Ctrl Pts',(12.7115427371053,-14.5763250373713,13.));
#8856=CARTESIAN_POINT('Ctrl Pts',(12.7002526008255,-14.5547677198027,13.));
#8857=CARTESIAN_POINT('Ctrl Pts',(12.6887481997665,-14.5333705425118,13.));
#8858=CARTESIAN_POINT('Ctrl Pts',(12.6781379055282,-14.5136363255141,13.));
#8859=CARTESIAN_POINT('Ctrl Pts',(12.6673442953663,-14.4940391161015,13.));
#8860=CARTESIAN_POINT('Ctrl Pts',(12.656388173486,-14.4745649057707,13.));
#8861=CARTESIAN_POINT('Ctrl Pts',(12.6413169180704,-14.4477761568762,13.));
#8862=CARTESIAN_POINT('Ctrl Pts',(12.6259439377051,-14.4212156950105,13.));
#8863=CARTESIAN_POINT('Ctrl Pts',(12.6103925841804,-14.3947967980687,13.));
#8864=CARTESIAN_POINT('Ctrl Pts',(12.6005265277414,-14.3780361779808,13.));
#8865=CARTESIAN_POINT('Ctrl Pts',(12.5905900370726,-14.3613315562137,13.));
#8866=CARTESIAN_POINT('Ctrl Pts',(12.5805908896517,-14.3446791501185,13.));
#8867=CARTESIAN_POINT('Ctrl Pts',(12.5716171202699,-14.3297343907646,13.));
#8868=CARTESIAN_POINT('Ctrl Pts',(12.5625934694456,-14.3148312514246,13.));
#8869=CARTESIAN_POINT('Ctrl Pts',(12.5534931964106,-14.2999916563736,13.));
#8870=CARTESIAN_POINT('Ctrl Pts',(12.5439269970518,-14.2843922865399,13.));
#8871=CARTESIAN_POINT('Ctrl Pts',(12.534276259247,-14.2688630443264,13.));
#8872=CARTESIAN_POINT('Ctrl Pts',(12.524460288528,-14.2534670740992,13.));
#8873=CARTESIAN_POINT('Ctrl Pts',(12.5081559827695,-14.2278944014392,13.));
#8874=CARTESIAN_POINT('Ctrl Pts',(12.4913891919205,-14.2026946289112,13.));
#8875=CARTESIAN_POINT('Ctrl Pts',(12.4736648236276,-14.1782508276066,13.));
#8876=CARTESIAN_POINT('Ctrl Pts',(12.4638909761914,-14.1647716456823,13.));
#8877=CARTESIAN_POINT('Ctrl Pts',(12.453824835945,-14.1515231428882,13.));
#8878=CARTESIAN_POINT('Ctrl Pts',(12.4434054355307,-14.138552318439,13.));
#8879=CARTESIAN_POINT('Ctrl Pts',(12.4349297906175,-14.128001221649,13.));
#8880=CARTESIAN_POINT('Ctrl Pts',(12.4262204477597,-14.1176338183186,13.));
#8881=CARTESIAN_POINT('Ctrl Pts',(12.4172651441477,-14.1074595503134,13.));
#8882=CARTESIAN_POINT('',(13.4869019493419,-17.3811241238545,0.));
#8883=CARTESIAN_POINT('Origin',(3.33073116609659E-12,-4.58435815896522E-12,
0.));
#8884=CARTESIAN_POINT('',(12.3627494547115,-18.1978687191668,0.));
#8885=CARTESIAN_POINT('Origin',(3.33073116609659E-12,-4.58435815896522E-12,
0.));
#8886=CARTESIAN_POINT('',(12.3627494547115,-18.1978687191668,13.));
#8887=CARTESIAN_POINT('Origin',(3.33073116609659E-12,-4.58435815896522E-12,
13.));
#8888=CARTESIAN_POINT('',(12.3627494547115,-18.1978687191668,0.));
#8889=CARTESIAN_POINT('Ctrl Pts',(9.57984538049454,-16.1689656784104,0.));
#8890=CARTESIAN_POINT('Ctrl Pts',(9.57984538049454,-16.1689656784104,21.));
#8891=CARTESIAN_POINT('Ctrl Pts',(9.58464985151482,-16.1770747160769,0.));
#8892=CARTESIAN_POINT('Ctrl Pts',(9.58464985151482,-16.1770747160769,21.));
#8893=CARTESIAN_POINT('Ctrl Pts',(9.59446643316596,-16.1931534965272,0.));
#8894=CARTESIAN_POINT('Ctrl Pts',(9.59446643316596,-16.1931534965272,21.));
#8895=CARTESIAN_POINT('Ctrl Pts',(9.60981421781523,-16.2168537871666,0.));
#8896=CARTESIAN_POINT('Ctrl Pts',(9.60981421781523,-16.2168537871666,21.));
#8897=CARTESIAN_POINT('Ctrl Pts',(9.63146315443272,-16.2476599387841,0.));
#8898=CARTESIAN_POINT('Ctrl Pts',(9.63146315443272,-16.2476599387841,21.));
#8899=CARTESIAN_POINT('Ctrl Pts',(9.66014786078746,-16.2850845948324,0.));
#8900=CARTESIAN_POINT('Ctrl Pts',(9.66014786078746,-16.2850845948324,21.));
#8901=CARTESIAN_POINT('Ctrl Pts',(9.69000797146315,-16.3217321000366,0.));
#8902=CARTESIAN_POINT('Ctrl Pts',(9.69000797146315,-16.3217321000366,21.));
#8903=CARTESIAN_POINT('Ctrl Pts',(9.72060002001011,-16.3579039682519,0.));
#8904=CARTESIAN_POINT('Ctrl Pts',(9.72060002001011,-16.3579039682519,21.));
#8905=CARTESIAN_POINT('Ctrl Pts',(9.75159288382684,-16.3938231282759,0.));
#8906=CARTESIAN_POINT('Ctrl Pts',(9.75159288382684,-16.3938231282759,21.));
#8907=CARTESIAN_POINT('Ctrl Pts',(9.78285689698057,-16.4295725710378,0.));
#8908=CARTESIAN_POINT('Ctrl Pts',(9.78285689698057,-16.4295725710378,21.));
#8909=CARTESIAN_POINT('Ctrl Pts',(9.81439757053278,-16.4651416449558,0.));
#8910=CARTESIAN_POINT('Ctrl Pts',(9.81439757053278,-16.4651416449558,21.));
#8911=CARTESIAN_POINT('Ctrl Pts',(9.84630229363521,-16.5004633692332,0.));
#8912=CARTESIAN_POINT('Ctrl Pts',(9.84630229363521,-16.5004633692332,21.));
#8913=CARTESIAN_POINT('Ctrl Pts',(9.87868437546979,-16.5354535643506,0.));
#8914=CARTESIAN_POINT('Ctrl Pts',(9.87868437546979,-16.5354535643506,21.));
#8915=CARTESIAN_POINT('Ctrl Pts',(9.91162317616648,-16.5700527532381,0.));
#8916=CARTESIAN_POINT('Ctrl Pts',(9.91162317616648,-16.5700527532381,21.));
#8917=CARTESIAN_POINT('Ctrl Pts',(9.9451214271291,-16.6042559779574,0.));
#8918=CARTESIAN_POINT('Ctrl Pts',(9.9451214271291,-16.6042559779574,21.));
#8919=CARTESIAN_POINT('Ctrl Pts',(9.97913546489641,-16.6380914029057,0.));
#8920=CARTESIAN_POINT('Ctrl Pts',(9.97913546489641,-16.6380914029057,21.));
#8921=CARTESIAN_POINT('Ctrl Pts',(10.0135950379525,-16.6716062376277,0.));
#8922=CARTESIAN_POINT('Ctrl Pts',(10.0135950379525,-16.6716062376277,21.));
#8923=CARTESIAN_POINT('Ctrl Pts',(10.0484259314257,-16.7048506904207,0.));
#8924=CARTESIAN_POINT('Ctrl Pts',(10.0484259314257,-16.7048506904207,21.));
#8925=CARTESIAN_POINT('Ctrl Pts',(10.0835742491038,-16.7378607357337,0.));
#8926=CARTESIAN_POINT('Ctrl Pts',(10.0835742491038,-16.7378607357337,21.));
#8927=CARTESIAN_POINT('Ctrl Pts',(10.1190207721353,-16.7706479198888,0.));
#8928=CARTESIAN_POINT('Ctrl Pts',(10.1190207721353,-16.7706479198888,21.));
#8929=CARTESIAN_POINT('Ctrl Pts',(10.1547673397274,-16.8032089941901,0.));
#8930=CARTESIAN_POINT('Ctrl Pts',(10.1547673397274,-16.8032089941901,21.));
#8931=CARTESIAN_POINT('Ctrl Pts',(10.1908283166713,-16.8355319435838,0.));
#8932=CARTESIAN_POINT('Ctrl Pts',(10.1908283166713,-16.8355319435838,21.));
#8933=CARTESIAN_POINT('Ctrl Pts',(10.2272206796636,-16.8676029947679,0.));
#8934=CARTESIAN_POINT('Ctrl Pts',(10.2272206796636,-16.8676029947679,21.));
#8935=CARTESIAN_POINT('Ctrl Pts',(10.2639532144219,-16.8994142530447,0.));
#8936=CARTESIAN_POINT('Ctrl Pts',(10.2639532144219,-16.8994142530447,21.));
#8937=CARTESIAN_POINT('Ctrl Pts',(10.3010210756062,-16.9309675442426,0.));
#8938=CARTESIAN_POINT('Ctrl Pts',(10.3010210756062,-16.9309675442426,21.));
#8939=CARTESIAN_POINT('Ctrl Pts',(10.3384116178624,-16.9622702798438,0.));
#8940=CARTESIAN_POINT('Ctrl Pts',(10.3384116178624,-16.9622702798438,21.));
#8941=CARTESIAN_POINT('Ctrl Pts',(10.3761078860454,-16.9933329788855,0.));
#8942=CARTESIAN_POINT('Ctrl Pts',(10.3761078860454,-16.9933329788855,21.));
#8943=CARTESIAN_POINT('Ctrl Pts',(10.4140927470882,-17.0241663361802,0.));
#8944=CARTESIAN_POINT('Ctrl Pts',(10.4140927470882,-17.0241663361802,21.));
#8945=CARTESIAN_POINT('Ctrl Pts',(10.452353435089,-17.0547779975888,0.));
#8946=CARTESIAN_POINT('Ctrl Pts',(10.452353435089,-17.0547779975888,21.));
#8947=CARTESIAN_POINT('Ctrl Pts',(10.4908835057575,-17.0851711712016,0.));
#8948=CARTESIAN_POINT('Ctrl Pts',(10.4908835057575,-17.0851711712016,21.));
#8949=CARTESIAN_POINT('Ctrl Pts',(10.5296803023445,-17.1153464189932,0.));
#8950=CARTESIAN_POINT('Ctrl Pts',(10.5296803023445,-17.1153464189932,21.));
#8951=CARTESIAN_POINT('Ctrl Pts',(10.5687434234512,-17.1453027387554,0.));
#8952=CARTESIAN_POINT('Ctrl Pts',(10.5687434234512,-17.1453027387554,21.));
#8953=CARTESIAN_POINT('Ctrl Pts',(10.6080729180997,-17.1750388395657,0.));
#8954=CARTESIAN_POINT('Ctrl Pts',(10.6080729180997,-17.1750388395657,21.));
#8955=CARTESIAN_POINT('Ctrl Pts',(10.6476672831754,-17.2045545572011,0.));
#8956=CARTESIAN_POINT('Ctrl Pts',(10.6476672831754,-17.2045545572011,21.));
#8957=CARTESIAN_POINT('Ctrl Pts',(10.6875226650217,-17.2338514174708,0.));
#8958=CARTESIAN_POINT('Ctrl Pts',(10.6875226650217,-17.2338514174708,21.));
#8959=CARTESIAN_POINT('Ctrl Pts',(10.7276339231608,-17.2629318816279,0.));
#8960=CARTESIAN_POINT('Ctrl Pts',(10.7276339231608,-17.2629318816279,21.));
#8961=CARTESIAN_POINT('Ctrl Pts',(10.7679952591482,-17.2917988998581,0.));
#8962=CARTESIAN_POINT('Ctrl Pts',(10.7679952591482,-17.2917988998581,21.));
#8963=CARTESIAN_POINT('Ctrl Pts',(10.8086009632423,-17.3204553814537,0.));
#8964=CARTESIAN_POINT('Ctrl Pts',(10.8086009632423,-17.3204553814537,21.));
#8965=CARTESIAN_POINT('Ctrl Pts',(10.8494462423127,-17.3489036079991,0.));
#8966=CARTESIAN_POINT('Ctrl Pts',(10.8494462423127,-17.3489036079991,21.));
#8967=CARTESIAN_POINT('Ctrl Pts',(10.8905275295837,-17.377145012528,0.));
#8968=CARTESIAN_POINT('Ctrl Pts',(10.8905275295837,-17.377145012528,21.));
#8969=CARTESIAN_POINT('Ctrl Pts',(10.9318420203801,-17.4051805054129,0.));
#8970=CARTESIAN_POINT('Ctrl Pts',(10.9318420203801,-17.4051805054129,21.));
#8971=CARTESIAN_POINT('Ctrl Pts',(10.9733873885115,-17.4330106728622,0.));
#8972=CARTESIAN_POINT('Ctrl Pts',(10.9733873885115,-17.4330106728622,21.));
#8973=CARTESIAN_POINT('Ctrl Pts',(11.0151614525642,-17.460636011184,0.));
#8974=CARTESIAN_POINT('Ctrl Pts',(11.0151614525642,-17.460636011184,21.));
#8975=CARTESIAN_POINT('Ctrl Pts',(11.0571618040371,-17.4880571878157,0.));
#8976=CARTESIAN_POINT('Ctrl Pts',(11.0571618040371,-17.4880571878157,21.));
#8977=CARTESIAN_POINT('Ctrl Pts',(11.0993856581394,-17.5152751467292,0.));
#8978=CARTESIAN_POINT('Ctrl Pts',(11.0993856581394,-17.5152751467292,21.));
#8979=CARTESIAN_POINT('Ctrl Pts',(11.1418300507683,-17.5422909714139,0.));
#8980=CARTESIAN_POINT('Ctrl Pts',(11.1418300507683,-17.5422909714139,21.));
#8981=CARTESIAN_POINT('Ctrl Pts',(11.1844919535058,-17.5691058058227,0.));
#8982=CARTESIAN_POINT('Ctrl Pts',(11.1844919535058,-17.5691058058227,21.));
#8983=CARTESIAN_POINT('Ctrl Pts',(11.2273684103051,-17.5957207597803,0.));
#8984=CARTESIAN_POINT('Ctrl Pts',(11.2273684103051,-17.5957207597803,21.));
#8985=CARTESIAN_POINT('Ctrl Pts',(11.2704566868205,-17.6221368072528,0.));
#8986=CARTESIAN_POINT('Ctrl Pts',(11.2704566868205,-17.6221368072528,21.));
#8987=CARTESIAN_POINT('Ctrl Pts',(11.3137543310722,-17.6483547422688,0.));
#8988=CARTESIAN_POINT('Ctrl Pts',(11.3137543310722,-17.6483547422688,21.));
#8989=CARTESIAN_POINT('Ctrl Pts',(11.3572590796967,-17.674375235974,0.));
#8990=CARTESIAN_POINT('Ctrl Pts',(11.3572590796967,-17.674375235974,21.));
#8991=CARTESIAN_POINT('Ctrl Pts',(11.4009687970126,-17.700198872213,0.));
#8992=CARTESIAN_POINT('Ctrl Pts',(11.4009687970126,-17.700198872213,21.));
#8993=CARTESIAN_POINT('Ctrl Pts',(11.4448814046804,-17.725826190457,0.));
#8994=CARTESIAN_POINT('Ctrl Pts',(11.4448814046804,-17.725826190457,21.));
#8995=CARTESIAN_POINT('Ctrl Pts',(11.4889948016216,-17.7512577332768,0.));
#8996=CARTESIAN_POINT('Ctrl Pts',(11.4889948016216,-17.7512577332768,21.));
#8997=CARTESIAN_POINT('Ctrl Pts',(11.5333068279911,-17.7764940721306,0.));
#8998=CARTESIAN_POINT('Ctrl Pts',(11.5333068279911,-17.7764940721306,21.));
#8999=CARTESIAN_POINT('Ctrl Pts',(11.5778153222435,-17.8015357852426,0.));
#9000=CARTESIAN_POINT('Ctrl Pts',(11.5778153222435,-17.8015357852426,21.));
#9001=CARTESIAN_POINT('Ctrl Pts',(11.6225181583564,-17.8263834470057,0.));
#9002=CARTESIAN_POINT('Ctrl Pts',(11.6225181583564,-17.8263834470057,21.));
#9003=CARTESIAN_POINT('Ctrl Pts',(11.6674132861792,-17.8510376144926,0.));
#9004=CARTESIAN_POINT('Ctrl Pts',(11.6674132861792,-17.8510376144926,21.));
#9005=CARTESIAN_POINT('Ctrl Pts',(11.7124987772363,-17.8754988158862,0.));
#9006=CARTESIAN_POINT('Ctrl Pts',(11.7124987772363,-17.8754988158862,21.));
#9007=CARTESIAN_POINT('Ctrl Pts',(11.7577728408871,-17.8997675418752,0.));
#9008=CARTESIAN_POINT('Ctrl Pts',(11.7577728408871,-17.8997675418752,21.));
#9009=CARTESIAN_POINT('Ctrl Pts',(11.8032337607271,-17.9238442458356,0.));
#9010=CARTESIAN_POINT('Ctrl Pts',(11.8032337607271,-17.9238442458356,21.));
#9011=CARTESIAN_POINT('Ctrl Pts',(11.8488798430201,-17.9477293432951,0.));
#9012=CARTESIAN_POINT('Ctrl Pts',(11.8488798430201,-17.9477293432951,21.));
#9013=CARTESIAN_POINT('Ctrl Pts',(11.8947093631895,-17.9714232133203,0.));
#9014=CARTESIAN_POINT('Ctrl Pts',(11.8947093631895,-17.9714232133203,21.));
#9015=CARTESIAN_POINT('Ctrl Pts',(11.9407205019619,-17.9949261997754,0.));
#9016=CARTESIAN_POINT('Ctrl Pts',(11.9407205019619,-17.9949261997754,21.));
#9017=CARTESIAN_POINT('Ctrl Pts',(11.986911314246,-18.0182386160553,0.));
#9018=CARTESIAN_POINT('Ctrl Pts',(11.986911314246,-18.0182386160553,21.));
#9019=CARTESIAN_POINT('Ctrl Pts',(12.0332798395991,-18.0413607600052,0.));
#9020=CARTESIAN_POINT('Ctrl Pts',(12.0332798395991,-18.0413607600052,21.));
#9021=CARTESIAN_POINT('Ctrl Pts',(12.0798241915081,-18.0642929289333,0.));
#9022=CARTESIAN_POINT('Ctrl Pts',(12.0798241915081,-18.0642929289333,21.));
#9023=CARTESIAN_POINT('Ctrl Pts',(12.1265426519718,-18.0870354350128,0.));
#9024=CARTESIAN_POINT('Ctrl Pts',(12.1265426519718,-18.0870354350128,21.));
#9025=CARTESIAN_POINT('Ctrl Pts',(12.1734337668195,-18.109588624154,0.));
#9026=CARTESIAN_POINT('Ctrl Pts',(12.1734337668195,-18.109588624154,21.));
#9027=CARTESIAN_POINT('Ctrl Pts',(12.2204964278426,-18.1319528884305,0.));
#9028=CARTESIAN_POINT('Ctrl Pts',(12.2204964278426,-18.1319528884305,21.));
#9029=CARTESIAN_POINT('Ctrl Pts',(12.2677298318549,-18.1541286139166,0.));
#9030=CARTESIAN_POINT('Ctrl Pts',(12.2677298318549,-18.1541286139166,21.));
#9031=CARTESIAN_POINT('Ctrl Pts',(12.3056527265146,-18.1717186310224,0.));
#9032=CARTESIAN_POINT('Ctrl Pts',(12.3056527265146,-18.1717186310224,21.));
#9033=CARTESIAN_POINT('Ctrl Pts',(12.3341713636489,-18.1848265584754,0.));
#9034=CARTESIAN_POINT('Ctrl Pts',(12.3341713636489,-18.1848265584754,21.));
#9035=CARTESIAN_POINT('Ctrl Pts',(12.3532177620787,-18.1935275957711,0.));
#9036=CARTESIAN_POINT('Ctrl Pts',(12.3532177620787,-18.1935275957711,21.));
#9037=CARTESIAN_POINT('Ctrl Pts',(12.3627494547115,-18.1978687191668,0.));
#9038=CARTESIAN_POINT('Ctrl Pts',(12.3627494547115,-18.1978687191668,21.));
#9039=CARTESIAN_POINT('Ctrl Pts',(9.57984538049454,-16.1689656784104,0.));
#9040=CARTESIAN_POINT('Ctrl Pts',(9.58464985151482,-16.1770747160769,0.));
#9041=CARTESIAN_POINT('Ctrl Pts',(9.59446643316596,-16.1931534965272,0.));
#9042=CARTESIAN_POINT('Ctrl Pts',(9.60981421781523,-16.2168537871666,0.));
#9043=CARTESIAN_POINT('Ctrl Pts',(9.63146315443272,-16.2476599387841,0.));
#9044=CARTESIAN_POINT('Ctrl Pts',(9.66014786078746,-16.2850845948324,0.));
#9045=CARTESIAN_POINT('Ctrl Pts',(9.69000797146315,-16.3217321000366,0.));
#9046=CARTESIAN_POINT('Ctrl Pts',(9.72060002001011,-16.3579039682519,0.));
#9047=CARTESIAN_POINT('Ctrl Pts',(9.75159288382684,-16.3938231282759,0.));
#9048=CARTESIAN_POINT('Ctrl Pts',(9.78285689698057,-16.4295725710378,0.));
#9049=CARTESIAN_POINT('Ctrl Pts',(9.81439757053278,-16.4651416449558,0.));
#9050=CARTESIAN_POINT('Ctrl Pts',(9.84630229363521,-16.5004633692332,0.));
#9051=CARTESIAN_POINT('Ctrl Pts',(9.87868437546979,-16.5354535643506,0.));
#9052=CARTESIAN_POINT('Ctrl Pts',(9.91162317616648,-16.5700527532381,0.));
#9053=CARTESIAN_POINT('Ctrl Pts',(9.9451214271291,-16.6042559779574,0.));
#9054=CARTESIAN_POINT('Ctrl Pts',(9.97913546489641,-16.6380914029057,0.));
#9055=CARTESIAN_POINT('Ctrl Pts',(10.0135950379525,-16.6716062376277,0.));
#9056=CARTESIAN_POINT('Ctrl Pts',(10.0484259314257,-16.7048506904207,0.));
#9057=CARTESIAN_POINT('Ctrl Pts',(10.0835742491038,-16.7378607357337,0.));
#9058=CARTESIAN_POINT('Ctrl Pts',(10.1190207721353,-16.7706479198888,0.));
#9059=CARTESIAN_POINT('Ctrl Pts',(10.1547673397274,-16.8032089941901,0.));
#9060=CARTESIAN_POINT('Ctrl Pts',(10.1908283166713,-16.8355319435838,0.));
#9061=CARTESIAN_POINT('Ctrl Pts',(10.2272206796636,-16.8676029947679,0.));
#9062=CARTESIAN_POINT('Ctrl Pts',(10.2639532144219,-16.8994142530447,0.));
#9063=CARTESIAN_POINT('Ctrl Pts',(10.3010210756062,-16.9309675442426,0.));
#9064=CARTESIAN_POINT('Ctrl Pts',(10.3384116178624,-16.9622702798438,0.));
#9065=CARTESIAN_POINT('Ctrl Pts',(10.3761078860454,-16.9933329788855,0.));
#9066=CARTESIAN_POINT('Ctrl Pts',(10.4140927470882,-17.0241663361802,0.));
#9067=CARTESIAN_POINT('Ctrl Pts',(10.452353435089,-17.0547779975888,0.));
#9068=CARTESIAN_POINT('Ctrl Pts',(10.4908835057575,-17.0851711712016,0.));
#9069=CARTESIAN_POINT('Ctrl Pts',(10.5296803023445,-17.1153464189932,0.));
#9070=CARTESIAN_POINT('Ctrl Pts',(10.5687434234512,-17.1453027387554,0.));
#9071=CARTESIAN_POINT('Ctrl Pts',(10.6080729180997,-17.1750388395657,0.));
#9072=CARTESIAN_POINT('Ctrl Pts',(10.6476672831754,-17.2045545572011,0.));
#9073=CARTESIAN_POINT('Ctrl Pts',(10.6875226650217,-17.2338514174708,0.));
#9074=CARTESIAN_POINT('Ctrl Pts',(10.7276339231608,-17.2629318816279,0.));
#9075=CARTESIAN_POINT('Ctrl Pts',(10.7679952591482,-17.2917988998581,0.));
#9076=CARTESIAN_POINT('Ctrl Pts',(10.8086009632423,-17.3204553814537,0.));
#9077=CARTESIAN_POINT('Ctrl Pts',(10.8494462423127,-17.3489036079991,0.));
#9078=CARTESIAN_POINT('Ctrl Pts',(10.8905275295837,-17.377145012528,0.));
#9079=CARTESIAN_POINT('Ctrl Pts',(10.9318420203801,-17.4051805054129,0.));
#9080=CARTESIAN_POINT('Ctrl Pts',(10.9733873885115,-17.4330106728622,0.));
#9081=CARTESIAN_POINT('Ctrl Pts',(11.0151614525642,-17.460636011184,0.));
#9082=CARTESIAN_POINT('Ctrl Pts',(11.0571618040371,-17.4880571878157,0.));
#9083=CARTESIAN_POINT('Ctrl Pts',(11.0993856581394,-17.5152751467292,0.));
#9084=CARTESIAN_POINT('Ctrl Pts',(11.1418300507683,-17.5422909714139,0.));
#9085=CARTESIAN_POINT('Ctrl Pts',(11.1844919535058,-17.5691058058227,0.));
#9086=CARTESIAN_POINT('Ctrl Pts',(11.2273684103051,-17.5957207597803,0.));
#9087=CARTESIAN_POINT('Ctrl Pts',(11.2704566868205,-17.6221368072528,0.));
#9088=CARTESIAN_POINT('Ctrl Pts',(11.3137543310722,-17.6483547422688,0.));
#9089=CARTESIAN_POINT('Ctrl Pts',(11.3572590796967,-17.674375235974,0.));
#9090=CARTESIAN_POINT('Ctrl Pts',(11.4009687970126,-17.700198872213,0.));
#9091=CARTESIAN_POINT('Ctrl Pts',(11.4448814046804,-17.725826190457,0.));
#9092=CARTESIAN_POINT('Ctrl Pts',(11.4889948016216,-17.7512577332768,0.));
#9093=CARTESIAN_POINT('Ctrl Pts',(11.5333068279911,-17.7764940721306,0.));
#9094=CARTESIAN_POINT('Ctrl Pts',(11.5778153222435,-17.8015357852426,0.));
#9095=CARTESIAN_POINT('Ctrl Pts',(11.6225181583564,-17.8263834470057,0.));
#9096=CARTESIAN_POINT('Ctrl Pts',(11.6674132861792,-17.8510376144926,0.));
#9097=CARTESIAN_POINT('Ctrl Pts',(11.7124987772363,-17.8754988158862,0.));
#9098=CARTESIAN_POINT('Ctrl Pts',(11.7577728408871,-17.8997675418752,0.));
#9099=CARTESIAN_POINT('Ctrl Pts',(11.8032337607271,-17.9238442458356,0.));
#9100=CARTESIAN_POINT('Ctrl Pts',(11.8488798430201,-17.9477293432951,0.));
#9101=CARTESIAN_POINT('Ctrl Pts',(11.8947093631895,-17.9714232133203,0.));
#9102=CARTESIAN_POINT('Ctrl Pts',(11.9407205019619,-17.9949261997754,0.));
#9103=CARTESIAN_POINT('Ctrl Pts',(11.986911314246,-18.0182386160553,0.));
#9104=CARTESIAN_POINT('Ctrl Pts',(12.0332798395991,-18.0413607600052,0.));
#9105=CARTESIAN_POINT('Ctrl Pts',(12.0798241915081,-18.0642929289333,0.));
#9106=CARTESIAN_POINT('Ctrl Pts',(12.1265426519718,-18.0870354350128,0.));
#9107=CARTESIAN_POINT('Ctrl Pts',(12.1734337668195,-18.109588624154,0.));
#9108=CARTESIAN_POINT('Ctrl Pts',(12.2299089600472,-18.1364257412858,0.));
#9109=CARTESIAN_POINT('Ctrl Pts',(12.2771850498068,-18.1585543320743,0.));
#9110=CARTESIAN_POINT('Ctrl Pts',(12.3151419520839,-18.1761067306718,0.));
#9111=CARTESIAN_POINT('Ctrl Pts',(12.3436860694314,-18.1891864723772,0.));
#9112=CARTESIAN_POINT('Ctrl Pts',(12.3627494547115,-18.1978687191668,0.));
#9113=CARTESIAN_POINT('Ctrl Pts',(9.57984538049454,-16.1689656784104,13.));
#9114=CARTESIAN_POINT('Ctrl Pts',(9.58794311444024,-16.1826331205288,13.));
#9115=CARTESIAN_POINT('Ctrl Pts',(9.59639855902139,-16.196060540494,13.));
#9116=CARTESIAN_POINT('Ctrl Pts',(9.60518801710191,-16.2092641655575,13.));
#9117=CARTESIAN_POINT('Ctrl Pts',(9.61548991937318,-16.2247398016872,13.));
#9118=CARTESIAN_POINT('Ctrl Pts',(9.62624998105864,-16.2399084848403,13.));
#9119=CARTESIAN_POINT('Ctrl Pts',(9.63737105567212,-16.2548366371546,13.));
#9120=CARTESIAN_POINT('Ctrl Pts',(9.65301893987961,-16.2758412618842,13.));
#9121=CARTESIAN_POINT('Ctrl Pts',(9.66937567449445,-16.296373798593,13.));
#9122=CARTESIAN_POINT('Ctrl Pts',(9.6861023820138,-16.3166650331525,13.));
#9123=CARTESIAN_POINT('Ctrl Pts',(9.69722828051143,-16.3301619042994,13.));
#9124=CARTESIAN_POINT('Ctrl Pts',(9.70851618070908,-16.343553146753,13.));
#9125=CARTESIAN_POINT('Ctrl Pts',(9.71989107792203,-16.3568892752803,13.));
#9126=CARTESIAN_POINT('Ctrl Pts',(9.73186502185141,-16.3709277366598,13.));
#9127=CARTESIAN_POINT('Ctrl Pts',(9.74393463777169,-16.3849056240606,13.));
#9128=CARTESIAN_POINT('Ctrl Pts',(9.75606525514033,-16.3988451548263,13.));
#9129=CARTESIAN_POINT('Ctrl Pts',(9.76953696976191,-16.4143257667958,13.));
#9130=CARTESIAN_POINT('Ctrl Pts',(9.78308498747857,-16.4297583183374,13.));
#9131=CARTESIAN_POINT('Ctrl Pts',(9.79671869020116,-16.445133876345,13.));
#9132=CARTESIAN_POINT('Ctrl Pts',(9.81727215878356,-16.4683132763127,13.));
#9133=CARTESIAN_POINT('Ctrl Pts',(9.83802550134714,-16.4913594464763,13.));
#9134=CARTESIAN_POINT('Ctrl Pts',(9.85910360865385,-16.5141788054386,13.));
#9135=CARTESIAN_POINT('Ctrl Pts',(9.87441639279619,-16.530756570841,13.));
#9136=CARTESIAN_POINT('Ctrl Pts',(9.88990330206655,-16.5472127771021,13.));
#9137=CARTESIAN_POINT('Ctrl Pts',(9.90558047214739,-16.5635345032248,13.));
#9138=CARTESIAN_POINT('Ctrl Pts',(9.92474447016412,-16.5834864158106,13.));
#9139=CARTESIAN_POINT('Ctrl Pts',(9.94419173110064,-16.6032381063723,13.));
#9140=CARTESIAN_POINT('Ctrl Pts',(9.96388214930523,-16.6228156007794,13.));
#9141=CARTESIAN_POINT('Ctrl Pts',(9.98515106890727,-16.6439625439386,13.));
#9142=CARTESIAN_POINT('Ctrl Pts',(10.0066988150519,-16.664909699818,13.));
#9143=CARTESIAN_POINT('Ctrl Pts',(10.0284493480894,-16.6857083247985,13.));
#9144=CARTESIAN_POINT('Ctrl Pts',(10.0485293380065,-16.7049095176695,13.));
#9145=CARTESIAN_POINT('Ctrl Pts',(10.0687801145839,-16.7239855768671,13.));
#9146=CARTESIAN_POINT('Ctrl Pts',(10.089177591015,-16.7429517500618,13.));
#9147=CARTESIAN_POINT('Ctrl Pts',(10.1168886100199,-16.7687182701321,13.));
#9148=CARTESIAN_POINT('Ctrl Pts',(10.1448719871897,-16.7942808297091,13.));
#9149=CARTESIAN_POINT('Ctrl Pts',(10.1731502199795,-16.819619458001,13.));
#9150=CARTESIAN_POINT('Ctrl Pts',(10.2004381038856,-16.8440706870545,13.));
#9151=CARTESIAN_POINT('Ctrl Pts',(10.228006930926,-16.868308889081,13.));
#9152=CARTESIAN_POINT('Ctrl Pts',(10.2558682820648,-16.8923226175308,13.));
#9153=CARTESIAN_POINT('Ctrl Pts',(10.2937187080095,-16.9249459402769,13.));
#9154=CARTESIAN_POINT('Ctrl Pts',(10.3321063567311,-16.9571568355792,13.));
#9155=CARTESIAN_POINT('Ctrl Pts',(10.3709578723438,-16.9889999234809,13.));
#9156=CARTESIAN_POINT('Ctrl Pts',(10.4051075099835,-17.0169893055171,13.));
#9157=CARTESIAN_POINT('Ctrl Pts',(10.4396099588442,-17.0446984862637,13.));
#9158=CARTESIAN_POINT('Ctrl Pts',(10.4744368761282,-17.0721430001052,13.));
#9159=CARTESIAN_POINT('Ctrl Pts',(10.5257802080853,-17.1126028769606,13.));
#9160=CARTESIAN_POINT('Ctrl Pts',(10.577836103537,-17.1524822679612,13.));
#9161=CARTESIAN_POINT('Ctrl Pts',(10.630594631353,-17.1917748564007,13.));
#9162=CARTESIAN_POINT('Ctrl Pts',(10.6971764079367,-17.2413624861769,13.));
#9163=CARTESIAN_POINT('Ctrl Pts',(10.764872979571,-17.2900185096906,13.));
#9164=CARTESIAN_POINT('Ctrl Pts',(10.8335716331614,-17.3377983049103,13.));
#9165=CARTESIAN_POINT('Ctrl Pts',(10.9266292560921,-17.402519721341,13.));
#9166=CARTESIAN_POINT('Ctrl Pts',(11.0215303650587,-17.4656299469596,13.));
#9167=CARTESIAN_POINT('Ctrl Pts',(11.1181400566921,-17.5271690591565,13.));
#9168=CARTESIAN_POINT('Ctrl Pts',(11.2042701269916,-17.5820327893897,13.));
#9169=CARTESIAN_POINT('Ctrl Pts',(11.291751266876,-17.6356526672064,13.));
#9170=CARTESIAN_POINT('Ctrl Pts',(11.3804891404118,-17.6880597480309,13.));
#9171=CARTESIAN_POINT('Ctrl Pts',(11.5062551088123,-17.76233499273,13.));
#9172=CARTESIAN_POINT('Ctrl Pts',(11.6345494491014,-17.8341701544337,13.));
#9173=CARTESIAN_POINT('Ctrl Pts',(11.765154236571,-17.9036238130503,13.));
#9174=CARTESIAN_POINT('Ctrl Pts',(11.8666049274963,-17.9575737622862,13.));
#9175=CARTESIAN_POINT('Ctrl Pts',(11.9694546928344,-18.0100864753188,13.));
#9176=CARTESIAN_POINT('Ctrl Pts',(12.073610189358,-18.0611784506835,13.));
#9177=CARTESIAN_POINT('Ctrl Pts',(12.1637125549315,-18.1053768655136,13.));
#9178=CARTESIAN_POINT('Ctrl Pts',(12.2547877907941,-18.1485120961321,13.));
#9179=CARTESIAN_POINT('Ctrl Pts',(12.3468112467815,-18.1905949543846,13.));
#9180=CARTESIAN_POINT('Ctrl Pts',(12.3521208125291,-18.1930230494864,13.));
#9181=CARTESIAN_POINT('Ctrl Pts',(12.357433548566,-18.1954476376835,13.));
#9182=CARTESIAN_POINT('Ctrl Pts',(12.3627494547115,-18.1978687191668,13.));
#9183=CARTESIAN_POINT('Ctrl Pts',(7.455743247944,-20.698113262342,0.));
#9184=CARTESIAN_POINT('Ctrl Pts',(7.455743247944,-20.698113262342,21.));
#9185=CARTESIAN_POINT('Ctrl Pts',(7.45783379370107,-20.6878503127065,0.));
#9186=CARTESIAN_POINT('Ctrl Pts',(7.45783379370107,-20.6878503127065,21.));
#9187=CARTESIAN_POINT('Ctrl Pts',(7.46198969876653,-20.6673271112931,0.));
#9188=CARTESIAN_POINT('Ctrl Pts',(7.46198969876653,-20.6673271112931,21.));
#9189=CARTESIAN_POINT('Ctrl Pts',(7.46814799701905,-20.6365504027501,0.));
#9190=CARTESIAN_POINT('Ctrl Pts',(7.46814799701905,-20.6365504027501,21.));
#9191=CARTESIAN_POINT('Ctrl Pts',(7.47620789245427,-20.5955309838521,0.));
#9192=CARTESIAN_POINT('Ctrl Pts',(7.47620789245427,-20.5955309838521,21.));
#9193=CARTESIAN_POINT('Ctrl Pts',(7.48603045196744,-20.5442837929044,0.));
#9194=CARTESIAN_POINT('Ctrl Pts',(7.48603045196744,-20.5442837929044,21.));
#9195=CARTESIAN_POINT('Ctrl Pts',(7.49560012018405,-20.4930639156161,0.));
#9196=CARTESIAN_POINT('Ctrl Pts',(7.49560012018405,-20.4930639156161,21.));
#9197=CARTESIAN_POINT('Ctrl Pts',(7.50491611266253,-20.4418717748497,0.));
#9198=CARTESIAN_POINT('Ctrl Pts',(7.50491611266253,-20.4418717748497,21.));
#9199=CARTESIAN_POINT('Ctrl Pts',(7.51397746081993,-20.3907080367098,0.));
#9200=CARTESIAN_POINT('Ctrl Pts',(7.51397746081993,-20.3907080367098,21.));
#9201=CARTESIAN_POINT('Ctrl Pts',(7.52278303006887,-20.3395736743243,0.));
#9202=CARTESIAN_POINT('Ctrl Pts',(7.52278303006887,-20.3395736743243,21.));
#9203=CARTESIAN_POINT('Ctrl Pts',(7.53133155804007,-20.2884698940944,0.));
#9204=CARTESIAN_POINT('Ctrl Pts',(7.53133155804007,-20.2884698940944,21.));
#9205=CARTESIAN_POINT('Ctrl Pts',(7.53962169534166,-20.2373980474879,0.));
#9206=CARTESIAN_POINT('Ctrl Pts',(7.53962169534166,-20.2373980474879,21.));
#9207=CARTESIAN_POINT('Ctrl Pts',(7.54765204869254,-20.1863595454674,0.));
#9208=CARTESIAN_POINT('Ctrl Pts',(7.54765204869254,-20.1863595454674,21.));
#9209=CARTESIAN_POINT('Ctrl Pts',(7.55542122125494,-20.1353557774357,0.));
#9210=CARTESIAN_POINT('Ctrl Pts',(7.55542122125494,-20.1353557774357,21.));
#9211=CARTESIAN_POINT('Ctrl Pts',(7.5629278654946,-20.0843880130978,0.));
#9212=CARTESIAN_POINT('Ctrl Pts',(7.5629278654946,-20.0843880130978,21.));
#9213=CARTESIAN_POINT('Ctrl Pts',(7.57017066105972,-20.0334574248557,0.));
#9214=CARTESIAN_POINT('Ctrl Pts',(7.57017066105972,-20.0334574248557,21.));
#9215=CARTESIAN_POINT('Ctrl Pts',(7.57714827622805,-19.9825651387294,0.));
#9216=CARTESIAN_POINT('Ctrl Pts',(7.57714827622805,-19.9825651387294,21.));
#9217=CARTESIAN_POINT('Ctrl Pts',(7.58385933533351,-19.931712276832,0.));
#9218=CARTESIAN_POINT('Ctrl Pts',(7.58385933533351,-19.931712276832,21.));
#9219=CARTESIAN_POINT('Ctrl Pts',(7.59030238888851,-19.8808999994024,0.));
#9220=CARTESIAN_POINT('Ctrl Pts',(7.59030238888851,-19.8808999994024,21.));
#9221=CARTESIAN_POINT('Ctrl Pts',(7.59647587605448,-19.830129556152,0.));
#9222=CARTESIAN_POINT('Ctrl Pts',(7.59647587605448,-19.830129556152,21.));
#9223=CARTESIAN_POINT('Ctrl Pts',(7.60237814110186,-19.7794022782484,0.));
#9224=CARTESIAN_POINT('Ctrl Pts',(7.60237814110186,-19.7794022782484,21.));
#9225=CARTESIAN_POINT('Ctrl Pts',(7.60800746969261,-19.7287195480601,0.));
#9226=CARTESIAN_POINT('Ctrl Pts',(7.60800746969261,-19.7287195480601,21.));
#9227=CARTESIAN_POINT('Ctrl Pts',(7.61336212350878,-19.6780827744426,0.));
#9228=CARTESIAN_POINT('Ctrl Pts',(7.61336212350878,-19.6780827744426,21.));
#9229=CARTESIAN_POINT('Ctrl Pts',(7.6184403707059,-19.6274933688524,0.));
#9230=CARTESIAN_POINT('Ctrl Pts',(7.6184403707059,-19.6274933688524,21.));
#9231=CARTESIAN_POINT('Ctrl Pts',(7.62324053735219,-19.5769527121826,0.));
#9232=CARTESIAN_POINT('Ctrl Pts',(7.62324053735219,-19.5769527121826,21.));
#9233=CARTESIAN_POINT('Ctrl Pts',(7.62776096538882,-19.5264621687521,0.));
#9234=CARTESIAN_POINT('Ctrl Pts',(7.62776096538882,-19.5264621687521,21.));
#9235=CARTESIAN_POINT('Ctrl Pts',(7.63199992715365,-19.4760231231881,0.));
#9236=CARTESIAN_POINT('Ctrl Pts',(7.63199992715365,-19.4760231231881,21.));
#9237=CARTESIAN_POINT('Ctrl Pts',(7.63595554930653,-19.4256370121006,0.));
#9238=CARTESIAN_POINT('Ctrl Pts',(7.63595554930653,-19.4256370121006,21.));
#9239=CARTESIAN_POINT('Ctrl Pts',(7.6396257482276,-19.3753053524647,0.));
#9240=CARTESIAN_POINT('Ctrl Pts',(7.6396257482276,-19.3753053524647,21.));
#9241=CARTESIAN_POINT('Ctrl Pts',(7.64300812875338,-19.3250297839295,0.));
#9242=CARTESIAN_POINT('Ctrl Pts',(7.64300812875338,-19.3250297839295,21.));
#9243=CARTESIAN_POINT('Ctrl Pts',(7.64610005549613,-19.2748120456486,0.));
#9244=CARTESIAN_POINT('Ctrl Pts',(7.64610005549613,-19.2748120456486,21.));
#9245=CARTESIAN_POINT('Ctrl Pts',(7.64889882291923,-19.224653915265,0.));
#9246=CARTESIAN_POINT('Ctrl Pts',(7.64889882291923,-19.224653915265,21.));
#9247=CARTESIAN_POINT('Ctrl Pts',(7.65140181220525,-19.1745571539291,0.));
#9248=CARTESIAN_POINT('Ctrl Pts',(7.65140181220525,-19.1745571539291,21.));
#9249=CARTESIAN_POINT('Ctrl Pts',(7.65360662280608,-19.1245234597312,0.));
#9250=CARTESIAN_POINT('Ctrl Pts',(7.65360662280608,-19.1245234597312,21.));
#9251=CARTESIAN_POINT('Ctrl Pts',(7.65551129907201,-19.0745543888799,0.));
#9252=CARTESIAN_POINT('Ctrl Pts',(7.65551129907201,-19.0745543888799,21.));
#9253=CARTESIAN_POINT('Ctrl Pts',(7.65711415727854,-19.0246514144531,0.));
#9254=CARTESIAN_POINT('Ctrl Pts',(7.65711415727854,-19.0246514144531,21.));
#9255=CARTESIAN_POINT('Ctrl Pts',(7.65841335587266,-18.974816073814,0.));
#9256=CARTESIAN_POINT('Ctrl Pts',(7.65841335587266,-18.974816073814,21.));
#9257=CARTESIAN_POINT('Ctrl Pts',(7.65940650980098,-18.9250501008887,0.));
#9258=CARTESIAN_POINT('Ctrl Pts',(7.65940650980098,-18.9250501008887,21.));
#9259=CARTESIAN_POINT('Ctrl Pts',(7.66009036321662,-18.8753555389435,0.));
#9260=CARTESIAN_POINT('Ctrl Pts',(7.66009036321662,-18.8753555389435,21.));
#9261=CARTESIAN_POINT('Ctrl Pts',(7.66046025294774,-18.8257349246207,0.));
#9262=CARTESIAN_POINT('Ctrl Pts',(7.66046025294774,-18.8257349246207,21.));
#9263=CARTESIAN_POINT('Ctrl Pts',(7.6605104692254,-18.7761911671591,0.));
#9264=CARTESIAN_POINT('Ctrl Pts',(7.6605104692254,-18.7761911671591,21.));
#9265=CARTESIAN_POINT('Ctrl Pts',(7.66023521705904,-18.7267272235231,0.));
#9266=CARTESIAN_POINT('Ctrl Pts',(7.66023521705904,-18.7267272235231,21.));
#9267=CARTESIAN_POINT('Ctrl Pts',(7.65962948375621,-18.6773458057584,0.));
#9268=CARTESIAN_POINT('Ctrl Pts',(7.65962948375621,-18.6773458057584,21.));
#9269=CARTESIAN_POINT('Ctrl Pts',(7.65868976978871,-18.6280491346907,0.));
#9270=CARTESIAN_POINT('Ctrl Pts',(7.65868976978871,-18.6280491346907,21.));
#9271=CARTESIAN_POINT('Ctrl Pts',(7.65741532450727,-18.5788385228928,0.));
#9272=CARTESIAN_POINT('Ctrl Pts',(7.65741532450727,-18.5788385228928,21.));
#9273=CARTESIAN_POINT('Ctrl Pts',(7.65580722110436,-18.5297146894905,0.));
#9274=CARTESIAN_POINT('Ctrl Pts',(7.65580722110436,-18.5297146894905,21.));
#9275=CARTESIAN_POINT('Ctrl Pts',(7.65386603444742,-18.4806785483052,0.));
#9276=CARTESIAN_POINT('Ctrl Pts',(7.65386603444742,-18.4806785483052,21.));
#9277=CARTESIAN_POINT('Ctrl Pts',(7.65158974829126,-18.4317319183719,0.));
#9278=CARTESIAN_POINT('Ctrl Pts',(7.65158974829126,-18.4317319183719,21.));
#9279=CARTESIAN_POINT('Ctrl Pts',(7.6489719793775,-18.3828781275628,0.));
#9280=CARTESIAN_POINT('Ctrl Pts',(7.6489719793775,-18.3828781275628,21.));
#9281=CARTESIAN_POINT('Ctrl Pts',(7.64599903846601,-18.3341230095852,0.));
#9282=CARTESIAN_POINT('Ctrl Pts',(7.64599903846601,-18.3341230095852,21.));
#9283=CARTESIAN_POINT('Ctrl Pts',(7.64265220270759,-18.2854741391282,0.));
#9284=CARTESIAN_POINT('Ctrl Pts',(7.64265220270759,-18.2854741391282,21.));
#9285=CARTESIAN_POINT('Ctrl Pts',(7.63891299603826,-18.2369390502576,0.));
#9286=CARTESIAN_POINT('Ctrl Pts',(7.63891299603826,-18.2369390502576,21.));
#9287=CARTESIAN_POINT('Ctrl Pts',(7.63476798969016,-18.1885236169197,0.));
#9288=CARTESIAN_POINT('Ctrl Pts',(7.63476798969016,-18.1885236169197,21.));
#9289=CARTESIAN_POINT('Ctrl Pts',(7.63021285851761,-18.1402306858819,0.));
#9290=CARTESIAN_POINT('Ctrl Pts',(7.63021285851761,-18.1402306858819,21.));
#9291=CARTESIAN_POINT('Ctrl Pts',(7.62525915358073,-18.0920577897363,0.));
#9292=CARTESIAN_POINT('Ctrl Pts',(7.62525915358073,-18.0920577897363,21.));
#9293=CARTESIAN_POINT('Ctrl Pts',(7.61992799636653,-18.0439992897906,0.));
#9294=CARTESIAN_POINT('Ctrl Pts',(7.61992799636653,-18.0439992897906,21.));
#9295=CARTESIAN_POINT('Ctrl Pts',(7.61423755067037,-17.9960506269561,0.));
#9296=CARTESIAN_POINT('Ctrl Pts',(7.61423755067037,-17.9960506269561,21.));
#9297=CARTESIAN_POINT('Ctrl Pts',(7.60819152580111,-17.9482122228183,0.));
#9298=CARTESIAN_POINT('Ctrl Pts',(7.60819152580111,-17.9482122228183,21.));
#9299=CARTESIAN_POINT('Ctrl Pts',(7.60176928403058,-17.900492838997,0.));
#9300=CARTESIAN_POINT('Ctrl Pts',(7.60176928403058,-17.900492838997,21.));
#9301=CARTESIAN_POINT('Ctrl Pts',(7.59491004201955,-17.8529149331931,0.));
#9302=CARTESIAN_POINT('Ctrl Pts',(7.59491004201955,-17.8529149331931,21.));
#9303=CARTESIAN_POINT('Ctrl Pts',(7.58752955799498,-17.8055090348024,0.));
#9304=CARTESIAN_POINT('Ctrl Pts',(7.58752955799498,-17.8055090348024,21.));
#9305=CARTESIAN_POINT('Ctrl Pts',(7.57954834582803,-17.7583042294209,0.));
#9306=CARTESIAN_POINT('Ctrl Pts',(7.57954834582803,-17.7583042294209,21.));
#9307=CARTESIAN_POINT('Ctrl Pts',(7.57091795530423,-17.7113192869136,0.));
#9308=CARTESIAN_POINT('Ctrl Pts',(7.57091795530423,-17.7113192869136,21.));
#9309=CARTESIAN_POINT('Ctrl Pts',(7.56164400295862,-17.6645549117314,0.));
#9310=CARTESIAN_POINT('Ctrl Pts',(7.56164400295862,-17.6645549117314,21.));
#9311=CARTESIAN_POINT('Ctrl Pts',(7.55182125346563,-17.6179818599248,0.));
#9312=CARTESIAN_POINT('Ctrl Pts',(7.55182125346563,-17.6179818599248,21.));
#9313=CARTESIAN_POINT('Ctrl Pts',(7.54158441095317,-17.5715579419204,0.));
#9314=CARTESIAN_POINT('Ctrl Pts',(7.54158441095317,-17.5715579419204,21.));
#9315=CARTESIAN_POINT('Ctrl Pts',(7.53103903007863,-17.5252518287336,0.));
#9316=CARTESIAN_POINT('Ctrl Pts',(7.53103903007863,-17.5252518287336,21.));
#9317=CARTESIAN_POINT('Ctrl Pts',(7.52019696747328,-17.4790653226646,0.));
#9318=CARTESIAN_POINT('Ctrl Pts',(7.52019696747328,-17.4790653226646,21.));
#9319=CARTESIAN_POINT('Ctrl Pts',(7.50891486634214,-17.4330545448126,0.));
#9320=CARTESIAN_POINT('Ctrl Pts',(7.50891486634214,-17.4330545448126,21.));
#9321=CARTESIAN_POINT('Ctrl Pts',(7.4968177445175,-17.3873563447297,0.));
#9322=CARTESIAN_POINT('Ctrl Pts',(7.4968177445175,-17.3873563447297,21.));
#9323=CARTESIAN_POINT('Ctrl Pts',(7.48340100912745,-17.3421522689127,0.));
#9324=CARTESIAN_POINT('Ctrl Pts',(7.48340100912745,-17.3421522689127,21.));
#9325=CARTESIAN_POINT('Ctrl Pts',(7.47120323460919,-17.3065305096784,0.));
#9326=CARTESIAN_POINT('Ctrl Pts',(7.47120323460919,-17.3065305096784,21.));
#9327=CARTESIAN_POINT('Ctrl Pts',(7.4610504981825,-17.2801832097582,0.));
#9328=CARTESIAN_POINT('Ctrl Pts',(7.4610504981825,-17.2801832097582,21.));
#9329=CARTESIAN_POINT('Ctrl Pts',(7.45381253347182,-17.2627905583523,0.));
#9330=CARTESIAN_POINT('Ctrl Pts',(7.45381253347182,-17.2627905583523,21.));
#9331=CARTESIAN_POINT('Ctrl Pts',(7.45007618140238,-17.2541372868972,0.));
#9332=CARTESIAN_POINT('Ctrl Pts',(7.45007618140238,-17.2541372868972,21.));
#9333=CARTESIAN_POINT('',(7.45574324794406,-20.698113262342,0.));
#9334=CARTESIAN_POINT('Ctrl Pts',(7.45007618140238,-17.2541372868972,0.));
#9335=CARTESIAN_POINT('Ctrl Pts',(7.45381253347182,-17.2627905583523,0.));
#9336=CARTESIAN_POINT('Ctrl Pts',(7.4610504981825,-17.2801832097582,0.));
#9337=CARTESIAN_POINT('Ctrl Pts',(7.47120323460919,-17.3065305096784,0.));
#9338=CARTESIAN_POINT('Ctrl Pts',(7.48340100912745,-17.3421522689127,0.));
#9339=CARTESIAN_POINT('Ctrl Pts',(7.4968177445175,-17.3873563447297,0.));
#9340=CARTESIAN_POINT('Ctrl Pts',(7.50891486634214,-17.4330545448126,0.));
#9341=CARTESIAN_POINT('Ctrl Pts',(7.52019696747328,-17.4790653226646,0.));
#9342=CARTESIAN_POINT('Ctrl Pts',(7.53103903007863,-17.5252518287336,0.));
#9343=CARTESIAN_POINT('Ctrl Pts',(7.54158441095317,-17.5715579419204,0.));
#9344=CARTESIAN_POINT('Ctrl Pts',(7.55182125346563,-17.6179818599248,0.));
#9345=CARTESIAN_POINT('Ctrl Pts',(7.56164400295862,-17.6645549117314,0.));
#9346=CARTESIAN_POINT('Ctrl Pts',(7.57091795530423,-17.7113192869136,0.));
#9347=CARTESIAN_POINT('Ctrl Pts',(7.57954834582803,-17.7583042294209,0.));
#9348=CARTESIAN_POINT('Ctrl Pts',(7.58752955799498,-17.8055090348024,0.));
#9349=CARTESIAN_POINT('Ctrl Pts',(7.59491004201955,-17.8529149331931,0.));
#9350=CARTESIAN_POINT('Ctrl Pts',(7.60176928403058,-17.900492838997,0.));
#9351=CARTESIAN_POINT('Ctrl Pts',(7.60819152580111,-17.9482122228183,0.));
#9352=CARTESIAN_POINT('Ctrl Pts',(7.61423755067037,-17.9960506269561,0.));
#9353=CARTESIAN_POINT('Ctrl Pts',(7.61992799636653,-18.0439992897906,0.));
#9354=CARTESIAN_POINT('Ctrl Pts',(7.62525915358073,-18.0920577897363,0.));
#9355=CARTESIAN_POINT('Ctrl Pts',(7.63021285851761,-18.1402306858819,0.));
#9356=CARTESIAN_POINT('Ctrl Pts',(7.63476798969016,-18.1885236169197,0.));
#9357=CARTESIAN_POINT('Ctrl Pts',(7.63891299603826,-18.2369390502576,0.));
#9358=CARTESIAN_POINT('Ctrl Pts',(7.64265220270759,-18.2854741391282,0.));
#9359=CARTESIAN_POINT('Ctrl Pts',(7.64599903846601,-18.3341230095852,0.));
#9360=CARTESIAN_POINT('Ctrl Pts',(7.6489719793775,-18.3828781275628,0.));
#9361=CARTESIAN_POINT('Ctrl Pts',(7.65158974829126,-18.4317319183719,0.));
#9362=CARTESIAN_POINT('Ctrl Pts',(7.65386603444742,-18.4806785483052,0.));
#9363=CARTESIAN_POINT('Ctrl Pts',(7.65580722110436,-18.5297146894905,0.));
#9364=CARTESIAN_POINT('Ctrl Pts',(7.65741532450727,-18.5788385228928,0.));
#9365=CARTESIAN_POINT('Ctrl Pts',(7.65868976978871,-18.6280491346907,0.));
#9366=CARTESIAN_POINT('Ctrl Pts',(7.65962948375621,-18.6773458057584,0.));
#9367=CARTESIAN_POINT('Ctrl Pts',(7.66023521705904,-18.7267272235231,0.));
#9368=CARTESIAN_POINT('Ctrl Pts',(7.6605104692254,-18.7761911671591,0.));
#9369=CARTESIAN_POINT('Ctrl Pts',(7.66046025294774,-18.8257349246207,0.));
#9370=CARTESIAN_POINT('Ctrl Pts',(7.66009036321662,-18.8753555389435,0.));
#9371=CARTESIAN_POINT('Ctrl Pts',(7.65940650980098,-18.9250501008887,0.));
#9372=CARTESIAN_POINT('Ctrl Pts',(7.65841335587266,-18.974816073814,0.));
#9373=CARTESIAN_POINT('Ctrl Pts',(7.65711415727854,-19.0246514144531,0.));
#9374=CARTESIAN_POINT('Ctrl Pts',(7.65551129907201,-19.0745543888799,0.));
#9375=CARTESIAN_POINT('Ctrl Pts',(7.65360662280608,-19.1245234597312,0.));
#9376=CARTESIAN_POINT('Ctrl Pts',(7.65140181220525,-19.1745571539291,0.));
#9377=CARTESIAN_POINT('Ctrl Pts',(7.64889882291923,-19.224653915265,0.));
#9378=CARTESIAN_POINT('Ctrl Pts',(7.64610005549613,-19.2748120456486,0.));
#9379=CARTESIAN_POINT('Ctrl Pts',(7.64300812875338,-19.3250297839295,0.));
#9380=CARTESIAN_POINT('Ctrl Pts',(7.6396257482276,-19.3753053524647,0.));
#9381=CARTESIAN_POINT('Ctrl Pts',(7.63595554930653,-19.4256370121006,0.));
#9382=CARTESIAN_POINT('Ctrl Pts',(7.63199992715365,-19.4760231231881,0.));
#9383=CARTESIAN_POINT('Ctrl Pts',(7.62776096538882,-19.5264621687521,0.));
#9384=CARTESIAN_POINT('Ctrl Pts',(7.62324053735219,-19.5769527121826,0.));
#9385=CARTESIAN_POINT('Ctrl Pts',(7.6184403707059,-19.6274933688524,0.));
#9386=CARTESIAN_POINT('Ctrl Pts',(7.61336212350878,-19.6780827744426,0.));
#9387=CARTESIAN_POINT('Ctrl Pts',(7.60800746969261,-19.7287195480601,0.));
#9388=CARTESIAN_POINT('Ctrl Pts',(7.60237814110186,-19.7794022782484,0.));
#9389=CARTESIAN_POINT('Ctrl Pts',(7.59647587605448,-19.830129556152,0.));
#9390=CARTESIAN_POINT('Ctrl Pts',(7.59030238888851,-19.8808999994024,0.));
#9391=CARTESIAN_POINT('Ctrl Pts',(7.58385933533351,-19.931712276832,0.));
#9392=CARTESIAN_POINT('Ctrl Pts',(7.57714827622805,-19.9825651387294,0.));
#9393=CARTESIAN_POINT('Ctrl Pts',(7.57017066105972,-20.0334574248557,0.));
#9394=CARTESIAN_POINT('Ctrl Pts',(7.5629278654946,-20.0843880130978,0.));
#9395=CARTESIAN_POINT('Ctrl Pts',(7.55542122125494,-20.1353557774357,0.));
#9396=CARTESIAN_POINT('Ctrl Pts',(7.54765204869254,-20.1863595454674,0.));
#9397=CARTESIAN_POINT('Ctrl Pts',(7.53962169534166,-20.2373980474879,0.));
#9398=CARTESIAN_POINT('Ctrl Pts',(7.53133155804007,-20.2884698940944,0.));
#9399=CARTESIAN_POINT('Ctrl Pts',(7.52278303006887,-20.3395736743243,0.));
#9400=CARTESIAN_POINT('Ctrl Pts',(7.51397746081993,-20.3907080367098,0.));
#9401=CARTESIAN_POINT('Ctrl Pts',(7.50491611266253,-20.4418717748497,0.));
#9402=CARTESIAN_POINT('Ctrl Pts',(7.49560012018405,-20.4930639156161,0.));
#9403=CARTESIAN_POINT('Ctrl Pts',(7.48411651832412,-20.5545277683621,0.));
#9404=CARTESIAN_POINT('Ctrl Pts',(7.47423073598681,-20.6057817877246,0.));
#9405=CARTESIAN_POINT('Ctrl Pts',(7.46612041736313,-20.6468066077586,0.));
#9406=CARTESIAN_POINT('Ctrl Pts',(7.45992433946823,-20.6775873630604,0.));
#9407=CARTESIAN_POINT('Ctrl Pts',(7.455743247944,-20.698113262342,0.));
#9408=CARTESIAN_POINT('',(7.45574324794406,-20.698113262342,13.));
#9409=CARTESIAN_POINT('Ctrl Pts',(7.455743247944,-20.698113262342,13.));
#9410=CARTESIAN_POINT('Ctrl Pts',(7.47632490106067,-20.5970733933809,13.));
#9411=CARTESIAN_POINT('Ctrl Pts',(7.49544541955086,-20.496187784905,13.));
#9412=CARTESIAN_POINT('Ctrl Pts',(7.51308219823822,-20.3954689842507,13.));
#9413=CARTESIAN_POINT('Ctrl Pts',(7.54230710648616,-20.2285735573624,13.));
#9414=CARTESIAN_POINT('Ctrl Pts',(7.56745095675757,-20.0621477318166,13.));
#9415=CARTESIAN_POINT('Ctrl Pts',(7.58830059897784,-19.8963869129096,13.));
#9416=CARTESIAN_POINT('Ctrl Pts',(7.60432685672297,-19.7689734263959,13.));
#9417=CARTESIAN_POINT('Ctrl Pts',(7.6178148542035,-19.6419503944581,13.));
#9418=CARTESIAN_POINT('Ctrl Pts',(7.62864367929131,-19.5154161645489,13.));
#9419=CARTESIAN_POINT('Ctrl Pts',(7.64030064883062,-19.3792051119398,13.));
#9420=CARTESIAN_POINT('Ctrl Pts',(7.64888186436128,-19.2435576445087,13.));
#9421=CARTESIAN_POINT('Ctrl Pts',(7.65417053742034,-19.1086228836098,13.));
#9422=CARTESIAN_POINT('Ctrl Pts',(7.6570984904104,-19.0339193365717,13.));
#9423=CARTESIAN_POINT('Ctrl Pts',(7.65902218171088,-18.9594327324131,13.));
#9424=CARTESIAN_POINT('Ctrl Pts',(7.65990167998048,-18.8851905418284,13.));
#9425=CARTESIAN_POINT('Ctrl Pts',(7.66074919903795,-18.8136478525884,13.));
#9426=CARTESIAN_POINT('Ctrl Pts',(7.66062065572298,-18.7423342828967,13.));
#9427=CARTESIAN_POINT('Ctrl Pts',(7.65944821270055,-18.6712863090049,13.));
#9428=CARTESIAN_POINT('Ctrl Pts',(7.65843486239164,-18.6098790722244,13.));
#9429=CARTESIAN_POINT('Ctrl Pts',(7.65664478982407,-18.5486691991956,13.));
#9430=CARTESIAN_POINT('Ctrl Pts',(7.65407864069922,-18.4876659849921,13.));
#9431=CARTESIAN_POINT('Ctrl Pts',(7.6522370315769,-18.4438867382289,13.));
#9432=CARTESIAN_POINT('Ctrl Pts',(7.64999840197462,-18.4002130327578,13.));
#9433=CARTESIAN_POINT('Ctrl Pts',(7.6473265656267,-18.3566609384042,13.));
#9434=CARTESIAN_POINT('Ctrl Pts',(7.6446982368131,-18.3138180357798,13.));
#9435=CARTESIAN_POINT('Ctrl Pts',(7.64164464439788,-18.2710948572858,13.));
#9436=CARTESIAN_POINT('Ctrl Pts',(7.63811742043929,-18.2285117407612,13.));
#9437=CARTESIAN_POINT('Ctrl Pts',(7.63505911004306,-18.1915896769798,13.));
#9438=CARTESIAN_POINT('Ctrl Pts',(7.63164238136018,-18.1547737064202,13.));
#9439=CARTESIAN_POINT('Ctrl Pts',(7.62788266165966,-18.1180614604294,13.));
#9440=CARTESIAN_POINT('Ctrl Pts',(7.62447721821563,-18.0848085885711,13.));
#9441=CARTESIAN_POINT('Ctrl Pts',(7.62079564900185,-18.0516390296195,13.));
#9442=CARTESIAN_POINT('Ctrl Pts',(7.61686093607235,-18.0185473584385,13.));
#9443=CARTESIAN_POINT('Ctrl Pts',(7.613546541745,-17.9906726826464,13.));
#9444=CARTESIAN_POINT('Ctrl Pts',(7.61005417561771,-17.9628527173707,13.));
#9445=CARTESIAN_POINT('Ctrl Pts',(7.60636550500381,-17.9350952312728,13.));
#9446=CARTESIAN_POINT('Ctrl Pts',(7.60102759729104,-17.8949271288214,13.));
#9447=CARTESIAN_POINT('Ctrl Pts',(7.59527782596877,-17.8548900767427,13.));
#9448=CARTESIAN_POINT('Ctrl Pts',(7.58891067826389,-17.8150590779995,13.));
#9449=CARTESIAN_POINT('Ctrl Pts',(7.58506340059934,-17.7909916432666,13.));
#9450=CARTESIAN_POINT('Ctrl Pts',(7.58098742040086,-17.7670005718324,13.));
#9451=CARTESIAN_POINT('Ctrl Pts',(7.57665817621866,-17.7430955913955,13.));
#9452=CARTESIAN_POINT('Ctrl Pts',(7.57266539519107,-17.7210484745465,13.));
#9453=CARTESIAN_POINT('Ctrl Pts',(7.56845593268894,-17.6990750119179,13.));
#9454=CARTESIAN_POINT('Ctrl Pts',(7.5640539035508,-17.677168309485,13.));
#9455=CARTESIAN_POINT('Ctrl Pts',(7.55799846635133,-17.6470334201721,13.));
#9456=CARTESIAN_POINT('Ctrl Pts',(7.55158552707213,-17.6170224065982,13.));
#9457=CARTESIAN_POINT('Ctrl Pts',(7.54495919885622,-17.5870909089353,13.));
#9458=CARTESIAN_POINT('Ctrl Pts',(7.54075533803913,-17.5681018329159,13.));
#9459=CARTESIAN_POINT('Ctrl Pts',(7.53646718585673,-17.5491442490901,13.));
#9460=CARTESIAN_POINT('Ctrl Pts',(7.53210330803199,-17.5302169633181,13.));
#9461=CARTESIAN_POINT('Ctrl Pts',(7.52818693080402,-17.5132306053213,13.));
#9462=CARTESIAN_POINT('Ctrl Pts',(7.52421025221346,-17.4962684160965,13.));
#9463=CARTESIAN_POINT('Ctrl Pts',(7.5201410653043,-17.4793429835169,13.));
#9464=CARTESIAN_POINT('Ctrl Pts',(7.51586353943418,-17.4615509829677,13.));
#9465=CARTESIAN_POINT('Ctrl Pts',(7.51148394209619,-17.4437995539328,13.));
#9466=CARTESIAN_POINT('Ctrl Pts',(7.506906015607,-17.4261238143115,13.));
#9467=CARTESIAN_POINT('Ctrl Pts',(7.49930208984073,-17.3967644499221,13.));
#9468=CARTESIAN_POINT('Ctrl Pts',(7.49114308213723,-17.3676168188804,13.));
#9469=CARTESIAN_POINT('Ctrl Pts',(7.48183975621879,-17.3388922514903,13.));
#9470=CARTESIAN_POINT('Ctrl Pts',(7.47670957121225,-17.3230525027557,13.));
#9471=CARTESIAN_POINT('Ctrl Pts',(7.47123011545282,-17.3073418194655,13.));
#9472=CARTESIAN_POINT('Ctrl Pts',(7.46532888198223,-17.2917860605788,13.));
#9473=CARTESIAN_POINT('Ctrl Pts',(7.46052853291189,-17.2791322530176,13.));
#9474=CARTESIAN_POINT('Ctrl Pts',(7.45544915949247,-17.2665809316801,13.));
#9475=CARTESIAN_POINT('Ctrl Pts',(7.45007618140238,-17.2541372868972,13.));
#9476=CARTESIAN_POINT('',(7.45574324794406,-20.698113262342,0.));
#9477=CARTESIAN_POINT('Origin',(1.75106900012182E-12,-5.38923623413286E-12,
0.));
#9478=CARTESIAN_POINT('',(6.1342227326009,-21.1275013067528,0.));
#9479=CARTESIAN_POINT('Origin',(1.75106900012182E-12,-5.38923623413286E-12,
0.));
#9480=CARTESIAN_POINT('',(6.1342227326009,-21.1275013067528,13.));
#9481=CARTESIAN_POINT('Origin',(1.75106900012182E-12,-5.38923623413286E-12,
13.));
#9482=CARTESIAN_POINT('',(6.1342227326009,-21.1275013067528,0.));
#9483=CARTESIAN_POINT('Ctrl Pts',(4.1144891981253,-18.337935196262,0.));
#9484=CARTESIAN_POINT('Ctrl Pts',(4.1144891981253,-18.337935196262,21.));
#9485=CARTESIAN_POINT('Ctrl Pts',(4.11655269114951,-18.3471320125699,0.));
#9486=CARTESIAN_POINT('Ctrl Pts',(4.11655269114951,-18.3471320125699,21.));
#9487=CARTESIAN_POINT('Ctrl Pts',(4.12092019868859,-18.3654573320481,0.));
#9488=CARTESIAN_POINT('Ctrl Pts',(4.12092019868859,-18.3654573320481,21.));
#9489=CARTESIAN_POINT('Ctrl Pts',(4.12819301671078,-18.3927403741815,0.));
#9490=CARTESIAN_POINT('Ctrl Pts',(4.12819301671078,-18.3927403741815,21.));
#9491=CARTESIAN_POINT('Ctrl Pts',(4.13926275457062,-18.4287286547442,0.));
#9492=CARTESIAN_POINT('Ctrl Pts',(4.13926275457062,-18.4287286547442,21.));
#9493=CARTESIAN_POINT('Ctrl Pts',(4.15497867673974,-18.4731856794913,0.));
#9494=CARTESIAN_POINT('Ctrl Pts',(4.15497867673974,-18.4731856794913,21.));
#9495=CARTESIAN_POINT('Ctrl Pts',(4.17205262766561,-18.5172668097744,0.));
#9496=CARTESIAN_POINT('Ctrl Pts',(4.17205262766561,-18.5172668097744,21.));
#9497=CARTESIAN_POINT('Ctrl Pts',(4.1899696727862,-18.5611217636409,0.));
#9498=CARTESIAN_POINT('Ctrl Pts',(4.1899696727862,-18.5611217636409,21.));
#9499=CARTESIAN_POINT('Ctrl Pts',(4.20834600700664,-18.6048602364653,0.));
#9500=CARTESIAN_POINT('Ctrl Pts',(4.20834600700664,-18.6048602364653,21.));
#9501=CARTESIAN_POINT('Ctrl Pts',(4.22703266508918,-18.6485210883348,0.));
#9502=CARTESIAN_POINT('Ctrl Pts',(4.22703266508918,-18.6485210883348,21.));
#9503=CARTESIAN_POINT('Ctrl Pts',(4.24603817988452,-18.6920958920047,0.));
#9504=CARTESIAN_POINT('Ctrl Pts',(4.24603817988452,-18.6920958920047,21.));
#9505=CARTESIAN_POINT('Ctrl Pts',(4.26546636161932,-18.735547949685,0.));
#9506=CARTESIAN_POINT('Ctrl Pts',(4.26546636161932,-18.735547949685,21.));
#9507=CARTESIAN_POINT('Ctrl Pts',(4.28545098663152,-18.778832216358,0.));
#9508=CARTESIAN_POINT('Ctrl Pts',(4.28545098663152,-18.778832216358,21.));
#9509=CARTESIAN_POINT('Ctrl Pts',(4.30608591031525,-18.8219166495975,0.));
#9510=CARTESIAN_POINT('Ctrl Pts',(4.30608591031525,-18.8219166495975,21.));
#9511=CARTESIAN_POINT('Ctrl Pts',(4.32737526247704,-18.8647973781745,0.));
#9512=CARTESIAN_POINT('Ctrl Pts',(4.32737526247704,-18.8647973781745,21.));
#9513=CARTESIAN_POINT('Ctrl Pts',(4.34926881342021,-18.9074876952706,0.));
#9514=CARTESIAN_POINT('Ctrl Pts',(4.34926881342021,-18.9074876952706,21.));
#9515=CARTESIAN_POINT('Ctrl Pts',(4.37168516143122,-18.9500107909187,0.));
#9516=CARTESIAN_POINT('Ctrl Pts',(4.37168516143122,-18.9500107909187,21.));
#9517=CARTESIAN_POINT('Ctrl Pts',(4.39453820875554,-18.9923914823906,0.));
#9518=CARTESIAN_POINT('Ctrl Pts',(4.39453820875554,-18.9923914823906,21.));
#9519=CARTESIAN_POINT('Ctrl Pts',(4.41776558033331,-19.034647328575,0.));
#9520=CARTESIAN_POINT('Ctrl Pts',(4.41776558033331,-19.034647328575,21.));
#9521=CARTESIAN_POINT('Ctrl Pts',(4.44134542994081,-19.0767833717249,0.));
#9522=CARTESIAN_POINT('Ctrl Pts',(4.44134542994081,-19.0767833717249,21.));
#9523=CARTESIAN_POINT('Ctrl Pts',(4.46528051067021,-19.1187970904933,0.));
#9524=CARTESIAN_POINT('Ctrl Pts',(4.46528051067021,-19.1187970904933,21.));
#9525=CARTESIAN_POINT('Ctrl Pts',(4.48958819710576,-19.1606814968494,0.));
#9526=CARTESIAN_POINT('Ctrl Pts',(4.48958819710576,-19.1606814968494,21.));
#9527=CARTESIAN_POINT('Ctrl Pts',(4.51428889122954,-19.2024287376926,0.));
#9528=CARTESIAN_POINT('Ctrl Pts',(4.51428889122954,-19.2024287376926,21.));
#9529=CARTESIAN_POINT('Ctrl Pts',(4.53939338835151,-19.2440340196551,0.));
#9530=CARTESIAN_POINT('Ctrl Pts',(4.53939338835151,-19.2440340196551,21.));
#9531=CARTESIAN_POINT('Ctrl Pts',(4.5648965160674,-19.2854975819105,0.));
#9532=CARTESIAN_POINT('Ctrl Pts',(4.5648965160674,-19.2854975819105,21.));
#9533=CARTESIAN_POINT('Ctrl Pts',(4.59078395765677,-19.3268225655679,0.));
#9534=CARTESIAN_POINT('Ctrl Pts',(4.59078395765677,-19.3268225655679,21.));
#9535=CARTESIAN_POINT('Ctrl Pts',(4.61703633725711,-19.3680137353983,0.));
#9536=CARTESIAN_POINT('Ctrl Pts',(4.61703633725711,-19.3680137353983,21.));
#9537=CARTESIAN_POINT('Ctrl Pts',(4.64363405547472,-19.4090759683639,0.));
#9538=CARTESIAN_POINT('Ctrl Pts',(4.64363405547472,-19.4090759683639,21.));
#9539=CARTESIAN_POINT('Ctrl Pts',(4.67056260851452,-19.4500125912299,0.));
#9540=CARTESIAN_POINT('Ctrl Pts',(4.67056260851452,-19.4500125912299,21.));
#9541=CARTESIAN_POINT('Ctrl Pts',(4.69781487613784,-19.4908246636763,0.));
#9542=CARTESIAN_POINT('Ctrl Pts',(4.69781487613784,-19.4908246636763,21.));
#9543=CARTESIAN_POINT('Ctrl Pts',(4.72538815796615,-19.531511899192,0.));
#9544=CARTESIAN_POINT('Ctrl Pts',(4.72538815796615,-19.531511899192,21.));
#9545=CARTESIAN_POINT('Ctrl Pts',(4.7532823819461,-19.5720732205813,0.));
#9546=CARTESIAN_POINT('Ctrl Pts',(4.7532823819461,-19.5720732205813,21.));
#9547=CARTESIAN_POINT('Ctrl Pts',(4.7814979936173,-19.6125074152527,0.));
#9548=CARTESIAN_POINT('Ctrl Pts',(4.7814979936173,-19.6125074152527,21.));
#9549=CARTESIAN_POINT('Ctrl Pts',(4.8100336141806,-19.6528138625329,0.));
#9550=CARTESIAN_POINT('Ctrl Pts',(4.8100336141806,-19.6528138625329,21.));
#9551=CARTESIAN_POINT('Ctrl Pts',(4.83888510708974,-19.6929928227072,0.));
#9552=CARTESIAN_POINT('Ctrl Pts',(4.83888510708974,-19.6929928227072,21.));
#9553=CARTESIAN_POINT('Ctrl Pts',(4.86804682289086,-19.7330450480715,0.));
#9554=CARTESIAN_POINT('Ctrl Pts',(4.86804682289086,-19.7330450480715,21.));
#9555=CARTESIAN_POINT('Ctrl Pts',(4.89751233527804,-19.772971552601,0.));
#9556=CARTESIAN_POINT('Ctrl Pts',(4.89751233527804,-19.772971552601,21.));
#9557=CARTESIAN_POINT('Ctrl Pts',(4.92727531494346,-19.8127733387903,0.));
#9558=CARTESIAN_POINT('Ctrl Pts',(4.92727531494346,-19.8127733387903,21.));
#9559=CARTESIAN_POINT('Ctrl Pts',(4.95733049830095,-19.8524510953961,0.));
#9560=CARTESIAN_POINT('Ctrl Pts',(4.95733049830095,-19.8524510953961,21.));
#9561=CARTESIAN_POINT('Ctrl Pts',(4.98767405031333,-19.8920050831202,0.));
#9562=CARTESIAN_POINT('Ctrl Pts',(4.98767405031333,-19.8920050831202,21.));
#9563=CARTESIAN_POINT('Ctrl Pts',(5.01830302225557,-19.931435301086,0.));
#9564=CARTESIAN_POINT('Ctrl Pts',(5.01830302225557,-19.931435301086,21.));
#9565=CARTESIAN_POINT('Ctrl Pts',(5.04921502064063,-19.9707415879783,0.));
#9566=CARTESIAN_POINT('Ctrl Pts',(5.04921502064063,-19.9707415879783,21.));
#9567=CARTESIAN_POINT('Ctrl Pts',(5.08040781745336,-20.0099237417205,0.));
#9568=CARTESIAN_POINT('Ctrl Pts',(5.08040781745336,-20.0099237417205,21.));
#9569=CARTESIAN_POINT('Ctrl Pts',(5.11187891582334,-20.0489816528155,0.));
#9570=CARTESIAN_POINT('Ctrl Pts',(5.11187891582334,-20.0489816528155,21.));
#9571=CARTESIAN_POINT('Ctrl Pts',(5.14362537555397,-20.087915358486,0.));
#9572=CARTESIAN_POINT('Ctrl Pts',(5.14362537555397,-20.087915358486,21.));
#9573=CARTESIAN_POINT('Ctrl Pts',(5.17564404279921,-20.1267249732337,0.));
#9574=CARTESIAN_POINT('Ctrl Pts',(5.17564404279921,-20.1267249732337,21.));
#9575=CARTESIAN_POINT('Ctrl Pts',(5.20793168386163,-20.1654106491899,0.));
#9576=CARTESIAN_POINT('Ctrl Pts',(5.20793168386163,-20.1654106491899,21.));
#9577=CARTESIAN_POINT('Ctrl Pts',(5.2404851444189,-20.2039725283917,0.));
#9578=CARTESIAN_POINT('Ctrl Pts',(5.2404851444189,-20.2039725283917,21.));
#9579=CARTESIAN_POINT('Ctrl Pts',(5.27330152298149,-20.2424106921768,0.));
#9580=CARTESIAN_POINT('Ctrl Pts',(5.27330152298149,-20.2424106921768,21.));
#9581=CARTESIAN_POINT('Ctrl Pts',(5.30637824220997,-20.2807251380077,0.));
#9582=CARTESIAN_POINT('Ctrl Pts',(5.30637824220997,-20.2807251380077,21.));
#9583=CARTESIAN_POINT('Ctrl Pts',(5.33971294212213,-20.3189158047642,0.));
#9584=CARTESIAN_POINT('Ctrl Pts',(5.33971294212213,-20.3189158047642,21.));
#9585=CARTESIAN_POINT('Ctrl Pts',(5.37330341114648,-20.3569825877537,0.));
#9586=CARTESIAN_POINT('Ctrl Pts',(5.37330341114648,-20.3569825877537,21.));
#9587=CARTESIAN_POINT('Ctrl Pts',(5.40714750595874,-20.3949253578015,0.));
#9588=CARTESIAN_POINT('Ctrl Pts',(5.40714750595874,-20.3949253578015,21.));
#9589=CARTESIAN_POINT('Ctrl Pts',(5.4412430606511,-20.4327439816542,0.));
#9590=CARTESIAN_POINT('Ctrl Pts',(5.4412430606511,-20.4327439816542,21.));
#9591=CARTESIAN_POINT('Ctrl Pts',(5.4755878444985,-20.4704383353718,0.));
#9592=CARTESIAN_POINT('Ctrl Pts',(5.4755878444985,-20.4704383353718,21.));
#9593=CARTESIAN_POINT('Ctrl Pts',(5.51017962306782,-20.5080083009242,0.));
#9594=CARTESIAN_POINT('Ctrl Pts',(5.51017962306782,-20.5080083009242,21.));
#9595=CARTESIAN_POINT('Ctrl Pts',(5.54501619689459,-20.5454537676144,0.));
#9596=CARTESIAN_POINT('Ctrl Pts',(5.54501619689459,-20.5454537676144,21.));
#9597=CARTESIAN_POINT('Ctrl Pts',(5.58009544402474,-20.5827746317185,0.));
#9598=CARTESIAN_POINT('Ctrl Pts',(5.58009544402474,-20.5827746317185,21.));
#9599=CARTESIAN_POINT('Ctrl Pts',(5.61541536715148,-20.6199707996366,0.));
#9600=CARTESIAN_POINT('Ctrl Pts',(5.61541536715148,-20.6199707996366,21.));
#9601=CARTESIAN_POINT('Ctrl Pts',(5.65097411164334,-20.6570421847033,0.));
#9602=CARTESIAN_POINT('Ctrl Pts',(5.65097411164334,-20.6570421847033,21.));
#9603=CARTESIAN_POINT('Ctrl Pts',(5.68676990500163,-20.6939886877061,0.));
#9604=CARTESIAN_POINT('Ctrl Pts',(5.68676990500163,-20.6939886877061,21.));
#9605=CARTESIAN_POINT('Ctrl Pts',(5.7228010079824,-20.7308101804425,0.));
#9606=CARTESIAN_POINT('Ctrl Pts',(5.7228010079824,-20.7308101804425,21.));
#9607=CARTESIAN_POINT('Ctrl Pts',(5.75906566327795,-20.7675064905026,0.));
#9608=CARTESIAN_POINT('Ctrl Pts',(5.75906566327795,-20.7675064905026,21.));
#9609=CARTESIAN_POINT('Ctrl Pts',(5.79556203439643,-20.8040773827343,0.));
#9610=CARTESIAN_POINT('Ctrl Pts',(5.79556203439643,-20.8040773827343,21.));
#9611=CARTESIAN_POINT('Ctrl Pts',(5.83228817460177,-20.8405225541277,0.));
#9612=CARTESIAN_POINT('Ctrl Pts',(5.83228817460177,-20.8405225541277,21.));
#9613=CARTESIAN_POINT('Ctrl Pts',(5.86924212736287,-20.8768416821402,0.));
#9614=CARTESIAN_POINT('Ctrl Pts',(5.86924212736287,-20.8768416821402,21.));
#9615=CARTESIAN_POINT('Ctrl Pts',(5.90642200662599,-20.9130344665641,0.));
#9616=CARTESIAN_POINT('Ctrl Pts',(5.90642200662599,-20.9130344665641,21.));
#9617=CARTESIAN_POINT('Ctrl Pts',(5.94382608200804,-20.9491006734021,0.));
#9618=CARTESIAN_POINT('Ctrl Pts',(5.94382608200804,-20.9491006734021,21.));
#9619=CARTESIAN_POINT('Ctrl Pts',(5.98145286361836,-20.9850401822713,0.));
#9620=CARTESIAN_POINT('Ctrl Pts',(5.98145286361836,-20.9850401822713,21.));
#9621=CARTESIAN_POINT('Ctrl Pts',(6.01930117633044,-21.0208530236003,0.));
#9622=CARTESIAN_POINT('Ctrl Pts',(6.01930117633044,-21.0208530236003,21.));
#9623=CARTESIAN_POINT('Ctrl Pts',(6.05737013696532,-21.0565393163693,0.));
#9624=CARTESIAN_POINT('Ctrl Pts',(6.05737013696532,-21.0565393163693,21.));
#9625=CARTESIAN_POINT('Ctrl Pts',(6.08800133883114,-21.0849872356853,0.));
#9626=CARTESIAN_POINT('Ctrl Pts',(6.08800133883114,-21.0849872356853,21.));
#9627=CARTESIAN_POINT('Ctrl Pts',(6.11107360216957,-21.1062663590356,0.));
#9628=CARTESIAN_POINT('Ctrl Pts',(6.11107360216957,-21.1062663590356,21.));
#9629=CARTESIAN_POINT('Ctrl Pts',(6.12649903511517,-21.1204271980506,0.));
#9630=CARTESIAN_POINT('Ctrl Pts',(6.12649903511517,-21.1204271980506,21.));
#9631=CARTESIAN_POINT('Ctrl Pts',(6.1342227326009,-21.1275013067528,0.));
#9632=CARTESIAN_POINT('Ctrl Pts',(6.1342227326009,-21.1275013067528,21.));
#9633=CARTESIAN_POINT('Ctrl Pts',(4.1144891981253,-18.337935196262,0.));
#9634=CARTESIAN_POINT('Ctrl Pts',(4.11655269114951,-18.3471320125699,0.));
#9635=CARTESIAN_POINT('Ctrl Pts',(4.12092019868859,-18.3654573320481,0.));
#9636=CARTESIAN_POINT('Ctrl Pts',(4.12819301671078,-18.3927403741815,0.));
#9637=CARTESIAN_POINT('Ctrl Pts',(4.13926275457062,-18.4287286547442,0.));
#9638=CARTESIAN_POINT('Ctrl Pts',(4.15497867673974,-18.4731856794913,0.));
#9639=CARTESIAN_POINT('Ctrl Pts',(4.17205262766561,-18.5172668097744,0.));
#9640=CARTESIAN_POINT('Ctrl Pts',(4.1899696727862,-18.5611217636409,0.));
#9641=CARTESIAN_POINT('Ctrl Pts',(4.20834600700664,-18.6048602364653,0.));
#9642=CARTESIAN_POINT('Ctrl Pts',(4.22703266508918,-18.6485210883348,0.));
#9643=CARTESIAN_POINT('Ctrl Pts',(4.24603817988452,-18.6920958920047,0.));
#9644=CARTESIAN_POINT('Ctrl Pts',(4.26546636161932,-18.735547949685,0.));
#9645=CARTESIAN_POINT('Ctrl Pts',(4.28545098663152,-18.778832216358,0.));
#9646=CARTESIAN_POINT('Ctrl Pts',(4.30608591031525,-18.8219166495975,0.));
#9647=CARTESIAN_POINT('Ctrl Pts',(4.32737526247704,-18.8647973781745,0.));
#9648=CARTESIAN_POINT('Ctrl Pts',(4.34926881342021,-18.9074876952706,0.));
#9649=CARTESIAN_POINT('Ctrl Pts',(4.37168516143122,-18.9500107909187,0.));
#9650=CARTESIAN_POINT('Ctrl Pts',(4.39453820875554,-18.9923914823906,0.));
#9651=CARTESIAN_POINT('Ctrl Pts',(4.41776558033331,-19.034647328575,0.));
#9652=CARTESIAN_POINT('Ctrl Pts',(4.44134542994081,-19.0767833717249,0.));
#9653=CARTESIAN_POINT('Ctrl Pts',(4.46528051067021,-19.1187970904933,0.));
#9654=CARTESIAN_POINT('Ctrl Pts',(4.48958819710576,-19.1606814968494,0.));
#9655=CARTESIAN_POINT('Ctrl Pts',(4.51428889122954,-19.2024287376926,0.));
#9656=CARTESIAN_POINT('Ctrl Pts',(4.53939338835151,-19.2440340196551,0.));
#9657=CARTESIAN_POINT('Ctrl Pts',(4.5648965160674,-19.2854975819105,0.));
#9658=CARTESIAN_POINT('Ctrl Pts',(4.59078395765677,-19.3268225655679,0.));
#9659=CARTESIAN_POINT('Ctrl Pts',(4.61703633725711,-19.3680137353983,0.));
#9660=CARTESIAN_POINT('Ctrl Pts',(4.64363405547472,-19.4090759683639,0.));
#9661=CARTESIAN_POINT('Ctrl Pts',(4.67056260851452,-19.4500125912299,0.));
#9662=CARTESIAN_POINT('Ctrl Pts',(4.69781487613784,-19.4908246636763,0.));
#9663=CARTESIAN_POINT('Ctrl Pts',(4.72538815796615,-19.531511899192,0.));
#9664=CARTESIAN_POINT('Ctrl Pts',(4.7532823819461,-19.5720732205813,0.));
#9665=CARTESIAN_POINT('Ctrl Pts',(4.7814979936173,-19.6125074152527,0.));
#9666=CARTESIAN_POINT('Ctrl Pts',(4.8100336141806,-19.6528138625329,0.));
#9667=CARTESIAN_POINT('Ctrl Pts',(4.83888510708974,-19.6929928227072,0.));
#9668=CARTESIAN_POINT('Ctrl Pts',(4.86804682289086,-19.7330450480715,0.));
#9669=CARTESIAN_POINT('Ctrl Pts',(4.89751233527804,-19.772971552601,0.));
#9670=CARTESIAN_POINT('Ctrl Pts',(4.92727531494346,-19.8127733387903,0.));
#9671=CARTESIAN_POINT('Ctrl Pts',(4.95733049830095,-19.8524510953961,0.));
#9672=CARTESIAN_POINT('Ctrl Pts',(4.98767405031333,-19.8920050831202,0.));
#9673=CARTESIAN_POINT('Ctrl Pts',(5.01830302225557,-19.931435301086,0.));
#9674=CARTESIAN_POINT('Ctrl Pts',(5.04921502064063,-19.9707415879783,0.));
#9675=CARTESIAN_POINT('Ctrl Pts',(5.08040781745336,-20.0099237417205,0.));
#9676=CARTESIAN_POINT('Ctrl Pts',(5.11187891582334,-20.0489816528155,0.));
#9677=CARTESIAN_POINT('Ctrl Pts',(5.14362537555397,-20.087915358486,0.));
#9678=CARTESIAN_POINT('Ctrl Pts',(5.17564404279921,-20.1267249732337,0.));
#9679=CARTESIAN_POINT('Ctrl Pts',(5.20793168386163,-20.1654106491899,0.));
#9680=CARTESIAN_POINT('Ctrl Pts',(5.2404851444189,-20.2039725283917,0.));
#9681=CARTESIAN_POINT('Ctrl Pts',(5.27330152298149,-20.2424106921768,0.));
#9682=CARTESIAN_POINT('Ctrl Pts',(5.30637824220997,-20.2807251380077,0.));
#9683=CARTESIAN_POINT('Ctrl Pts',(5.33971294212213,-20.3189158047642,0.));
#9684=CARTESIAN_POINT('Ctrl Pts',(5.37330341114648,-20.3569825877537,0.));
#9685=CARTESIAN_POINT('Ctrl Pts',(5.40714750595874,-20.3949253578015,0.));
#9686=CARTESIAN_POINT('Ctrl Pts',(5.4412430606511,-20.4327439816542,0.));
#9687=CARTESIAN_POINT('Ctrl Pts',(5.4755878444985,-20.4704383353718,0.));
#9688=CARTESIAN_POINT('Ctrl Pts',(5.51017962306782,-20.5080083009242,0.));
#9689=CARTESIAN_POINT('Ctrl Pts',(5.54501619689459,-20.5454537676144,0.));
#9690=CARTESIAN_POINT('Ctrl Pts',(5.58009544402474,-20.5827746317185,0.));
#9691=CARTESIAN_POINT('Ctrl Pts',(5.61541536715148,-20.6199707996366,0.));
#9692=CARTESIAN_POINT('Ctrl Pts',(5.65097411164334,-20.6570421847033,0.));
#9693=CARTESIAN_POINT('Ctrl Pts',(5.68676990500163,-20.6939886877061,0.));
#9694=CARTESIAN_POINT('Ctrl Pts',(5.7228010079824,-20.7308101804425,0.));
#9695=CARTESIAN_POINT('Ctrl Pts',(5.75906566327795,-20.7675064905026,0.));
#9696=CARTESIAN_POINT('Ctrl Pts',(5.79556203439643,-20.8040773827343,0.));
#9697=CARTESIAN_POINT('Ctrl Pts',(5.83228817460177,-20.8405225541277,0.));
#9698=CARTESIAN_POINT('Ctrl Pts',(5.86924212736287,-20.8768416821402,0.));
#9699=CARTESIAN_POINT('Ctrl Pts',(5.90642200662599,-20.9130344665641,0.));
#9700=CARTESIAN_POINT('Ctrl Pts',(5.94382608200804,-20.9491006734021,0.));
#9701=CARTESIAN_POINT('Ctrl Pts',(5.98145286361836,-20.9850401822713,0.));
#9702=CARTESIAN_POINT('Ctrl Pts',(6.02687083887286,-21.0280155918661,0.));
#9703=CARTESIAN_POINT('Ctrl Pts',(6.06499496148844,-21.0636702474951,0.));
#9704=CARTESIAN_POINT('Ctrl Pts',(6.09567013127871,-21.0920928984154,0.));
#9705=CARTESIAN_POINT('Ctrl Pts',(6.118775337615,-21.1133530893457,0.));
#9706=CARTESIAN_POINT('Ctrl Pts',(6.1342227326009,-21.1275013067528,0.));
#9707=CARTESIAN_POINT('Ctrl Pts',(4.1144891981253,-18.337935196262,13.));
#9708=CARTESIAN_POINT('Ctrl Pts',(4.11796712887951,-18.3534360435645,13.));
#9709=CARTESIAN_POINT('Ctrl Pts',(4.12185943358937,-18.3688191548995,13.));
#9710=CARTESIAN_POINT('Ctrl Pts',(4.12613856044267,-18.3840926404824,13.));
#9711=CARTESIAN_POINT('Ctrl Pts',(4.13115401716692,-18.4019943079477,13.));
#9712=CARTESIAN_POINT('Ctrl Pts',(4.13670006307401,-18.4197456248295,13.));
#9713=CARTESIAN_POINT('Ctrl Pts',(4.1426637807957,-18.4373797424196,13.));
#9714=CARTESIAN_POINT('Ctrl Pts',(4.15105501703309,-18.4621917897769,13.));
#9715=CARTESIAN_POINT('Ctrl Pts',(4.16026629328986,-18.4867739015683,13.));
#9716=CARTESIAN_POINT('Ctrl Pts',(4.16990400115282,-18.5112408492934,13.));
#9717=CARTESIAN_POINT('Ctrl Pts',(4.17631459686346,-18.5275152282609,13.));
#9718=CARTESIAN_POINT('Ctrl Pts',(4.18291190640786,-18.5437392096496,13.));
#9719=CARTESIAN_POINT('Ctrl Pts',(4.18960898617043,-18.5599376581358,13.));
#9720=CARTESIAN_POINT('Ctrl Pts',(4.19665876042785,-18.5769891804704,13.));
#9721=CARTESIAN_POINT('Ctrl Pts',(4.20381824254442,-18.5940126577989,13.));
#9722=CARTESIAN_POINT('Ctrl Pts',(4.21104759333806,-18.6110185062838,13.));
#9723=CARTESIAN_POINT('Ctrl Pts',(4.21907618313383,-18.6299044319376,13.));
#9724=CARTESIAN_POINT('Ctrl Pts',(4.22719219297436,-18.6487682283615,13.));
#9725=CARTESIAN_POINT('Ctrl Pts',(4.23540730606873,-18.6676042988365,13.));
#9726=CARTESIAN_POINT('Ctrl Pts',(4.24779198778708,-18.6960005893047,13.));
#9727=CARTESIAN_POINT('Ctrl Pts',(4.26040793123128,-18.7243319351566,13.));
#9728=CARTESIAN_POINT('Ctrl Pts',(4.27340283281643,-18.7525479285623,13.));
#9729=CARTESIAN_POINT('Ctrl Pts',(4.28284334471928,-18.7730462309044,13.));
#9730=CARTESIAN_POINT('Ctrl Pts',(4.29248702330027,-18.7934827312566,13.));
#9731=CARTESIAN_POINT('Ctrl Pts',(4.302353207313,-18.8138501272208,13.));
#9732=CARTESIAN_POINT('Ctrl Pts',(4.31441377244323,-18.8387475247599,13.));
#9733=CARTESIAN_POINT('Ctrl Pts',(4.32680560862706,-18.8635420328946,13.));
#9734=CARTESIAN_POINT('Ctrl Pts',(4.33948253068719,-18.8882460103694,13.));
#9735=CARTESIAN_POINT('Ctrl Pts',(4.35317571045417,-18.9149304060703,13.));
#9736=CARTESIAN_POINT('Ctrl Pts',(4.36719580768616,-18.9415109549169,13.));
#9737=CARTESIAN_POINT('Ctrl Pts',(4.38145466528598,-18.9680129070804,13.));
#9738=CARTESIAN_POINT('Ctrl Pts',(4.39461837564025,-18.9924793848231,13.));
#9739=CARTESIAN_POINT('Ctrl Pts',(4.40798318219245,-19.0168796293508,13.));
#9740=CARTESIAN_POINT('Ctrl Pts',(4.42152146523896,-19.0412206988271,13.));
#9741=CARTESIAN_POINT('Ctrl Pts',(4.43991391790099,-19.0742892915392,13.));
#9742=CARTESIAN_POINT('Ctrl Pts',(4.45862842583093,-19.1072480695959,13.));
#9743=CARTESIAN_POINT('Ctrl Pts',(4.47769255669439,-19.1400849917414,13.));
#9744=CARTESIAN_POINT('Ctrl Pts',(4.49608903122715,-19.1717719123942,13.));
#9745=CARTESIAN_POINT('Ctrl Pts',(4.51481852753143,-19.2033430485072,13.));
#9746=CARTESIAN_POINT('Ctrl Pts',(4.53389559693718,-19.2347910924796,13.));
#9747=CARTESIAN_POINT('Ctrl Pts',(4.55981233024546,-19.2775141413591,13.));
#9748=CARTESIAN_POINT('Ctrl Pts',(4.58636743987533,-19.3200109593949,13.));
#9749=CARTESIAN_POINT('Ctrl Pts',(4.61347737187984,-19.362301314555,13.));
#9750=CARTESIAN_POINT('Ctrl Pts',(4.63730641274119,-19.3994736173474,13.));
#9751=CARTESIAN_POINT('Ctrl Pts',(4.66155758397822,-19.4364884575386,13.));
#9752=CARTESIAN_POINT('Ctrl Pts',(4.68619912960012,-19.4733518508001,13.));
#9753=CARTESIAN_POINT('Ctrl Pts',(4.72252675031123,-19.527697442147,13.));
#9754=CARTESIAN_POINT('Ctrl Pts',(4.7597114391618,-19.5817111528721,13.));
#9755=CARTESIAN_POINT('Ctrl Pts',(4.79774570305514,-19.6353839065428,13.));
#9756=CARTESIAN_POINT('Ctrl Pts',(4.84574531526665,-19.7031194454701,13.));
#9757=CARTESIAN_POINT('Ctrl Pts',(4.89509304274286,-19.7703134648063,13.));
#9758=CARTESIAN_POINT('Ctrl Pts',(4.94566457622742,-19.8369838018677,13.));
#9759=CARTESIAN_POINT('Ctrl Pts',(5.01416761732255,-19.9272939136015,13.));
#9760=CARTESIAN_POINT('Ctrl Pts',(5.08492180316416,-20.0166413603291,13.));
#9761=CARTESIAN_POINT('Ctrl Pts',(5.15778644842965,-20.1050225704803,13.));
#9762=CARTESIAN_POINT('Ctrl Pts',(5.22274718796653,-20.1838167339825,13.));
#9763=CARTESIAN_POINT('Ctrl Pts',(5.28937724256698,-20.2618454270028,13.));
#9764=CARTESIAN_POINT('Ctrl Pts',(5.35757729677352,-20.3391090335982,13.));
#9765=CARTESIAN_POINT('Ctrl Pts',(5.45423552752918,-20.4486128104235,13.));
#9766=CARTESIAN_POINT('Ctrl Pts',(5.55405240994679,-20.5565772403027,13.));
#9767=CARTESIAN_POINT('Ctrl Pts',(5.65680258312696,-20.662990693601,13.));
#9768=CARTESIAN_POINT('Ctrl Pts',(5.73661648094275,-20.7456501405381,13.));
#9769=CARTESIAN_POINT('Ctrl Pts',(5.81820510837542,-20.8273750321949,13.));
#9770=CARTESIAN_POINT('Ctrl Pts',(5.90147459238375,-20.9081522149626,13.));
#9771=CARTESIAN_POINT('Ctrl Pts',(5.97350899070235,-20.9780305843057,13.));
#9772=CARTESIAN_POINT('Ctrl Pts',(6.04679718623577,-21.0471984384854,13.));
#9773=CARTESIAN_POINT('Ctrl Pts',(6.12131239423385,-21.1156584428611,13.));
#9774=CARTESIAN_POINT('Ctrl Pts',(6.12561174166735,-21.1196084196781,13.));
#9775=CARTESIAN_POINT('Ctrl Pts',(6.12991518786664,-21.1235560409334,13.));
#9776=CARTESIAN_POINT('Ctrl Pts',(6.1342227326009,-21.1275013067528,13.));
#9777=CARTESIAN_POINT('Ctrl Pts',(0.694764450219577,-21.9890268624765,0.));
#9778=CARTESIAN_POINT('Ctrl Pts',(0.694764450219577,-21.9890268624765,21.));
#9779=CARTESIAN_POINT('Ctrl Pts',(0.699924103234218,-21.9799122315157,0.));
#9780=CARTESIAN_POINT('Ctrl Pts',(0.699924103234218,-21.9799122315157,21.));
#9781=CARTESIAN_POINT('Ctrl Pts',(0.710218621843551,-21.9616777523685,0.));
#9782=CARTESIAN_POINT('Ctrl Pts',(0.710218621843551,-21.9616777523685,21.));
#9783=CARTESIAN_POINT('Ctrl Pts',(0.725586037496632,-21.9343103819749,0.));
#9784=CARTESIAN_POINT('Ctrl Pts',(0.725586037496632,-21.9343103819749,21.));
#9785=CARTESIAN_POINT('Ctrl Pts',(0.745927151109818,-21.8977892409997,0.));
#9786=CARTESIAN_POINT('Ctrl Pts',(0.745927151109818,-21.8977892409997,21.));
#9787=CARTESIAN_POINT('Ctrl Pts',(0.771105213258327,-21.8520856039249,0.));
#9788=CARTESIAN_POINT('Ctrl Pts',(0.771105213258327,-21.8520856039249,21.));
#9789=CARTESIAN_POINT('Ctrl Pts',(0.796034321106407,-21.8063297959755,0.));
#9790=CARTESIAN_POINT('Ctrl Pts',(0.796034321106407,-21.8063297959755,21.));
#9791=CARTESIAN_POINT('Ctrl Pts',(0.820713597934075,-21.7605219769118,0.));
#9792=CARTESIAN_POINT('Ctrl Pts',(0.820713597934075,-21.7605219769118,21.));
#9793=CARTESIAN_POINT('Ctrl Pts',(0.845141916726555,-21.7146624809285,0.));
#9794=CARTESIAN_POINT('Ctrl Pts',(0.845141916726555,-21.7146624809285,21.));
#9795=CARTESIAN_POINT('Ctrl Pts',(0.869317897714094,-21.6687518829182,0.));
#9796=CARTESIAN_POINT('Ctrl Pts',(0.869317897714094,-21.6687518829182,21.));
#9797=CARTESIAN_POINT('Ctrl Pts',(0.89323996751367,-21.6227909401433,0.));
#9798=CARTESIAN_POINT('Ctrl Pts',(0.89323996751367,-21.6227909401433,21.));
#9799=CARTESIAN_POINT('Ctrl Pts',(0.916906425150851,-21.5767805209408,0.));
#9800=CARTESIAN_POINT('Ctrl Pts',(0.916906425150851,-21.5767805209408,21.));
#9801=CARTESIAN_POINT('Ctrl Pts',(0.940315509525146,-21.5307215366685,0.));
#9802=CARTESIAN_POINT('Ctrl Pts',(0.940315509525146,-21.5307215366685,21.));
#9803=CARTESIAN_POINT('Ctrl Pts',(0.963465462815768,-21.4846148770804,0.));
#9804=CARTESIAN_POINT('Ctrl Pts',(0.963465462815768,-21.4846148770804,21.));
#9805=CARTESIAN_POINT('Ctrl Pts',(0.986354611081129,-21.4384613333266,0.));
#9806=CARTESIAN_POINT('Ctrl Pts',(0.986354611081129,-21.4384613333266,21.));
#9807=CARTESIAN_POINT('Ctrl Pts',(1.00898133629987,-21.3922616124166,0.));
#9808=CARTESIAN_POINT('Ctrl Pts',(1.00898133629987,-21.3922616124166,21.));
#9809=CARTESIAN_POINT('Ctrl Pts',(1.03134402396952,-21.3460163737343,0.));
#9810=CARTESIAN_POINT('Ctrl Pts',(1.03134402396952,-21.3460163737343,21.));
#9811=CARTESIAN_POINT('Ctrl Pts',(1.05344101900192,-21.2997262593683,0.));
#9812=CARTESIAN_POINT('Ctrl Pts',(1.05344101900192,-21.2997262593683,21.));
#9813=CARTESIAN_POINT('Ctrl Pts',(1.07527058431887,-21.2533919248553,0.));
#9814=CARTESIAN_POINT('Ctrl Pts',(1.07527058431887,-21.2533919248553,21.));
#9815=CARTESIAN_POINT('Ctrl Pts',(1.09683084929265,-21.2070140764156,0.));
#9816=CARTESIAN_POINT('Ctrl Pts',(1.09683084929265,-21.2070140764156,21.));
#9817=CARTESIAN_POINT('Ctrl Pts',(1.11811982787746,-21.1605934684164,0.));
#9818=CARTESIAN_POINT('Ctrl Pts',(1.11811982787746,-21.1605934684164,21.));
#9819=CARTESIAN_POINT('Ctrl Pts',(1.13913546246554,-21.1141308858087,0.));
#9820=CARTESIAN_POINT('Ctrl Pts',(1.13913546246554,-21.1141308858087,21.));
#9821=CARTESIAN_POINT('Ctrl Pts',(1.15987566445807,-21.0676271313238,0.));
#9822=CARTESIAN_POINT('Ctrl Pts',(1.15987566445807,-21.0676271313238,21.));
#9823=CARTESIAN_POINT('Ctrl Pts',(1.18033835060894,-21.0210830121673,0.));
#9824=CARTESIAN_POINT('Ctrl Pts',(1.18033835060894,-21.0210830121673,21.));
#9825=CARTESIAN_POINT('Ctrl Pts',(1.20052150219502,-20.9744993243732,0.));
#9826=CARTESIAN_POINT('Ctrl Pts',(1.20052150219502,-20.9744993243732,21.));
#9827=CARTESIAN_POINT('Ctrl Pts',(1.22042312071096,-20.9278768531175,0.));
#9828=CARTESIAN_POINT('Ctrl Pts',(1.22042312071096,-20.9278768531175,21.));
#9829=CARTESIAN_POINT('Ctrl Pts',(1.24004113517905,-20.881216381382,0.));
#9830=CARTESIAN_POINT('Ctrl Pts',(1.24004113517905,-20.881216381382,21.));
#9831=CARTESIAN_POINT('Ctrl Pts',(1.25937332001004,-20.83451869657,0.));
#9832=CARTESIAN_POINT('Ctrl Pts',(1.25937332001004,-20.83451869657,21.));
#9833=CARTESIAN_POINT('Ctrl Pts',(1.27841722479261,-20.7877845975367,0.));
#9834=CARTESIAN_POINT('Ctrl Pts',(1.27841722479261,-20.7877845975367,21.));
#9835=CARTESIAN_POINT('Ctrl Pts',(1.29717006491149,-20.7410149035348,0.));
#9836=CARTESIAN_POINT('Ctrl Pts',(1.29717006491149,-20.7410149035348,21.));
#9837=CARTESIAN_POINT('Ctrl Pts',(1.31562879653596,-20.694210454218,0.));
#9838=CARTESIAN_POINT('Ctrl Pts',(1.31562879653596,-20.694210454218,21.));
#9839=CARTESIAN_POINT('Ctrl Pts',(1.3337902972259,-20.6473721041685,0.));
#9840=CARTESIAN_POINT('Ctrl Pts',(1.3337902972259,-20.6473721041685,21.));
#9841=CARTESIAN_POINT('Ctrl Pts',(1.35165153211252,-20.6005007190809,0.));
#9842=CARTESIAN_POINT('Ctrl Pts',(1.35165153211252,-20.6005007190809,21.));
#9843=CARTESIAN_POINT('Ctrl Pts',(1.36920969340018,-20.5535971721246,0.));
#9844=CARTESIAN_POINT('Ctrl Pts',(1.36920969340018,-20.5535971721246,21.));
#9845=CARTESIAN_POINT('Ctrl Pts',(1.38646244026049,-20.5066623390132,0.));
#9846=CARTESIAN_POINT('Ctrl Pts',(1.38646244026049,-20.5066623390132,21.));
#9847=CARTESIAN_POINT('Ctrl Pts',(1.40340771617024,-20.4596971004275,0.));
#9848=CARTESIAN_POINT('Ctrl Pts',(1.40340771617024,-20.4596971004275,21.));
#9849=CARTESIAN_POINT('Ctrl Pts',(1.42004329463709,-20.4127023494155,0.));
#9850=CARTESIAN_POINT('Ctrl Pts',(1.42004329463709,-20.4127023494155,21.));
#9851=CARTESIAN_POINT('Ctrl Pts',(1.43636637152782,-20.3656789980171,0.));
#9852=CARTESIAN_POINT('Ctrl Pts',(1.43636637152782,-20.3656789980171,21.));
#9853=CARTESIAN_POINT('Ctrl Pts',(1.45237321894403,-20.3186279833818,0.));
#9854=CARTESIAN_POINT('Ctrl Pts',(1.45237321894403,-20.3186279833818,21.));
#9855=CARTESIAN_POINT('Ctrl Pts',(1.4680586180802,-20.2715502770004,0.));
#9856=CARTESIAN_POINT('Ctrl Pts',(1.4680586180802,-20.2715502770004,21.));
#9857=CARTESIAN_POINT('Ctrl Pts',(1.48341623961913,-20.224446881308,0.));
#9858=CARTESIAN_POINT('Ctrl Pts',(1.48341623961913,-20.224446881308,21.));
#9859=CARTESIAN_POINT('Ctrl Pts',(1.49843965844501,-20.1773188177942,0.));
#9860=CARTESIAN_POINT('Ctrl Pts',(1.49843965844501,-20.1773188177942,21.));
#9861=CARTESIAN_POINT('Ctrl Pts',(1.51312326913582,-20.1301671167606,0.));
#9862=CARTESIAN_POINT('Ctrl Pts',(1.51312326913582,-20.1301671167606,21.));
#9863=CARTESIAN_POINT('Ctrl Pts',(1.52746305716964,-20.0829928089241,0.));
#9864=CARTESIAN_POINT('Ctrl Pts',(1.52746305716964,-20.0829928089241,21.));
#9865=CARTESIAN_POINT('Ctrl Pts',(1.54145790302917,-20.0357969106526,0.));
#9866=CARTESIAN_POINT('Ctrl Pts',(1.54145790302917,-20.0357969106526,21.));
#9867=CARTESIAN_POINT('Ctrl Pts',(1.55510860515913,-19.9885804375097,0.));
#9868=CARTESIAN_POINT('Ctrl Pts',(1.55510860515913,-19.9885804375097,21.));
#9869=CARTESIAN_POINT('Ctrl Pts',(1.56841542790452,-19.9413444362352,0.));
#9870=CARTESIAN_POINT('Ctrl Pts',(1.56841542790452,-19.9413444362352,21.));
#9871=CARTESIAN_POINT('Ctrl Pts',(1.58137589158952,-19.8940900137801,0.));
#9872=CARTESIAN_POINT('Ctrl Pts',(1.58137589158952,-19.8940900137801,21.));
#9873=CARTESIAN_POINT('Ctrl Pts',(1.59398289700558,-19.8468183626037,0.));
#9874=CARTESIAN_POINT('Ctrl Pts',(1.59398289700558,-19.8468183626037,21.));
#9875=CARTESIAN_POINT('Ctrl Pts',(1.60622162219699,-19.7995308006834,0.));
#9876=CARTESIAN_POINT('Ctrl Pts',(1.60622162219699,-19.7995308006834,21.));
#9877=CARTESIAN_POINT('Ctrl Pts',(1.61807191996833,-19.7522287462982,0.));
#9878=CARTESIAN_POINT('Ctrl Pts',(1.61807191996833,-19.7522287462982,21.));
#9879=CARTESIAN_POINT('Ctrl Pts',(1.62951389038421,-19.7049136553525,0.));
#9880=CARTESIAN_POINT('Ctrl Pts',(1.62951389038421,-19.7049136553525,21.));
#9881=CARTESIAN_POINT('Ctrl Pts',(1.64053294677821,-19.6575869645839,0.));
#9882=CARTESIAN_POINT('Ctrl Pts',(1.64053294677821,-19.6575869645839,21.));
#9883=CARTESIAN_POINT('Ctrl Pts',(1.65112409599282,-19.6102500448855,0.));
#9884=CARTESIAN_POINT('Ctrl Pts',(1.65112409599282,-19.6102500448855,21.));
#9885=CARTESIAN_POINT('Ctrl Pts',(1.66129908621006,-19.5629041190868,0.));
#9886=CARTESIAN_POINT('Ctrl Pts',(1.66129908621006,-19.5629041190868,21.));
#9887=CARTESIAN_POINT('Ctrl Pts',(1.67107974760948,-19.5155503513712,0.));
#9888=CARTESIAN_POINT('Ctrl Pts',(1.67107974760948,-19.5155503513712,21.));
#9889=CARTESIAN_POINT('Ctrl Pts',(1.68048476382294,-19.4681900187091,0.));
#9890=CARTESIAN_POINT('Ctrl Pts',(1.68048476382294,-19.4681900187091,21.));
#9891=CARTESIAN_POINT('Ctrl Pts',(1.6895175323357,-19.4208246682917,0.));
#9892=CARTESIAN_POINT('Ctrl Pts',(1.6895175323357,-19.4208246682917,21.));
#9893=CARTESIAN_POINT('Ctrl Pts',(1.69815571801251,-19.3734562555057,0.));
#9894=CARTESIAN_POINT('Ctrl Pts',(1.69815571801251,-19.3734562555057,21.));
#9895=CARTESIAN_POINT('Ctrl Pts',(1.70633457265124,-19.3260873558094,0.));
#9896=CARTESIAN_POINT('Ctrl Pts',(1.70633457265124,-19.3260873558094,21.));
#9897=CARTESIAN_POINT('Ctrl Pts',(1.71396454346262,-19.2787209722437,0.));
#9898=CARTESIAN_POINT('Ctrl Pts',(1.71396454346262,-19.2787209722437,21.));
#9899=CARTESIAN_POINT('Ctrl Pts',(1.72096104670233,-19.2313602042899,0.));
#9900=CARTESIAN_POINT('Ctrl Pts',(1.72096104670233,-19.2313602042899,21.));
#9901=CARTESIAN_POINT('Ctrl Pts',(1.72727220327097,-19.1840079312107,0.));
#9902=CARTESIAN_POINT('Ctrl Pts',(1.72727220327097,-19.1840079312107,21.));
#9903=CARTESIAN_POINT('Ctrl Pts',(1.73290313712353,-19.1366665585833,0.));
#9904=CARTESIAN_POINT('Ctrl Pts',(1.73290313712353,-19.1366665585833,21.));
#9905=CARTESIAN_POINT('Ctrl Pts',(1.7379530116984,-19.0893375576541,0.));
#9906=CARTESIAN_POINT('Ctrl Pts',(1.7379530116984,-19.0893375576541,21.));
#9907=CARTESIAN_POINT('Ctrl Pts',(1.74256297552948,-19.0420224296189,0.));
#9908=CARTESIAN_POINT('Ctrl Pts',(1.74256297552948,-19.0420224296189,21.));
#9909=CARTESIAN_POINT('Ctrl Pts',(1.74684309825012,-18.9947239970259,0.));
#9910=CARTESIAN_POINT('Ctrl Pts',(1.74684309825012,-18.9947239970259,21.));
#9911=CARTESIAN_POINT('Ctrl Pts',(1.75080409924533,-18.947447637865,0.));
#9912=CARTESIAN_POINT('Ctrl Pts',(1.75080409924533,-18.947447637865,21.));
#9913=CARTESIAN_POINT('Ctrl Pts',(1.75429229572775,-18.9002024267872,0.));
#9914=CARTESIAN_POINT('Ctrl Pts',(1.75429229572775,-18.9002024267872,21.));
#9915=CARTESIAN_POINT('Ctrl Pts',(1.75690876962597,-18.8530026395886,0.));
#9916=CARTESIAN_POINT('Ctrl Pts',(1.75690876962597,-18.8530026395886,21.));
#9917=CARTESIAN_POINT('Ctrl Pts',(1.7581175236483,-18.8058650094753,0.));
#9918=CARTESIAN_POINT('Ctrl Pts',(1.7581175236483,-18.8058650094753,21.));
#9919=CARTESIAN_POINT('Ctrl Pts',(1.75752447968136,-18.7682173836138,0.));
#9920=CARTESIAN_POINT('Ctrl Pts',(1.75752447968136,-18.7682173836138,21.));
#9921=CARTESIAN_POINT('Ctrl Pts',(1.75601041697575,-18.7400222442427,0.));
#9922=CARTESIAN_POINT('Ctrl Pts',(1.75601041697575,-18.7400222442427,21.));
#9923=CARTESIAN_POINT('Ctrl Pts',(1.75450132833463,-18.7212441956871,0.));
#9924=CARTESIAN_POINT('Ctrl Pts',(1.75450132833463,-18.7212441956871,21.));
#9925=CARTESIAN_POINT('Ctrl Pts',(1.75362185428836,-18.7118598491961,0.));
#9926=CARTESIAN_POINT('Ctrl Pts',(1.75362185428836,-18.7118598491961,21.));
#9927=CARTESIAN_POINT('',(0.69476445021964,-21.9890268624765,0.));
#9928=CARTESIAN_POINT('Ctrl Pts',(1.75362185428836,-18.7118598491961,0.));
#9929=CARTESIAN_POINT('Ctrl Pts',(1.75450132833463,-18.7212441956871,0.));
#9930=CARTESIAN_POINT('Ctrl Pts',(1.75601041697575,-18.7400222442427,0.));
#9931=CARTESIAN_POINT('Ctrl Pts',(1.75752447968136,-18.7682173836138,0.));
#9932=CARTESIAN_POINT('Ctrl Pts',(1.7581175236483,-18.8058650094753,0.));
#9933=CARTESIAN_POINT('Ctrl Pts',(1.75690876962597,-18.8530026395886,0.));
#9934=CARTESIAN_POINT('Ctrl Pts',(1.75429229572775,-18.9002024267872,0.));
#9935=CARTESIAN_POINT('Ctrl Pts',(1.75080409924533,-18.947447637865,0.));
#9936=CARTESIAN_POINT('Ctrl Pts',(1.74684309825012,-18.9947239970259,0.));
#9937=CARTESIAN_POINT('Ctrl Pts',(1.74256297552948,-19.0420224296189,0.));
#9938=CARTESIAN_POINT('Ctrl Pts',(1.7379530116984,-19.0893375576541,0.));
#9939=CARTESIAN_POINT('Ctrl Pts',(1.73290313712353,-19.1366665585833,0.));
#9940=CARTESIAN_POINT('Ctrl Pts',(1.72727220327097,-19.1840079312107,0.));
#9941=CARTESIAN_POINT('Ctrl Pts',(1.72096104670233,-19.2313602042899,0.));
#9942=CARTESIAN_POINT('Ctrl Pts',(1.71396454346262,-19.2787209722437,0.));
#9943=CARTESIAN_POINT('Ctrl Pts',(1.70633457265124,-19.3260873558094,0.));
#9944=CARTESIAN_POINT('Ctrl Pts',(1.69815571801251,-19.3734562555057,0.));
#9945=CARTESIAN_POINT('Ctrl Pts',(1.6895175323357,-19.4208246682917,0.));
#9946=CARTESIAN_POINT('Ctrl Pts',(1.68048476382294,-19.4681900187091,0.));
#9947=CARTESIAN_POINT('Ctrl Pts',(1.67107974760948,-19.5155503513712,0.));
#9948=CARTESIAN_POINT('Ctrl Pts',(1.66129908621006,-19.5629041190868,0.));
#9949=CARTESIAN_POINT('Ctrl Pts',(1.65112409599282,-19.6102500448855,0.));
#9950=CARTESIAN_POINT('Ctrl Pts',(1.64053294677821,-19.6575869645839,0.));
#9951=CARTESIAN_POINT('Ctrl Pts',(1.62951389038421,-19.7049136553525,0.));
#9952=CARTESIAN_POINT('Ctrl Pts',(1.61807191996833,-19.7522287462982,0.));
#9953=CARTESIAN_POINT('Ctrl Pts',(1.60622162219699,-19.7995308006834,0.));
#9954=CARTESIAN_POINT('Ctrl Pts',(1.59398289700558,-19.8468183626037,0.));
#9955=CARTESIAN_POINT('Ctrl Pts',(1.58137589158952,-19.8940900137801,0.));
#9956=CARTESIAN_POINT('Ctrl Pts',(1.56841542790452,-19.9413444362352,0.));
#9957=CARTESIAN_POINT('Ctrl Pts',(1.55510860515913,-19.9885804375097,0.));
#9958=CARTESIAN_POINT('Ctrl Pts',(1.54145790302917,-20.0357969106526,0.));
#9959=CARTESIAN_POINT('Ctrl Pts',(1.52746305716964,-20.0829928089241,0.));
#9960=CARTESIAN_POINT('Ctrl Pts',(1.51312326913582,-20.1301671167606,0.));
#9961=CARTESIAN_POINT('Ctrl Pts',(1.49843965844501,-20.1773188177942,0.));
#9962=CARTESIAN_POINT('Ctrl Pts',(1.48341623961913,-20.224446881308,0.));
#9963=CARTESIAN_POINT('Ctrl Pts',(1.4680586180802,-20.2715502770004,0.));
#9964=CARTESIAN_POINT('Ctrl Pts',(1.45237321894403,-20.3186279833818,0.));
#9965=CARTESIAN_POINT('Ctrl Pts',(1.43636637152782,-20.3656789980171,0.));
#9966=CARTESIAN_POINT('Ctrl Pts',(1.42004329463709,-20.4127023494155,0.));
#9967=CARTESIAN_POINT('Ctrl Pts',(1.40340771617024,-20.4596971004275,0.));
#9968=CARTESIAN_POINT('Ctrl Pts',(1.38646244026049,-20.5066623390132,0.));
#9969=CARTESIAN_POINT('Ctrl Pts',(1.36920969340018,-20.5535971721246,0.));
#9970=CARTESIAN_POINT('Ctrl Pts',(1.35165153211252,-20.6005007190809,0.));
#9971=CARTESIAN_POINT('Ctrl Pts',(1.3337902972259,-20.6473721041685,0.));
#9972=CARTESIAN_POINT('Ctrl Pts',(1.31562879653596,-20.694210454218,0.));
#9973=CARTESIAN_POINT('Ctrl Pts',(1.29717006491149,-20.7410149035348,0.));
#9974=CARTESIAN_POINT('Ctrl Pts',(1.27841722479261,-20.7877845975367,0.));
#9975=CARTESIAN_POINT('Ctrl Pts',(1.25937332001004,-20.83451869657,0.));
#9976=CARTESIAN_POINT('Ctrl Pts',(1.24004113517905,-20.881216381382,0.));
#9977=CARTESIAN_POINT('Ctrl Pts',(1.22042312071096,-20.9278768531175,0.));
#9978=CARTESIAN_POINT('Ctrl Pts',(1.20052150219502,-20.9744993243732,0.));
#9979=CARTESIAN_POINT('Ctrl Pts',(1.18033835060894,-21.0210830121673,0.));
#9980=CARTESIAN_POINT('Ctrl Pts',(1.15987566445807,-21.0676271313238,0.));
#9981=CARTESIAN_POINT('Ctrl Pts',(1.13913546246554,-21.1141308858087,0.));
#9982=CARTESIAN_POINT('Ctrl Pts',(1.11811982787746,-21.1605934684164,0.));
#9983=CARTESIAN_POINT('Ctrl Pts',(1.09683084929265,-21.2070140764156,0.));
#9984=CARTESIAN_POINT('Ctrl Pts',(1.07527058431887,-21.2533919248553,0.));
#9985=CARTESIAN_POINT('Ctrl Pts',(1.05344101900192,-21.2997262593683,0.));
#9986=CARTESIAN_POINT('Ctrl Pts',(1.03134402396952,-21.3460163737343,0.));
#9987=CARTESIAN_POINT('Ctrl Pts',(1.00898133629987,-21.3922616124166,0.));
#9988=CARTESIAN_POINT('Ctrl Pts',(0.986354611081129,-21.4384613333266,0.));
#9989=CARTESIAN_POINT('Ctrl Pts',(0.963465462815768,-21.4846148770804,0.));
#9990=CARTESIAN_POINT('Ctrl Pts',(0.940315509525146,-21.5307215366685,0.));
#9991=CARTESIAN_POINT('Ctrl Pts',(0.916906425150851,-21.5767805209408,0.));
#9992=CARTESIAN_POINT('Ctrl Pts',(0.89323996751367,-21.6227909401433,0.));
#9993=CARTESIAN_POINT('Ctrl Pts',(0.869317897714094,-21.6687518829182,0.));
#9994=CARTESIAN_POINT('Ctrl Pts',(0.845141916726555,-21.7146624809285,0.));
#9995=CARTESIAN_POINT('Ctrl Pts',(0.820713597934075,-21.7605219769118,0.));
#9996=CARTESIAN_POINT('Ctrl Pts',(0.796034321106407,-21.8063297959755,0.));
#9997=CARTESIAN_POINT('Ctrl Pts',(0.76611939168871,-21.8612367655148,0.));
#9998=CARTESIAN_POINT('Ctrl Pts',(0.740879090965094,-21.9069273598709,0.));
#9999=CARTESIAN_POINT('Ctrl Pts',(0.720488353007144,-21.9434380560096,0.));
#10000=CARTESIAN_POINT('Ctrl Pts',(0.705083756261754,-21.970797600548,0.));
#10001=CARTESIAN_POINT('Ctrl Pts',(0.694764450219577,-21.9890268624765,
0.));
#10002=CARTESIAN_POINT('',(0.69476445021964,-21.9890268624765,13.));
#10003=CARTESIAN_POINT('Ctrl Pts',(0.694764450219577,-21.9890268624765,
13.));
#10004=CARTESIAN_POINT('Ctrl Pts',(0.745561803311463,-21.89929231523,13.));
#10005=CARTESIAN_POINT('Ctrl Pts',(0.794921865619054,-21.8092529629783,
13.));
#10006=CARTESIAN_POINT('Ctrl Pts',(0.842819260998952,-21.7189137535649,
13.));
#10007=CARTESIAN_POINT('Ctrl Pts',(0.922187324214976,-21.569217762233,13.));
#10008=CARTESIAN_POINT('Ctrl Pts',(0.997528955778406,-21.4187072720354,
13.));
#10009=CARTESIAN_POINT('Ctrl Pts',(1.06858105435695,-21.2675022574599,13.));
#10010=CARTESIAN_POINT('Ctrl Pts',(1.12319586370563,-21.1512772168374,13.));
#10011=CARTESIAN_POINT('Ctrl Pts',(1.17527598698666,-21.0346391550274,13.));
#10012=CARTESIAN_POINT('Ctrl Pts',(1.22467603889823,-20.9176442421133,13.));
#10013=CARTESIAN_POINT('Ctrl Pts',(1.27785400463397,-20.7917020370051,13.));
#10014=CARTESIAN_POINT('Ctrl Pts',(1.32793259719133,-20.6653453730115,13.));
#10015=CARTESIAN_POINT('Ctrl Pts',(1.37465955747084,-20.5386490816447,13.));
#10016=CARTESIAN_POINT('Ctrl Pts',(1.40052887204096,-20.468506572981,13.));
#10017=CARTESIAN_POINT('Ctrl Pts',(1.42537603793014,-20.3982600553259,13.));
#10018=CARTESIAN_POINT('Ctrl Pts',(1.44915458926219,-20.3279233153994,13.));
#10019=CARTESIAN_POINT('Ctrl Pts',(1.47206853368884,-20.2601440748846,13.));
#10020=CARTESIAN_POINT('Ctrl Pts',(1.49398338587319,-20.1922811201552,13.));
#10021=CARTESIAN_POINT('Ctrl Pts',(1.51482335690232,-20.1243481792969,13.));
#10022=CARTESIAN_POINT('Ctrl Pts',(1.53283548327962,-20.0656332840501,13.));
#10023=CARTESIAN_POINT('Ctrl Pts',(1.55004791413554,-20.0068660725075,13.));
#10024=CARTESIAN_POINT('Ctrl Pts',(1.56645839123305,-19.9480555843418,13.));
#10025=CARTESIAN_POINT('Ctrl Pts',(1.57823544812775,-19.9058499579596,13.));
#10026=CARTESIAN_POINT('Ctrl Pts',(1.58960230205608,-19.8636220212356,13.));
#10027=CARTESIAN_POINT('Ctrl Pts',(1.60051957198611,-19.8213758753108,13.));
#10028=CARTESIAN_POINT('Ctrl Pts',(1.61125906786244,-19.7798176549079,13.));
#10029=CARTESIAN_POINT('Ctrl Pts',(1.62155711722061,-19.7382418852391,13.));
#10030=CARTESIAN_POINT('Ctrl Pts',(1.63136143467465,-19.6966529622227,13.));
#10031=CARTESIAN_POINT('Ctrl Pts',(1.63986235386958,-19.6605929227937,13.));
#10032=CARTESIAN_POINT('Ctrl Pts',(1.64798961240502,-19.6245230266729,13.));
#10033=CARTESIAN_POINT('Ctrl Pts',(1.65575861443972,-19.5884457884257,13.));
#10034=CARTESIAN_POINT('Ctrl Pts',(1.66279554775982,-19.5557680881516,13.));
#10035=CARTESIAN_POINT('Ctrl Pts',(1.66954412476468,-19.5230842956051,13.));
#10036=CARTESIAN_POINT('Ctrl Pts',(1.67602787914578,-19.49039635302,13.));
#10037=CARTESIAN_POINT('Ctrl Pts',(1.68148945136204,-19.462861756776,13.));
#10038=CARTESIAN_POINT('Ctrl Pts',(1.68676485585863,-19.4353241970144,13.));
#10039=CARTESIAN_POINT('Ctrl Pts',(1.69183425656632,-19.4077853970595,13.));
#10040=CARTESIAN_POINT('Ctrl Pts',(1.69917023100168,-19.3679337569745,13.));
#10041=CARTESIAN_POINT('Ctrl Pts',(1.70607400306928,-19.3280794803457,13.));
#10042=CARTESIAN_POINT('Ctrl Pts',(1.71232694131222,-19.2882303922902,13.));
#10043=CARTESIAN_POINT('Ctrl Pts',(1.71610520915756,-19.2641520274933,13.));
#10044=CARTESIAN_POINT('Ctrl Pts',(1.71964237041073,-19.2400756155396,13.));
#10045=CARTESIAN_POINT('Ctrl Pts',(1.72291205972096,-19.2160028181149,13.));
#10046=CARTESIAN_POINT('Ctrl Pts',(1.72592763308942,-19.1938009267636,13.));
#10047=CARTESIAN_POINT('Ctrl Pts',(1.7287143697234,-19.1716021264808,13.));
#10048=CARTESIAN_POINT('Ctrl Pts',(1.73129733456843,-19.1494073125539,13.));
#10049=CARTESIAN_POINT('Ctrl Pts',(1.73485046445803,-19.1188760968816,13.));
#10050=CARTESIAN_POINT('Ctrl Pts',(1.7380253099616,-19.0883522198199,13.));
#10051=CARTESIAN_POINT('Ctrl Pts',(1.74097263876108,-19.0578380260755,13.));
#10052=CARTESIAN_POINT('Ctrl Pts',(1.74284247673618,-19.0384792771458,13.));
#10053=CARTESIAN_POINT('Ctrl Pts',(1.74462241723582,-19.0191244316077,13.));
#10054=CARTESIAN_POINT('Ctrl Pts',(1.74632097575636,-18.9997750007207,13.));
#10055=CARTESIAN_POINT('Ctrl Pts',(1.74784535296742,-18.9824097871383,13.));
#10056=CARTESIAN_POINT('Ctrl Pts',(1.74930491161338,-18.9650489252781,13.));
#10057=CARTESIAN_POINT('Ctrl Pts',(1.75066513119224,-18.9476944344223,13.));
#10058=CARTESIAN_POINT('Ctrl Pts',(1.75209499287337,-18.9294514081815,13.));
#10059=CARTESIAN_POINT('Ctrl Pts',(1.75341524153271,-18.9112154259254,13.));
#10060=CARTESIAN_POINT('Ctrl Pts',(1.75452347864582,-18.8929901415011,13.));
#10061=CARTESIAN_POINT('Ctrl Pts',(1.75636425803994,-18.8627179843758,13.));
#10062=CARTESIAN_POINT('Ctrl Pts',(1.75761169393786,-18.8324756678787,13.));
#10063=CARTESIAN_POINT('Ctrl Pts',(1.75764008468136,-18.8022820950489,13.));
#10064=CARTESIAN_POINT('Ctrl Pts',(1.75765574034772,-18.785632284429,13.));
#10065=CARTESIAN_POINT('Ctrl Pts',(1.75729933637223,-18.7689972917426,13.));
#10066=CARTESIAN_POINT('Ctrl Pts',(1.75649392368161,-18.7523793044392,13.));
#10067=CARTESIAN_POINT('Ctrl Pts',(1.7558387619977,-18.7388614288561,13.));
#10068=CARTESIAN_POINT('Ctrl Pts',(1.75488656240343,-18.7253548001979,13.));
#10069=CARTESIAN_POINT('Ctrl Pts',(1.75362185428836,-18.7118598491961,13.));
#10070=CARTESIAN_POINT('',(0.69476445021964,-21.9890268624765,0.));
#10071=CARTESIAN_POINT('Origin',(-1.0097419586829E-27,-5.6665783176868E-12,
0.));
#10072=CARTESIAN_POINT('',(-0.694764450219586,-21.9890268624765,0.));
#10073=CARTESIAN_POINT('Origin',(-1.0097419586829E-27,-5.6665783176868E-12,
0.));
#10074=CARTESIAN_POINT('',(-0.694764450219586,-21.9890268624765,13.));
#10075=CARTESIAN_POINT('Origin',(-1.0097419586829E-27,-5.6665783176868E-12,
13.));
#10076=CARTESIAN_POINT('',(-0.694764450219586,-21.9890268624765,0.));
#10077=CARTESIAN_POINT('Ctrl Pts',(-1.75362185428837,-18.7118598491961,
0.));
#10078=CARTESIAN_POINT('Ctrl Pts',(-1.75362185428837,-18.7118598491961,
21.));
#10079=CARTESIAN_POINT('Ctrl Pts',(-1.75450132833464,-18.7212441956871,
0.));
#10080=CARTESIAN_POINT('Ctrl Pts',(-1.75450132833464,-18.7212441956871,
21.));
#10081=CARTESIAN_POINT('Ctrl Pts',(-1.75601041697575,-18.7400222442427,
0.));
#10082=CARTESIAN_POINT('Ctrl Pts',(-1.75601041697575,-18.7400222442427,
21.));
#10083=CARTESIAN_POINT('Ctrl Pts',(-1.75752447968136,-18.7682173836138,
0.));
#10084=CARTESIAN_POINT('Ctrl Pts',(-1.75752447968136,-18.7682173836138,
21.));
#10085=CARTESIAN_POINT('Ctrl Pts',(-1.7581175236483,-18.8058650094753,0.));
#10086=CARTESIAN_POINT('Ctrl Pts',(-1.7581175236483,-18.8058650094753,21.));
#10087=CARTESIAN_POINT('Ctrl Pts',(-1.75690876962598,-18.8530026395886,
0.));
#10088=CARTESIAN_POINT('Ctrl Pts',(-1.75690876962598,-18.8530026395886,
21.));
#10089=CARTESIAN_POINT('Ctrl Pts',(-1.75429229572776,-18.9002024267872,
0.));
#10090=CARTESIAN_POINT('Ctrl Pts',(-1.75429229572776,-18.9002024267872,
21.));
#10091=CARTESIAN_POINT('Ctrl Pts',(-1.75080409924534,-18.947447637865,0.));
#10092=CARTESIAN_POINT('Ctrl Pts',(-1.75080409924534,-18.947447637865,21.));
#10093=CARTESIAN_POINT('Ctrl Pts',(-1.74684309825013,-18.9947239970259,
0.));
#10094=CARTESIAN_POINT('Ctrl Pts',(-1.74684309825013,-18.9947239970259,
21.));
#10095=CARTESIAN_POINT('Ctrl Pts',(-1.74256297552949,-19.0420224296189,
0.));
#10096=CARTESIAN_POINT('Ctrl Pts',(-1.74256297552949,-19.0420224296189,
21.));
#10097=CARTESIAN_POINT('Ctrl Pts',(-1.73795301169841,-19.0893375576541,
0.));
#10098=CARTESIAN_POINT('Ctrl Pts',(-1.73795301169841,-19.0893375576541,
21.));
#10099=CARTESIAN_POINT('Ctrl Pts',(-1.73290313712354,-19.1366665585833,
0.));
#10100=CARTESIAN_POINT('Ctrl Pts',(-1.73290313712354,-19.1366665585833,
21.));
#10101=CARTESIAN_POINT('Ctrl Pts',(-1.72727220327098,-19.1840079312107,
0.));
#10102=CARTESIAN_POINT('Ctrl Pts',(-1.72727220327098,-19.1840079312107,
21.));
#10103=CARTESIAN_POINT('Ctrl Pts',(-1.72096104670234,-19.2313602042899,
0.));
#10104=CARTESIAN_POINT('Ctrl Pts',(-1.72096104670234,-19.2313602042899,
21.));
#10105=CARTESIAN_POINT('Ctrl Pts',(-1.71396454346262,-19.2787209722437,
0.));
#10106=CARTESIAN_POINT('Ctrl Pts',(-1.71396454346262,-19.2787209722437,
21.));
#10107=CARTESIAN_POINT('Ctrl Pts',(-1.70633457265124,-19.3260873558094,
0.));
#10108=CARTESIAN_POINT('Ctrl Pts',(-1.70633457265124,-19.3260873558094,
21.));
#10109=CARTESIAN_POINT('Ctrl Pts',(-1.69815571801252,-19.3734562555057,
0.));
#10110=CARTESIAN_POINT('Ctrl Pts',(-1.69815571801252,-19.3734562555057,
21.));
#10111=CARTESIAN_POINT('Ctrl Pts',(-1.68951753233571,-19.4208246682917,
0.));
#10112=CARTESIAN_POINT('Ctrl Pts',(-1.68951753233571,-19.4208246682917,
21.));
#10113=CARTESIAN_POINT('Ctrl Pts',(-1.68048476382294,-19.4681900187091,
0.));
#10114=CARTESIAN_POINT('Ctrl Pts',(-1.68048476382294,-19.4681900187091,
21.));
#10115=CARTESIAN_POINT('Ctrl Pts',(-1.67107974760949,-19.5155503513712,
0.));
#10116=CARTESIAN_POINT('Ctrl Pts',(-1.67107974760949,-19.5155503513712,
21.));
#10117=CARTESIAN_POINT('Ctrl Pts',(-1.66129908621006,-19.5629041190868,
0.));
#10118=CARTESIAN_POINT('Ctrl Pts',(-1.66129908621006,-19.5629041190868,
21.));
#10119=CARTESIAN_POINT('Ctrl Pts',(-1.65112409599283,-19.6102500448855,
0.));
#10120=CARTESIAN_POINT('Ctrl Pts',(-1.65112409599283,-19.6102500448855,
21.));
#10121=CARTESIAN_POINT('Ctrl Pts',(-1.64053294677822,-19.6575869645839,
0.));
#10122=CARTESIAN_POINT('Ctrl Pts',(-1.64053294677822,-19.6575869645839,
21.));
#10123=CARTESIAN_POINT('Ctrl Pts',(-1.62951389038422,-19.7049136553525,
0.));
#10124=CARTESIAN_POINT('Ctrl Pts',(-1.62951389038422,-19.7049136553525,
21.));
#10125=CARTESIAN_POINT('Ctrl Pts',(-1.61807191996834,-19.7522287462982,
0.));
#10126=CARTESIAN_POINT('Ctrl Pts',(-1.61807191996834,-19.7522287462982,
21.));
#10127=CARTESIAN_POINT('Ctrl Pts',(-1.60622162219699,-19.7995308006834,
0.));
#10128=CARTESIAN_POINT('Ctrl Pts',(-1.60622162219699,-19.7995308006834,
21.));
#10129=CARTESIAN_POINT('Ctrl Pts',(-1.59398289700559,-19.8468183626037,
0.));
#10130=CARTESIAN_POINT('Ctrl Pts',(-1.59398289700559,-19.8468183626037,
21.));
#10131=CARTESIAN_POINT('Ctrl Pts',(-1.58137589158952,-19.8940900137801,
0.));
#10132=CARTESIAN_POINT('Ctrl Pts',(-1.58137589158952,-19.8940900137801,
21.));
#10133=CARTESIAN_POINT('Ctrl Pts',(-1.56841542790453,-19.9413444362352,
0.));
#10134=CARTESIAN_POINT('Ctrl Pts',(-1.56841542790453,-19.9413444362352,
21.));
#10135=CARTESIAN_POINT('Ctrl Pts',(-1.55510860515914,-19.9885804375096,
0.));
#10136=CARTESIAN_POINT('Ctrl Pts',(-1.55510860515914,-19.9885804375096,
21.));
#10137=CARTESIAN_POINT('Ctrl Pts',(-1.54145790302918,-20.0357969106526,
0.));
#10138=CARTESIAN_POINT('Ctrl Pts',(-1.54145790302918,-20.0357969106526,
21.));
#10139=CARTESIAN_POINT('Ctrl Pts',(-1.52746305716965,-20.0829928089241,
0.));
#10140=CARTESIAN_POINT('Ctrl Pts',(-1.52746305716965,-20.0829928089241,
21.));
#10141=CARTESIAN_POINT('Ctrl Pts',(-1.51312326913583,-20.1301671167606,
0.));
#10142=CARTESIAN_POINT('Ctrl Pts',(-1.51312326913583,-20.1301671167606,
21.));
#10143=CARTESIAN_POINT('Ctrl Pts',(-1.49843965844502,-20.1773188177942,
0.));
#10144=CARTESIAN_POINT('Ctrl Pts',(-1.49843965844502,-20.1773188177942,
21.));
#10145=CARTESIAN_POINT('Ctrl Pts',(-1.48341623961914,-20.224446881308,0.));
#10146=CARTESIAN_POINT('Ctrl Pts',(-1.48341623961914,-20.224446881308,21.));
#10147=CARTESIAN_POINT('Ctrl Pts',(-1.46805861808021,-20.2715502770004,
0.));
#10148=CARTESIAN_POINT('Ctrl Pts',(-1.46805861808021,-20.2715502770004,
21.));
#10149=CARTESIAN_POINT('Ctrl Pts',(-1.45237321894404,-20.3186279833818,
0.));
#10150=CARTESIAN_POINT('Ctrl Pts',(-1.45237321894404,-20.3186279833818,
21.));
#10151=CARTESIAN_POINT('Ctrl Pts',(-1.43636637152782,-20.3656789980171,
0.));
#10152=CARTESIAN_POINT('Ctrl Pts',(-1.43636637152782,-20.3656789980171,
21.));
#10153=CARTESIAN_POINT('Ctrl Pts',(-1.4200432946371,-20.4127023494155,0.));
#10154=CARTESIAN_POINT('Ctrl Pts',(-1.4200432946371,-20.4127023494155,21.));
#10155=CARTESIAN_POINT('Ctrl Pts',(-1.40340771617025,-20.4596971004275,
0.));
#10156=CARTESIAN_POINT('Ctrl Pts',(-1.40340771617025,-20.4596971004275,
21.));
#10157=CARTESIAN_POINT('Ctrl Pts',(-1.38646244026049,-20.5066623390132,
0.));
#10158=CARTESIAN_POINT('Ctrl Pts',(-1.38646244026049,-20.5066623390132,
21.));
#10159=CARTESIAN_POINT('Ctrl Pts',(-1.36920969340018,-20.5535971721246,
0.));
#10160=CARTESIAN_POINT('Ctrl Pts',(-1.36920969340018,-20.5535971721246,
21.));
#10161=CARTESIAN_POINT('Ctrl Pts',(-1.35165153211253,-20.6005007190809,
0.));
#10162=CARTESIAN_POINT('Ctrl Pts',(-1.35165153211253,-20.6005007190809,
21.));
#10163=CARTESIAN_POINT('Ctrl Pts',(-1.33379029722591,-20.6473721041685,
0.));
#10164=CARTESIAN_POINT('Ctrl Pts',(-1.33379029722591,-20.6473721041685,
21.));
#10165=CARTESIAN_POINT('Ctrl Pts',(-1.31562879653597,-20.694210454218,0.));
#10166=CARTESIAN_POINT('Ctrl Pts',(-1.31562879653597,-20.694210454218,21.));
#10167=CARTESIAN_POINT('Ctrl Pts',(-1.2971700649115,-20.7410149035348,0.));
#10168=CARTESIAN_POINT('Ctrl Pts',(-1.2971700649115,-20.7410149035348,21.));
#10169=CARTESIAN_POINT('Ctrl Pts',(-1.27841722479262,-20.7877845975367,
0.));
#10170=CARTESIAN_POINT('Ctrl Pts',(-1.27841722479262,-20.7877845975367,
21.));
#10171=CARTESIAN_POINT('Ctrl Pts',(-1.25937332001005,-20.83451869657,0.));
#10172=CARTESIAN_POINT('Ctrl Pts',(-1.25937332001005,-20.83451869657,21.));
#10173=CARTESIAN_POINT('Ctrl Pts',(-1.24004113517906,-20.881216381382,0.));
#10174=CARTESIAN_POINT('Ctrl Pts',(-1.24004113517906,-20.881216381382,21.));
#10175=CARTESIAN_POINT('Ctrl Pts',(-1.22042312071097,-20.9278768531175,
0.));
#10176=CARTESIAN_POINT('Ctrl Pts',(-1.22042312071097,-20.9278768531175,
21.));
#10177=CARTESIAN_POINT('Ctrl Pts',(-1.20052150219503,-20.9744993243732,
0.));
#10178=CARTESIAN_POINT('Ctrl Pts',(-1.20052150219503,-20.9744993243732,
21.));
#10179=CARTESIAN_POINT('Ctrl Pts',(-1.18033835060895,-21.0210830121673,
0.));
#10180=CARTESIAN_POINT('Ctrl Pts',(-1.18033835060895,-21.0210830121673,
21.));
#10181=CARTESIAN_POINT('Ctrl Pts',(-1.15987566445808,-21.0676271313238,
0.));
#10182=CARTESIAN_POINT('Ctrl Pts',(-1.15987566445808,-21.0676271313238,
21.));
#10183=CARTESIAN_POINT('Ctrl Pts',(-1.13913546246555,-21.1141308858087,
0.));
#10184=CARTESIAN_POINT('Ctrl Pts',(-1.13913546246555,-21.1141308858087,
21.));
#10185=CARTESIAN_POINT('Ctrl Pts',(-1.11811982787747,-21.1605934684164,
0.));
#10186=CARTESIAN_POINT('Ctrl Pts',(-1.11811982787747,-21.1605934684164,
21.));
#10187=CARTESIAN_POINT('Ctrl Pts',(-1.09683084929266,-21.2070140764156,
0.));
#10188=CARTESIAN_POINT('Ctrl Pts',(-1.09683084929266,-21.2070140764156,
21.));
#10189=CARTESIAN_POINT('Ctrl Pts',(-1.07527058431887,-21.2533919248553,
0.));
#10190=CARTESIAN_POINT('Ctrl Pts',(-1.07527058431887,-21.2533919248553,
21.));
#10191=CARTESIAN_POINT('Ctrl Pts',(-1.05344101900192,-21.2997262593683,
0.));
#10192=CARTESIAN_POINT('Ctrl Pts',(-1.05344101900192,-21.2997262593683,
21.));
#10193=CARTESIAN_POINT('Ctrl Pts',(-1.03134402396953,-21.3460163737343,
0.));
#10194=CARTESIAN_POINT('Ctrl Pts',(-1.03134402396953,-21.3460163737343,
21.));
#10195=CARTESIAN_POINT('Ctrl Pts',(-1.00898133629988,-21.3922616124166,
0.));
#10196=CARTESIAN_POINT('Ctrl Pts',(-1.00898133629988,-21.3922616124166,
21.));
#10197=CARTESIAN_POINT('Ctrl Pts',(-0.986354611081139,-21.4384613333266,
0.));
#10198=CARTESIAN_POINT('Ctrl Pts',(-0.986354611081139,-21.4384613333266,
21.));
#10199=CARTESIAN_POINT('Ctrl Pts',(-0.963465462815776,-21.4846148770804,
0.));
#10200=CARTESIAN_POINT('Ctrl Pts',(-0.963465462815776,-21.4846148770804,
21.));
#10201=CARTESIAN_POINT('Ctrl Pts',(-0.940315509525156,-21.5307215366685,
0.));
#10202=CARTESIAN_POINT('Ctrl Pts',(-0.940315509525156,-21.5307215366685,
21.));
#10203=CARTESIAN_POINT('Ctrl Pts',(-0.916906425150857,-21.5767805209408,
0.));
#10204=CARTESIAN_POINT('Ctrl Pts',(-0.916906425150857,-21.5767805209408,
21.));
#10205=CARTESIAN_POINT('Ctrl Pts',(-0.893239967513677,-21.6227909401433,
0.));
#10206=CARTESIAN_POINT('Ctrl Pts',(-0.893239967513677,-21.6227909401433,
21.));
#10207=CARTESIAN_POINT('Ctrl Pts',(-0.869317897714105,-21.6687518829182,
0.));
#10208=CARTESIAN_POINT('Ctrl Pts',(-0.869317897714105,-21.6687518829182,
21.));
#10209=CARTESIAN_POINT('Ctrl Pts',(-0.845141916726563,-21.7146624809285,
0.));
#10210=CARTESIAN_POINT('Ctrl Pts',(-0.845141916726563,-21.7146624809285,
21.));
#10211=CARTESIAN_POINT('Ctrl Pts',(-0.820713597934081,-21.7605219769118,
0.));
#10212=CARTESIAN_POINT('Ctrl Pts',(-0.820713597934081,-21.7605219769118,
21.));
#10213=CARTESIAN_POINT('Ctrl Pts',(-0.796034321106418,-21.8063297959755,
0.));
#10214=CARTESIAN_POINT('Ctrl Pts',(-0.796034321106418,-21.8063297959755,
21.));
#10215=CARTESIAN_POINT('Ctrl Pts',(-0.771105213258335,-21.8520856039249,
0.));
#10216=CARTESIAN_POINT('Ctrl Pts',(-0.771105213258335,-21.8520856039249,
21.));
#10217=CARTESIAN_POINT('Ctrl Pts',(-0.745927151109825,-21.8977892409997,
0.));
#10218=CARTESIAN_POINT('Ctrl Pts',(-0.745927151109825,-21.8977892409997,
21.));
#10219=CARTESIAN_POINT('Ctrl Pts',(-0.725586037496641,-21.9343103819749,
0.));
#10220=CARTESIAN_POINT('Ctrl Pts',(-0.725586037496641,-21.9343103819749,
21.));
#10221=CARTESIAN_POINT('Ctrl Pts',(-0.71021862184356,-21.9616777523685,
0.));
#10222=CARTESIAN_POINT('Ctrl Pts',(-0.71021862184356,-21.9616777523685,
21.));
#10223=CARTESIAN_POINT('Ctrl Pts',(-0.699924103234227,-21.9799122315157,
0.));
#10224=CARTESIAN_POINT('Ctrl Pts',(-0.699924103234227,-21.9799122315157,
21.));
#10225=CARTESIAN_POINT('Ctrl Pts',(-0.694764450219586,-21.9890268624765,
0.));
#10226=CARTESIAN_POINT('Ctrl Pts',(-0.694764450219586,-21.9890268624765,
21.));
#10227=CARTESIAN_POINT('Ctrl Pts',(-1.75362185428837,-18.7118598491961,
0.));
#10228=CARTESIAN_POINT('Ctrl Pts',(-1.75450132833464,-18.7212441956871,
0.));
#10229=CARTESIAN_POINT('Ctrl Pts',(-1.75601041697575,-18.7400222442427,
0.));
#10230=CARTESIAN_POINT('Ctrl Pts',(-1.75752447968136,-18.7682173836138,
0.));
#10231=CARTESIAN_POINT('Ctrl Pts',(-1.7581175236483,-18.8058650094753,0.));
#10232=CARTESIAN_POINT('Ctrl Pts',(-1.75690876962598,-18.8530026395886,
0.));
#10233=CARTESIAN_POINT('Ctrl Pts',(-1.75429229572776,-18.9002024267872,
0.));
#10234=CARTESIAN_POINT('Ctrl Pts',(-1.75080409924534,-18.947447637865,0.));
#10235=CARTESIAN_POINT('Ctrl Pts',(-1.74684309825013,-18.9947239970259,
0.));
#10236=CARTESIAN_POINT('Ctrl Pts',(-1.74256297552949,-19.0420224296189,
0.));
#10237=CARTESIAN_POINT('Ctrl Pts',(-1.73795301169841,-19.0893375576541,
0.));
#10238=CARTESIAN_POINT('Ctrl Pts',(-1.73290313712354,-19.1366665585833,
0.));
#10239=CARTESIAN_POINT('Ctrl Pts',(-1.72727220327098,-19.1840079312107,
0.));
#10240=CARTESIAN_POINT('Ctrl Pts',(-1.72096104670234,-19.2313602042899,
0.));
#10241=CARTESIAN_POINT('Ctrl Pts',(-1.71396454346262,-19.2787209722437,
0.));
#10242=CARTESIAN_POINT('Ctrl Pts',(-1.70633457265124,-19.3260873558094,
0.));
#10243=CARTESIAN_POINT('Ctrl Pts',(-1.69815571801252,-19.3734562555057,
0.));
#10244=CARTESIAN_POINT('Ctrl Pts',(-1.68951753233571,-19.4208246682917,
0.));
#10245=CARTESIAN_POINT('Ctrl Pts',(-1.68048476382294,-19.4681900187091,
0.));
#10246=CARTESIAN_POINT('Ctrl Pts',(-1.67107974760949,-19.5155503513712,
0.));
#10247=CARTESIAN_POINT('Ctrl Pts',(-1.66129908621006,-19.5629041190868,
0.));
#10248=CARTESIAN_POINT('Ctrl Pts',(-1.65112409599283,-19.6102500448855,
0.));
#10249=CARTESIAN_POINT('Ctrl Pts',(-1.64053294677822,-19.6575869645839,
0.));
#10250=CARTESIAN_POINT('Ctrl Pts',(-1.62951389038422,-19.7049136553525,
0.));
#10251=CARTESIAN_POINT('Ctrl Pts',(-1.61807191996834,-19.7522287462982,
0.));
#10252=CARTESIAN_POINT('Ctrl Pts',(-1.60622162219699,-19.7995308006834,
0.));
#10253=CARTESIAN_POINT('Ctrl Pts',(-1.59398289700559,-19.8468183626037,
0.));
#10254=CARTESIAN_POINT('Ctrl Pts',(-1.58137589158952,-19.8940900137801,
0.));
#10255=CARTESIAN_POINT('Ctrl Pts',(-1.56841542790453,-19.9413444362352,
0.));
#10256=CARTESIAN_POINT('Ctrl Pts',(-1.55510860515914,-19.9885804375096,
0.));
#10257=CARTESIAN_POINT('Ctrl Pts',(-1.54145790302918,-20.0357969106526,
0.));
#10258=CARTESIAN_POINT('Ctrl Pts',(-1.52746305716965,-20.0829928089241,
0.));
#10259=CARTESIAN_POINT('Ctrl Pts',(-1.51312326913583,-20.1301671167606,
0.));
#10260=CARTESIAN_POINT('Ctrl Pts',(-1.49843965844502,-20.1773188177942,
0.));
#10261=CARTESIAN_POINT('Ctrl Pts',(-1.48341623961914,-20.224446881308,0.));
#10262=CARTESIAN_POINT('Ctrl Pts',(-1.46805861808021,-20.2715502770004,
0.));
#10263=CARTESIAN_POINT('Ctrl Pts',(-1.45237321894404,-20.3186279833818,
0.));
#10264=CARTESIAN_POINT('Ctrl Pts',(-1.43636637152782,-20.3656789980171,
0.));
#10265=CARTESIAN_POINT('Ctrl Pts',(-1.4200432946371,-20.4127023494155,0.));
#10266=CARTESIAN_POINT('Ctrl Pts',(-1.40340771617025,-20.4596971004275,
0.));
#10267=CARTESIAN_POINT('Ctrl Pts',(-1.38646244026049,-20.5066623390132,
0.));
#10268=CARTESIAN_POINT('Ctrl Pts',(-1.36920969340018,-20.5535971721246,
0.));
#10269=CARTESIAN_POINT('Ctrl Pts',(-1.35165153211253,-20.6005007190809,
0.));
#10270=CARTESIAN_POINT('Ctrl Pts',(-1.33379029722591,-20.6473721041685,
0.));
#10271=CARTESIAN_POINT('Ctrl Pts',(-1.31562879653597,-20.694210454218,0.));
#10272=CARTESIAN_POINT('Ctrl Pts',(-1.2971700649115,-20.7410149035348,0.));
#10273=CARTESIAN_POINT('Ctrl Pts',(-1.27841722479262,-20.7877845975367,
0.));
#10274=CARTESIAN_POINT('Ctrl Pts',(-1.25937332001005,-20.83451869657,0.));
#10275=CARTESIAN_POINT('Ctrl Pts',(-1.24004113517906,-20.881216381382,0.));
#10276=CARTESIAN_POINT('Ctrl Pts',(-1.22042312071097,-20.9278768531175,
0.));
#10277=CARTESIAN_POINT('Ctrl Pts',(-1.20052150219503,-20.9744993243732,
0.));
#10278=CARTESIAN_POINT('Ctrl Pts',(-1.18033835060895,-21.0210830121673,
0.));
#10279=CARTESIAN_POINT('Ctrl Pts',(-1.15987566445808,-21.0676271313238,
0.));
#10280=CARTESIAN_POINT('Ctrl Pts',(-1.13913546246555,-21.1141308858087,
0.));
#10281=CARTESIAN_POINT('Ctrl Pts',(-1.11811982787747,-21.1605934684164,
0.));
#10282=CARTESIAN_POINT('Ctrl Pts',(-1.09683084929266,-21.2070140764156,
0.));
#10283=CARTESIAN_POINT('Ctrl Pts',(-1.07527058431887,-21.2533919248553,
0.));
#10284=CARTESIAN_POINT('Ctrl Pts',(-1.05344101900192,-21.2997262593683,
0.));
#10285=CARTESIAN_POINT('Ctrl Pts',(-1.03134402396953,-21.3460163737343,
0.));
#10286=CARTESIAN_POINT('Ctrl Pts',(-1.00898133629988,-21.3922616124166,
0.));
#10287=CARTESIAN_POINT('Ctrl Pts',(-0.986354611081139,-21.4384613333266,
0.));
#10288=CARTESIAN_POINT('Ctrl Pts',(-0.963465462815776,-21.4846148770804,
0.));
#10289=CARTESIAN_POINT('Ctrl Pts',(-0.940315509525156,-21.5307215366685,
0.));
#10290=CARTESIAN_POINT('Ctrl Pts',(-0.916906425150857,-21.5767805209408,
0.));
#10291=CARTESIAN_POINT('Ctrl Pts',(-0.893239967513677,-21.6227909401433,
0.));
#10292=CARTESIAN_POINT('Ctrl Pts',(-0.869317897714105,-21.6687518829182,
0.));
#10293=CARTESIAN_POINT('Ctrl Pts',(-0.845141916726563,-21.7146624809285,
0.));
#10294=CARTESIAN_POINT('Ctrl Pts',(-0.820713597934081,-21.7605219769118,
0.));
#10295=CARTESIAN_POINT('Ctrl Pts',(-0.796034321106418,-21.8063297959755,
0.));
#10296=CARTESIAN_POINT('Ctrl Pts',(-0.766119391688718,-21.8612367655148,
0.));
#10297=CARTESIAN_POINT('Ctrl Pts',(-0.740879090965101,-21.9069273598709,
0.));
#10298=CARTESIAN_POINT('Ctrl Pts',(-0.720488353007154,-21.9434380560096,
0.));
#10299=CARTESIAN_POINT('Ctrl Pts',(-0.705083756261763,-21.970797600548,
0.));
#10300=CARTESIAN_POINT('Ctrl Pts',(-0.694764450219586,-21.9890268624765,
0.));
#10301=CARTESIAN_POINT('Ctrl Pts',(-1.75362185428837,-18.7118598491961,
13.));
#10302=CARTESIAN_POINT('Ctrl Pts',(-1.75510417082366,-18.7276767707249,
13.));
#10303=CARTESIAN_POINT('Ctrl Pts',(-1.75615601189424,-18.743509767289,13.));
#10304=CARTESIAN_POINT('Ctrl Pts',(-1.75680608702495,-18.7593580381833,
13.));
#10305=CARTESIAN_POINT('Ctrl Pts',(-1.75756802370039,-18.7779333970397,
13.));
#10306=CARTESIAN_POINT('Ctrl Pts',(-1.75777887919059,-18.7965297250683,
13.));
#10307=CARTESIAN_POINT('Ctrl Pts',(-1.75755628860694,-18.8151436576357,
13.));
#10308=CARTESIAN_POINT('Ctrl Pts',(-1.75724309300303,-18.841334351581,13.));
#10309=CARTESIAN_POINT('Ctrl Pts',(-1.75607893899588,-18.8675597701101,
13.));
#10310=CARTESIAN_POINT('Ctrl Pts',(-1.75447363677663,-18.8938074357167,
13.));
#10311=CARTESIAN_POINT('Ctrl Pts',(-1.75340585762642,-18.9112662729005,
13.));
#10312=CARTESIAN_POINT('Ctrl Pts',(-1.75214492935969,-18.9287348768864,
13.));
#10313=CARTESIAN_POINT('Ctrl Pts',(-1.75078122387605,-18.9462100283318,
13.));
#10314=CARTESIAN_POINT('Ctrl Pts',(-1.74934570031115,-18.9646054898159,
13.));
#10315=CARTESIAN_POINT('Ctrl Pts',(-1.74779717198844,-18.9830081805071,
13.));
#10316=CARTESIAN_POINT('Ctrl Pts',(-1.74617674699282,-19.0014156957804,
13.));
#10317=CARTESIAN_POINT('Ctrl Pts',(-1.74437717633237,-19.0218582491274,
13.));
#10318=CARTESIAN_POINT('Ctrl Pts',(-1.74248762596055,-19.0423067706055,
13.));
#10319=CARTESIAN_POINT('Ctrl Pts',(-1.74049525500399,-19.0627595477289,
13.));
#10320=CARTESIAN_POINT('Ctrl Pts',(-1.73749165908531,-19.093593101938,13.));
#10321=CARTESIAN_POINT('Ctrl Pts',(-1.73424805120509,-19.1244363539499,
13.));
#10322=CARTESIAN_POINT('Ctrl Pts',(-1.73060838684927,-19.155287003772,13.));
#10323=CARTESIAN_POINT('Ctrl Pts',(-1.72796425026603,-19.177699326403,13.));
#10324=CARTESIAN_POINT('Ctrl Pts',(-1.72510779282446,-19.2001156538051,
13.));
#10325=CARTESIAN_POINT('Ctrl Pts',(-1.72201836571179,-19.2225350169884,
13.));
#10326=CARTESIAN_POINT('Ctrl Pts',(-1.71824180560906,-19.2499407687471,
13.));
#10327=CARTESIAN_POINT('Ctrl Pts',(-1.71411839343755,-19.2773510352525,
13.));
#10328=CARTESIAN_POINT('Ctrl Pts',(-1.70969587297323,-19.3047632983646,
13.));
#10329=CARTESIAN_POINT('Ctrl Pts',(-1.70491881688378,-19.3343730920291,
13.));
#10330=CARTESIAN_POINT('Ctrl Pts',(-1.69979875336634,-19.3639851445184,
13.));
#10331=CARTESIAN_POINT('Ctrl Pts',(-1.69442732753457,-19.3935962281315,
13.));
#10332=CARTESIAN_POINT('Ctrl Pts',(-1.68946845243803,-19.42093304143,13.));
#10333=CARTESIAN_POINT('Ctrl Pts',(-1.68429785630297,-19.4482690053405,
13.));
#10334=CARTESIAN_POINT('Ctrl Pts',(-1.67894398812104,-19.4756022976176,
13.));
#10335=CARTESIAN_POINT('Ctrl Pts',(-1.67167048330012,-19.512735978611,13.));
#10336=CARTESIAN_POINT('Ctrl Pts',(-1.66405675112383,-19.5498647402118,
13.));
#10337=CARTESIAN_POINT('Ctrl Pts',(-1.65607285223162,-19.5869856493823,
13.));
#10338=CARTESIAN_POINT('Ctrl Pts',(-1.64836856223834,-19.6228065249877,
13.));
#10339=CARTESIAN_POINT('Ctrl Pts',(-1.64031177032937,-19.6586201923391,
13.));
#10340=CARTESIAN_POINT('Ctrl Pts',(-1.63188637919459,-19.6944241981031,
13.));
#10341=CARTESIAN_POINT('Ctrl Pts',(-1.62044024925903,-19.7430649431597,
13.));
#10342=CARTESIAN_POINT('Ctrl Pts',(-1.60831707818776,-19.7916877990303,
13.));
#10343=CARTESIAN_POINT('Ctrl Pts',(-1.59560243914448,-19.8402857465804,
13.));
#10344=CARTESIAN_POINT('Ctrl Pts',(-1.58442654783662,-19.8830022859769,
13.));
#10345=CARTESIAN_POINT('Ctrl Pts',(-1.57280052806414,-19.9256995150004,
13.));
#10346=CARTESIAN_POINT('Ctrl Pts',(-1.56075644051379,-19.9683733417535,
13.));
#10347=CARTESIAN_POINT('Ctrl Pts',(-1.54300053140843,-20.0312849227129,
13.));
#10348=CARTESIAN_POINT('Ctrl Pts',(-1.52432694531153,-20.0941457150648,
13.));
#10349=CARTESIAN_POINT('Ctrl Pts',(-1.50474000380958,-20.1569447711145,
13.));
#10350=CARTESIAN_POINT('Ctrl Pts',(-1.48002109248255,-20.2361977927135,
13.));
#10351=CARTESIAN_POINT('Ctrl Pts',(-1.45385270859109,-20.3153523891039,
13.));
#10352=CARTESIAN_POINT('Ctrl Pts',(-1.42635858929742,-20.3943871109086,
13.));
#10353=CARTESIAN_POINT('Ctrl Pts',(-1.38911568501702,-20.5014457348841,
13.));
#10354=CARTESIAN_POINT('Ctrl Pts',(-1.34943433501594,-20.6082844520166,
13.));
#10355=CARTESIAN_POINT('Ctrl Pts',(-1.30744723531062,-20.7148563913857,
13.));
#10356=CARTESIAN_POINT('Ctrl Pts',(-1.27001463635412,-20.8098680662672,
13.));
#10357=CARTESIAN_POINT('Ctrl Pts',(-1.23075788105027,-20.9046675821832,
13.));
#10358=CARTESIAN_POINT('Ctrl Pts',(-1.18977154269178,-20.9992246142304,
13.));
#10359=CARTESIAN_POINT('Ctrl Pts',(-1.1316826302001,-21.1332379313512,13.));
#10360=CARTESIAN_POINT('Ctrl Pts',(-1.07011397706108,-21.2667633195663,
13.));
#10361=CARTESIAN_POINT('Ctrl Pts',(-1.00527632047501,-21.3997200780868,
13.));
#10362=CARTESIAN_POINT('Ctrl Pts',(-0.954911968701506,-21.5029977304476,
13.));
#10363=CARTESIAN_POINT('Ctrl Pts',(-0.902570955454164,-21.6059349895582,
13.));
#10364=CARTESIAN_POINT('Ctrl Pts',(-0.848338494601997,-21.7084903372331,
13.));
#10365=CARTESIAN_POINT('Ctrl Pts',(-0.801423317792771,-21.7972084627486,
13.));
#10366=CARTESIAN_POINT('Ctrl Pts',(-0.753096147909189,-21.8856382928766,
13.));
#10367=CARTESIAN_POINT('Ctrl Pts',(-0.703383282402061,-21.9737740855816,
13.));
#10368=CARTESIAN_POINT('Ctrl Pts',(-0.700514964339855,-21.9788593182183,
13.));
#10369=CARTESIAN_POINT('Ctrl Pts',(-0.697642020192887,-21.9839435771672,
13.));
#10370=CARTESIAN_POINT('Ctrl Pts',(-0.694764450219586,-21.9890268624765,
13.));
#10371=CARTESIAN_POINT('Ctrl Pts',(-6.13422273260091,-21.1275013067528,
0.));
#10372=CARTESIAN_POINT('Ctrl Pts',(-6.13422273260091,-21.1275013067528,
21.));
#10373=CARTESIAN_POINT('Ctrl Pts',(-6.12649903511518,-21.1204271980506,
0.));
#10374=CARTESIAN_POINT('Ctrl Pts',(-6.12649903511518,-21.1204271980506,
21.));
#10375=CARTESIAN_POINT('Ctrl Pts',(-6.11107360216958,-21.1062663590356,
0.));
#10376=CARTESIAN_POINT('Ctrl Pts',(-6.11107360216958,-21.1062663590356,
21.));
#10377=CARTESIAN_POINT('Ctrl Pts',(-6.08800133883115,-21.0849872356853,
0.));
#10378=CARTESIAN_POINT('Ctrl Pts',(-6.08800133883115,-21.0849872356853,
21.));
#10379=CARTESIAN_POINT('Ctrl Pts',(-6.05737013696533,-21.0565393163693,
0.));
#10380=CARTESIAN_POINT('Ctrl Pts',(-6.05737013696533,-21.0565393163693,
21.));
#10381=CARTESIAN_POINT('Ctrl Pts',(-6.01930117633045,-21.0208530236003,
0.));
#10382=CARTESIAN_POINT('Ctrl Pts',(-6.01930117633045,-21.0208530236003,
21.));
#10383=CARTESIAN_POINT('Ctrl Pts',(-5.98145286361837,-20.9850401822713,
0.));
#10384=CARTESIAN_POINT('Ctrl Pts',(-5.98145286361837,-20.9850401822713,
21.));
#10385=CARTESIAN_POINT('Ctrl Pts',(-5.94382608200804,-20.9491006734021,
0.));
#10386=CARTESIAN_POINT('Ctrl Pts',(-5.94382608200804,-20.9491006734021,
21.));
#10387=CARTESIAN_POINT('Ctrl Pts',(-5.906422006626,-20.9130344665641,0.));
#10388=CARTESIAN_POINT('Ctrl Pts',(-5.906422006626,-20.9130344665641,21.));
#10389=CARTESIAN_POINT('Ctrl Pts',(-5.86924212736288,-20.8768416821402,
0.));
#10390=CARTESIAN_POINT('Ctrl Pts',(-5.86924212736288,-20.8768416821402,
21.));
#10391=CARTESIAN_POINT('Ctrl Pts',(-5.83228817460178,-20.8405225541277,
0.));
#10392=CARTESIAN_POINT('Ctrl Pts',(-5.83228817460178,-20.8405225541277,
21.));
#10393=CARTESIAN_POINT('Ctrl Pts',(-5.79556203439644,-20.8040773827343,
0.));
#10394=CARTESIAN_POINT('Ctrl Pts',(-5.79556203439644,-20.8040773827343,
21.));
#10395=CARTESIAN_POINT('Ctrl Pts',(-5.75906566327796,-20.7675064905026,
0.));
#10396=CARTESIAN_POINT('Ctrl Pts',(-5.75906566327796,-20.7675064905026,
21.));
#10397=CARTESIAN_POINT('Ctrl Pts',(-5.72280100798241,-20.7308101804425,
0.));
#10398=CARTESIAN_POINT('Ctrl Pts',(-5.72280100798241,-20.7308101804425,
21.));
#10399=CARTESIAN_POINT('Ctrl Pts',(-5.68676990500164,-20.6939886877061,
0.));
#10400=CARTESIAN_POINT('Ctrl Pts',(-5.68676990500164,-20.6939886877061,
21.));
#10401=CARTESIAN_POINT('Ctrl Pts',(-5.65097411164335,-20.6570421847033,
0.));
#10402=CARTESIAN_POINT('Ctrl Pts',(-5.65097411164335,-20.6570421847033,
21.));
#10403=CARTESIAN_POINT('Ctrl Pts',(-5.6154153671515,-20.6199707996366,0.));
#10404=CARTESIAN_POINT('Ctrl Pts',(-5.6154153671515,-20.6199707996366,21.));
#10405=CARTESIAN_POINT('Ctrl Pts',(-5.58009544402475,-20.5827746317185,
0.));
#10406=CARTESIAN_POINT('Ctrl Pts',(-5.58009544402475,-20.5827746317185,
21.));
#10407=CARTESIAN_POINT('Ctrl Pts',(-5.5450161968946,-20.5454537676144,0.));
#10408=CARTESIAN_POINT('Ctrl Pts',(-5.5450161968946,-20.5454537676144,21.));
#10409=CARTESIAN_POINT('Ctrl Pts',(-5.51017962306782,-20.5080083009242,
0.));
#10410=CARTESIAN_POINT('Ctrl Pts',(-5.51017962306782,-20.5080083009242,
21.));
#10411=CARTESIAN_POINT('Ctrl Pts',(-5.47558784449851,-20.4704383353718,
0.));
#10412=CARTESIAN_POINT('Ctrl Pts',(-5.47558784449851,-20.4704383353718,
21.));
#10413=CARTESIAN_POINT('Ctrl Pts',(-5.44124306065111,-20.4327439816542,
0.));
#10414=CARTESIAN_POINT('Ctrl Pts',(-5.44124306065111,-20.4327439816542,
21.));
#10415=CARTESIAN_POINT('Ctrl Pts',(-5.40714750595875,-20.3949253578015,
0.));
#10416=CARTESIAN_POINT('Ctrl Pts',(-5.40714750595875,-20.3949253578015,
21.));
#10417=CARTESIAN_POINT('Ctrl Pts',(-5.37330341114649,-20.3569825877537,
0.));
#10418=CARTESIAN_POINT('Ctrl Pts',(-5.37330341114649,-20.3569825877537,
21.));
#10419=CARTESIAN_POINT('Ctrl Pts',(-5.33971294212214,-20.3189158047642,
0.));
#10420=CARTESIAN_POINT('Ctrl Pts',(-5.33971294212214,-20.3189158047642,
21.));
#10421=CARTESIAN_POINT('Ctrl Pts',(-5.30637824220998,-20.2807251380077,
0.));
#10422=CARTESIAN_POINT('Ctrl Pts',(-5.30637824220998,-20.2807251380077,
21.));
#10423=CARTESIAN_POINT('Ctrl Pts',(-5.27330152298151,-20.2424106921768,
0.));
#10424=CARTESIAN_POINT('Ctrl Pts',(-5.27330152298151,-20.2424106921768,
21.));
#10425=CARTESIAN_POINT('Ctrl Pts',(-5.24048514441891,-20.2039725283917,
0.));
#10426=CARTESIAN_POINT('Ctrl Pts',(-5.24048514441891,-20.2039725283917,
21.));
#10427=CARTESIAN_POINT('Ctrl Pts',(-5.20793168386164,-20.1654106491899,
0.));
#10428=CARTESIAN_POINT('Ctrl Pts',(-5.20793168386164,-20.1654106491899,
21.));
#10429=CARTESIAN_POINT('Ctrl Pts',(-5.17564404279922,-20.1267249732337,
0.));
#10430=CARTESIAN_POINT('Ctrl Pts',(-5.17564404279922,-20.1267249732337,
21.));
#10431=CARTESIAN_POINT('Ctrl Pts',(-5.14362537555398,-20.087915358486,0.));
#10432=CARTESIAN_POINT('Ctrl Pts',(-5.14362537555398,-20.087915358486,21.));
#10433=CARTESIAN_POINT('Ctrl Pts',(-5.11187891582335,-20.0489816528155,
0.));
#10434=CARTESIAN_POINT('Ctrl Pts',(-5.11187891582335,-20.0489816528155,
21.));
#10435=CARTESIAN_POINT('Ctrl Pts',(-5.08040781745337,-20.0099237417205,
0.));
#10436=CARTESIAN_POINT('Ctrl Pts',(-5.08040781745337,-20.0099237417205,
21.));
#10437=CARTESIAN_POINT('Ctrl Pts',(-5.04921502064063,-19.9707415879783,
0.));
#10438=CARTESIAN_POINT('Ctrl Pts',(-5.04921502064063,-19.9707415879783,
21.));
#10439=CARTESIAN_POINT('Ctrl Pts',(-5.01830302225558,-19.931435301086,0.));
#10440=CARTESIAN_POINT('Ctrl Pts',(-5.01830302225558,-19.931435301086,21.));
#10441=CARTESIAN_POINT('Ctrl Pts',(-4.98767405031333,-19.8920050831202,
0.));
#10442=CARTESIAN_POINT('Ctrl Pts',(-4.98767405031333,-19.8920050831202,
21.));
#10443=CARTESIAN_POINT('Ctrl Pts',(-4.95733049830096,-19.8524510953961,
0.));
#10444=CARTESIAN_POINT('Ctrl Pts',(-4.95733049830096,-19.8524510953961,
21.));
#10445=CARTESIAN_POINT('Ctrl Pts',(-4.92727531494347,-19.8127733387903,
0.));
#10446=CARTESIAN_POINT('Ctrl Pts',(-4.92727531494347,-19.8127733387903,
21.));
#10447=CARTESIAN_POINT('Ctrl Pts',(-4.89751233527805,-19.772971552601,0.));
#10448=CARTESIAN_POINT('Ctrl Pts',(-4.89751233527805,-19.772971552601,21.));
#10449=CARTESIAN_POINT('Ctrl Pts',(-4.86804682289087,-19.7330450480715,
0.));
#10450=CARTESIAN_POINT('Ctrl Pts',(-4.86804682289087,-19.7330450480715,
21.));
#10451=CARTESIAN_POINT('Ctrl Pts',(-4.83888510708974,-19.6929928227072,
0.));
#10452=CARTESIAN_POINT('Ctrl Pts',(-4.83888510708974,-19.6929928227072,
21.));
#10453=CARTESIAN_POINT('Ctrl Pts',(-4.81003361418061,-19.6528138625329,
0.));
#10454=CARTESIAN_POINT('Ctrl Pts',(-4.81003361418061,-19.6528138625329,
21.));
#10455=CARTESIAN_POINT('Ctrl Pts',(-4.78149799361731,-19.6125074152527,
0.));
#10456=CARTESIAN_POINT('Ctrl Pts',(-4.78149799361731,-19.6125074152527,
21.));
#10457=CARTESIAN_POINT('Ctrl Pts',(-4.75328238194611,-19.5720732205813,
0.));
#10458=CARTESIAN_POINT('Ctrl Pts',(-4.75328238194611,-19.5720732205813,
21.));
#10459=CARTESIAN_POINT('Ctrl Pts',(-4.72538815796616,-19.531511899192,0.));
#10460=CARTESIAN_POINT('Ctrl Pts',(-4.72538815796616,-19.531511899192,21.));
#10461=CARTESIAN_POINT('Ctrl Pts',(-4.69781487613785,-19.4908246636763,
0.));
#10462=CARTESIAN_POINT('Ctrl Pts',(-4.69781487613785,-19.4908246636763,
21.));
#10463=CARTESIAN_POINT('Ctrl Pts',(-4.67056260851454,-19.4500125912299,
0.));
#10464=CARTESIAN_POINT('Ctrl Pts',(-4.67056260851454,-19.4500125912299,
21.));
#10465=CARTESIAN_POINT('Ctrl Pts',(-4.64363405547472,-19.4090759683639,
0.));
#10466=CARTESIAN_POINT('Ctrl Pts',(-4.64363405547472,-19.4090759683639,
21.));
#10467=CARTESIAN_POINT('Ctrl Pts',(-4.61703633725712,-19.3680137353983,
0.));
#10468=CARTESIAN_POINT('Ctrl Pts',(-4.61703633725712,-19.3680137353983,
21.));
#10469=CARTESIAN_POINT('Ctrl Pts',(-4.59078395765677,-19.3268225655679,
0.));
#10470=CARTESIAN_POINT('Ctrl Pts',(-4.59078395765677,-19.3268225655679,
21.));
#10471=CARTESIAN_POINT('Ctrl Pts',(-4.56489651606741,-19.2854975819105,
0.));
#10472=CARTESIAN_POINT('Ctrl Pts',(-4.56489651606741,-19.2854975819105,
21.));
#10473=CARTESIAN_POINT('Ctrl Pts',(-4.53939338835152,-19.2440340196551,
0.));
#10474=CARTESIAN_POINT('Ctrl Pts',(-4.53939338835152,-19.2440340196551,
21.));
#10475=CARTESIAN_POINT('Ctrl Pts',(-4.51428889122955,-19.2024287376926,
0.));
#10476=CARTESIAN_POINT('Ctrl Pts',(-4.51428889122955,-19.2024287376926,
21.));
#10477=CARTESIAN_POINT('Ctrl Pts',(-4.48958819710577,-19.1606814968494,
0.));
#10478=CARTESIAN_POINT('Ctrl Pts',(-4.48958819710577,-19.1606814968494,
21.));
#10479=CARTESIAN_POINT('Ctrl Pts',(-4.46528051067022,-19.1187970904932,
0.));
#10480=CARTESIAN_POINT('Ctrl Pts',(-4.46528051067022,-19.1187970904932,
21.));
#10481=CARTESIAN_POINT('Ctrl Pts',(-4.44134542994082,-19.0767833717249,
0.));
#10482=CARTESIAN_POINT('Ctrl Pts',(-4.44134542994082,-19.0767833717249,
21.));
#10483=CARTESIAN_POINT('Ctrl Pts',(-4.41776558033332,-19.034647328575,0.));
#10484=CARTESIAN_POINT('Ctrl Pts',(-4.41776558033332,-19.034647328575,21.));
#10485=CARTESIAN_POINT('Ctrl Pts',(-4.39453820875555,-18.9923914823906,
0.));
#10486=CARTESIAN_POINT('Ctrl Pts',(-4.39453820875555,-18.9923914823906,
21.));
#10487=CARTESIAN_POINT('Ctrl Pts',(-4.37168516143123,-18.9500107909187,
0.));
#10488=CARTESIAN_POINT('Ctrl Pts',(-4.37168516143123,-18.9500107909187,
21.));
#10489=CARTESIAN_POINT('Ctrl Pts',(-4.34926881342022,-18.9074876952706,
0.));
#10490=CARTESIAN_POINT('Ctrl Pts',(-4.34926881342022,-18.9074876952706,
21.));
#10491=CARTESIAN_POINT('Ctrl Pts',(-4.32737526247704,-18.8647973781745,
0.));
#10492=CARTESIAN_POINT('Ctrl Pts',(-4.32737526247704,-18.8647973781745,
21.));
#10493=CARTESIAN_POINT('Ctrl Pts',(-4.30608591031526,-18.8219166495975,
0.));
#10494=CARTESIAN_POINT('Ctrl Pts',(-4.30608591031526,-18.8219166495975,
21.));
#10495=CARTESIAN_POINT('Ctrl Pts',(-4.28545098663153,-18.778832216358,0.));
#10496=CARTESIAN_POINT('Ctrl Pts',(-4.28545098663153,-18.778832216358,21.));
#10497=CARTESIAN_POINT('Ctrl Pts',(-4.26546636161933,-18.735547949685,0.));
#10498=CARTESIAN_POINT('Ctrl Pts',(-4.26546636161933,-18.735547949685,21.));
#10499=CARTESIAN_POINT('Ctrl Pts',(-4.24603817988453,-18.6920958920047,
0.));
#10500=CARTESIAN_POINT('Ctrl Pts',(-4.24603817988453,-18.6920958920047,
21.));
#10501=CARTESIAN_POINT('Ctrl Pts',(-4.22703266508919,-18.6485210883348,
0.));
#10502=CARTESIAN_POINT('Ctrl Pts',(-4.22703266508919,-18.6485210883348,
21.));
#10503=CARTESIAN_POINT('Ctrl Pts',(-4.20834600700665,-18.6048602364653,
0.));
#10504=CARTESIAN_POINT('Ctrl Pts',(-4.20834600700665,-18.6048602364653,
21.));
#10505=CARTESIAN_POINT('Ctrl Pts',(-4.18996967278621,-18.5611217636409,
0.));
#10506=CARTESIAN_POINT('Ctrl Pts',(-4.18996967278621,-18.5611217636409,
21.));
#10507=CARTESIAN_POINT('Ctrl Pts',(-4.17205262766562,-18.5172668097744,
0.));
#10508=CARTESIAN_POINT('Ctrl Pts',(-4.17205262766562,-18.5172668097744,
21.));
#10509=CARTESIAN_POINT('Ctrl Pts',(-4.15497867673974,-18.4731856794913,
0.));
#10510=CARTESIAN_POINT('Ctrl Pts',(-4.15497867673974,-18.4731856794913,
21.));
#10511=CARTESIAN_POINT('Ctrl Pts',(-4.13926275457062,-18.4287286547442,
0.));
#10512=CARTESIAN_POINT('Ctrl Pts',(-4.13926275457062,-18.4287286547442,
21.));
#10513=CARTESIAN_POINT('Ctrl Pts',(-4.12819301671079,-18.3927403741815,
0.));
#10514=CARTESIAN_POINT('Ctrl Pts',(-4.12819301671079,-18.3927403741815,
21.));
#10515=CARTESIAN_POINT('Ctrl Pts',(-4.1209201986886,-18.3654573320481,0.));
#10516=CARTESIAN_POINT('Ctrl Pts',(-4.1209201986886,-18.3654573320481,21.));
#10517=CARTESIAN_POINT('Ctrl Pts',(-4.11655269114952,-18.3471320125699,
0.));
#10518=CARTESIAN_POINT('Ctrl Pts',(-4.11655269114952,-18.3471320125699,
21.));
#10519=CARTESIAN_POINT('Ctrl Pts',(-4.11448919812531,-18.337935196262,0.));
#10520=CARTESIAN_POINT('Ctrl Pts',(-4.11448919812531,-18.337935196262,21.));
#10521=CARTESIAN_POINT('',(-6.13422273260085,-21.1275013067528,0.));
#10522=CARTESIAN_POINT('Ctrl Pts',(-4.11448919812531,-18.337935196262,0.));
#10523=CARTESIAN_POINT('Ctrl Pts',(-4.11655269114952,-18.3471320125699,
0.));
#10524=CARTESIAN_POINT('Ctrl Pts',(-4.1209201986886,-18.3654573320481,0.));
#10525=CARTESIAN_POINT('Ctrl Pts',(-4.12819301671079,-18.3927403741815,
0.));
#10526=CARTESIAN_POINT('Ctrl Pts',(-4.13926275457062,-18.4287286547442,
0.));
#10527=CARTESIAN_POINT('Ctrl Pts',(-4.15497867673974,-18.4731856794913,
0.));
#10528=CARTESIAN_POINT('Ctrl Pts',(-4.17205262766562,-18.5172668097744,
0.));
#10529=CARTESIAN_POINT('Ctrl Pts',(-4.18996967278621,-18.5611217636409,
0.));
#10530=CARTESIAN_POINT('Ctrl Pts',(-4.20834600700665,-18.6048602364653,
0.));
#10531=CARTESIAN_POINT('Ctrl Pts',(-4.22703266508919,-18.6485210883348,
0.));
#10532=CARTESIAN_POINT('Ctrl Pts',(-4.24603817988453,-18.6920958920047,
0.));
#10533=CARTESIAN_POINT('Ctrl Pts',(-4.26546636161933,-18.735547949685,0.));
#10534=CARTESIAN_POINT('Ctrl Pts',(-4.28545098663153,-18.778832216358,0.));
#10535=CARTESIAN_POINT('Ctrl Pts',(-4.30608591031526,-18.8219166495975,
0.));
#10536=CARTESIAN_POINT('Ctrl Pts',(-4.32737526247704,-18.8647973781745,
0.));
#10537=CARTESIAN_POINT('Ctrl Pts',(-4.34926881342022,-18.9074876952706,
0.));
#10538=CARTESIAN_POINT('Ctrl Pts',(-4.37168516143123,-18.9500107909187,
0.));
#10539=CARTESIAN_POINT('Ctrl Pts',(-4.39453820875555,-18.9923914823906,
0.));
#10540=CARTESIAN_POINT('Ctrl Pts',(-4.41776558033332,-19.034647328575,0.));
#10541=CARTESIAN_POINT('Ctrl Pts',(-4.44134542994082,-19.0767833717249,
0.));
#10542=CARTESIAN_POINT('Ctrl Pts',(-4.46528051067022,-19.1187970904932,
0.));
#10543=CARTESIAN_POINT('Ctrl Pts',(-4.48958819710577,-19.1606814968494,
0.));
#10544=CARTESIAN_POINT('Ctrl Pts',(-4.51428889122955,-19.2024287376926,
0.));
#10545=CARTESIAN_POINT('Ctrl Pts',(-4.53939338835152,-19.2440340196551,
0.));
#10546=CARTESIAN_POINT('Ctrl Pts',(-4.56489651606741,-19.2854975819105,
0.));
#10547=CARTESIAN_POINT('Ctrl Pts',(-4.59078395765677,-19.3268225655679,
0.));
#10548=CARTESIAN_POINT('Ctrl Pts',(-4.61703633725712,-19.3680137353983,
0.));
#10549=CARTESIAN_POINT('Ctrl Pts',(-4.64363405547472,-19.4090759683639,
0.));
#10550=CARTESIAN_POINT('Ctrl Pts',(-4.67056260851454,-19.4500125912299,
0.));
#10551=CARTESIAN_POINT('Ctrl Pts',(-4.69781487613785,-19.4908246636763,
0.));
#10552=CARTESIAN_POINT('Ctrl Pts',(-4.72538815796616,-19.531511899192,0.));
#10553=CARTESIAN_POINT('Ctrl Pts',(-4.75328238194611,-19.5720732205813,
0.));
#10554=CARTESIAN_POINT('Ctrl Pts',(-4.78149799361731,-19.6125074152527,
0.));
#10555=CARTESIAN_POINT('Ctrl Pts',(-4.81003361418061,-19.6528138625329,
0.));
#10556=CARTESIAN_POINT('Ctrl Pts',(-4.83888510708974,-19.6929928227072,
0.));
#10557=CARTESIAN_POINT('Ctrl Pts',(-4.86804682289087,-19.7330450480715,
0.));
#10558=CARTESIAN_POINT('Ctrl Pts',(-4.89751233527805,-19.772971552601,0.));
#10559=CARTESIAN_POINT('Ctrl Pts',(-4.92727531494347,-19.8127733387903,
0.));
#10560=CARTESIAN_POINT('Ctrl Pts',(-4.95733049830096,-19.8524510953961,
0.));
#10561=CARTESIAN_POINT('Ctrl Pts',(-4.98767405031333,-19.8920050831202,
0.));
#10562=CARTESIAN_POINT('Ctrl Pts',(-5.01830302225558,-19.931435301086,0.));
#10563=CARTESIAN_POINT('Ctrl Pts',(-5.04921502064063,-19.9707415879783,
0.));
#10564=CARTESIAN_POINT('Ctrl Pts',(-5.08040781745337,-20.0099237417205,
0.));
#10565=CARTESIAN_POINT('Ctrl Pts',(-5.11187891582335,-20.0489816528155,
0.));
#10566=CARTESIAN_POINT('Ctrl Pts',(-5.14362537555398,-20.087915358486,0.));
#10567=CARTESIAN_POINT('Ctrl Pts',(-5.17564404279922,-20.1267249732337,
0.));
#10568=CARTESIAN_POINT('Ctrl Pts',(-5.20793168386164,-20.1654106491899,
0.));
#10569=CARTESIAN_POINT('Ctrl Pts',(-5.24048514441891,-20.2039725283917,
0.));
#10570=CARTESIAN_POINT('Ctrl Pts',(-5.27330152298151,-20.2424106921768,
0.));
#10571=CARTESIAN_POINT('Ctrl Pts',(-5.30637824220998,-20.2807251380077,
0.));
#10572=CARTESIAN_POINT('Ctrl Pts',(-5.33971294212214,-20.3189158047642,
0.));
#10573=CARTESIAN_POINT('Ctrl Pts',(-5.37330341114649,-20.3569825877537,
0.));
#10574=CARTESIAN_POINT('Ctrl Pts',(-5.40714750595875,-20.3949253578015,
0.));
#10575=CARTESIAN_POINT('Ctrl Pts',(-5.44124306065111,-20.4327439816542,
0.));
#10576=CARTESIAN_POINT('Ctrl Pts',(-5.47558784449851,-20.4704383353718,
0.));
#10577=CARTESIAN_POINT('Ctrl Pts',(-5.51017962306782,-20.5080083009242,
0.));
#10578=CARTESIAN_POINT('Ctrl Pts',(-5.5450161968946,-20.5454537676144,0.));
#10579=CARTESIAN_POINT('Ctrl Pts',(-5.58009544402475,-20.5827746317185,
0.));
#10580=CARTESIAN_POINT('Ctrl Pts',(-5.6154153671515,-20.6199707996366,0.));
#10581=CARTESIAN_POINT('Ctrl Pts',(-5.65097411164335,-20.6570421847033,
0.));
#10582=CARTESIAN_POINT('Ctrl Pts',(-5.68676990500164,-20.6939886877061,
0.));
#10583=CARTESIAN_POINT('Ctrl Pts',(-5.72280100798241,-20.7308101804425,
0.));
#10584=CARTESIAN_POINT('Ctrl Pts',(-5.75906566327796,-20.7675064905026,
0.));
#10585=CARTESIAN_POINT('Ctrl Pts',(-5.79556203439644,-20.8040773827343,
0.));
#10586=CARTESIAN_POINT('Ctrl Pts',(-5.83228817460178,-20.8405225541277,
0.));
#10587=CARTESIAN_POINT('Ctrl Pts',(-5.86924212736288,-20.8768416821402,
0.));
#10588=CARTESIAN_POINT('Ctrl Pts',(-5.906422006626,-20.9130344665641,0.));
#10589=CARTESIAN_POINT('Ctrl Pts',(-5.94382608200804,-20.9491006734021,
0.));
#10590=CARTESIAN_POINT('Ctrl Pts',(-5.98145286361837,-20.9850401822713,
0.));
#10591=CARTESIAN_POINT('Ctrl Pts',(-6.02687083887287,-21.0280155918661,
0.));
#10592=CARTESIAN_POINT('Ctrl Pts',(-6.06499496148845,-21.0636702474951,
0.));
#10593=CARTESIAN_POINT('Ctrl Pts',(-6.09567013127872,-21.0920928984154,
0.));
#10594=CARTESIAN_POINT('Ctrl Pts',(-6.11877533761501,-21.1133530893457,
0.));
#10595=CARTESIAN_POINT('Ctrl Pts',(-6.13422273260091,-21.1275013067528,
0.));
#10596=CARTESIAN_POINT('',(-6.13422273260085,-21.1275013067528,13.));
#10597=CARTESIAN_POINT('Ctrl Pts',(-6.13422273260091,-21.1275013067528,
13.));
#10598=CARTESIAN_POINT('Ctrl Pts',(-6.05818207473574,-21.0578559224639,
13.));
#10599=CARTESIAN_POINT('Ctrl Pts',(-5.98341417184727,-20.9874765040291,
13.));
#10600=CARTESIAN_POINT('Ctrl Pts',(-5.90994468705572,-20.91635991547,13.));
#10601=CARTESIAN_POINT('Ctrl Pts',(-5.78820256793373,-20.7985166473367,
13.));
#10602=CARTESIAN_POINT('Ctrl Pts',(-5.67003811891004,-20.6786545089329,
13.));
#10603=CARTESIAN_POINT('Ctrl Pts',(-5.55573863837939,-20.5568062999927,
13.));
#10604=CARTESIAN_POINT('Ctrl Pts',(-5.46788135574845,-20.4631466220902,
13.));
#10605=CARTESIAN_POINT('Ctrl Pts',(-5.38230707224949,-20.3683108766313,
13.));
#10606=CARTESIAN_POINT('Ctrl Pts',(-5.29917141503086,-20.272307558011,13.));
#10607=CARTESIAN_POINT('Ctrl Pts',(-5.20967788549041,-20.1689623013743,
13.));
#10608=CARTESIAN_POINT('Ctrl Pts',(-5.12300396000483,-20.0642651120126,
13.));
#10609=CARTESIAN_POINT('Ctrl Pts',(-5.03941267542058,-19.9582092065757,
13.));
#10610=CARTESIAN_POINT('Ctrl Pts',(-4.99313426716769,-19.8994937733358,
13.));
#10611=CARTESIAN_POINT('Ctrl Pts',(-4.9477958395688,-19.8403635603379,13.));
#10612=CARTESIAN_POINT('Ctrl Pts',(-4.90344584463339,-19.780817320786,13.));
#10613=CARTESIAN_POINT('Ctrl Pts',(-4.86070845370395,-19.72343623378,13.));
#10614=CARTESIAN_POINT('Ctrl Pts',(-4.81889538674849,-19.665666793385,13.));
#10615=CARTESIAN_POINT('Ctrl Pts',(-4.7780829655059,-19.607498635726,13.));
#10616=CARTESIAN_POINT('Ctrl Pts',(-4.74280851477666,-19.5572235050457,
13.));
#10617=CARTESIAN_POINT('Ctrl Pts',(-4.70827845306304,-19.5066514991033,
13.));
#10618=CARTESIAN_POINT('Ctrl Pts',(-4.67449772148844,-19.4557905173051,
13.));
#10619=CARTESIAN_POINT('Ctrl Pts',(-4.65025481897416,-19.4192898920658,
13.));
#10620=CARTESIAN_POINT('Ctrl Pts',(-4.62639514838843,-19.382641288743,13.));
#10621=CARTESIAN_POINT('Ctrl Pts',(-4.60295743063937,-19.3458364383459,
13.));
#10622=CARTESIAN_POINT('Ctrl Pts',(-4.57990136645455,-19.309630908347,13.));
#10623=CARTESIAN_POINT('Ctrl Pts',(-4.55725971984417,-19.273272273525,13.));
#10624=CARTESIAN_POINT('Ctrl Pts',(-4.5350835755811,-19.2367485575731,13.));
#10625=CARTESIAN_POINT('Ctrl Pts',(-4.51585555580649,-19.2050803503215,
13.));
#10626=CARTESIAN_POINT('Ctrl Pts',(-4.49697986255775,-19.1732873013029,
13.));
#10627=CARTESIAN_POINT('Ctrl Pts',(-4.47844262265296,-19.1413765621579,
13.));
#10628=CARTESIAN_POINT('Ctrl Pts',(-4.46165213670422,-19.1124727544724,
13.));
#10629=CARTESIAN_POINT('Ctrl Pts',(-4.4451340112905,-19.0834740456903,13.));
#10630=CARTESIAN_POINT('Ctrl Pts',(-4.42886646472448,-19.0543895552964,
13.));
#10631=CARTESIAN_POINT('Ctrl Pts',(-4.41516354268672,-19.0298903167199,
13.));
#10632=CARTESIAN_POINT('Ctrl Pts',(-4.40163676089501,-19.0053307306813,
13.));
#10633=CARTESIAN_POINT('Ctrl Pts',(-4.38830551710826,-18.9807063064772,
13.));
#10634=CARTESIAN_POINT('Ctrl Pts',(-4.36901375649227,-18.9450720847457,
13.));
#10635=CARTESIAN_POINT('Ctrl Pts',(-4.35013223002823,-18.9093017976319,
13.));
#10636=CARTESIAN_POINT('Ctrl Pts',(-4.33187128669082,-18.8733353264261,
13.));
#10637=CARTESIAN_POINT('Ctrl Pts',(-4.32083731653844,-18.8516029896876,
13.));
#10638=CARTESIAN_POINT('Ctrl Pts',(-4.31003325584325,-18.829798004179,13.));
#10639=CARTESIAN_POINT('Ctrl Pts',(-4.29948469303248,-18.807913802916,13.));
#10640=CARTESIAN_POINT('Ctrl Pts',(-4.28975595059153,-18.787730412872,13.));
#10641=CARTESIAN_POINT('Ctrl Pts',(-4.28024580001115,-18.7674792481688,
13.));
#10642=CARTESIAN_POINT('Ctrl Pts',(-4.27093067976999,-18.7471689057697,
13.));
#10643=CARTESIAN_POINT('Ctrl Pts',(-4.25811678809167,-18.7192299720025,
13.));
#10644=CARTESIAN_POINT('Ctrl Pts',(-4.24566493398932,-18.6911811213678,
13.));
#10645=CARTESIAN_POINT('Ctrl Pts',(-4.23343245343576,-18.6630711735883,
13.));
#10646=CARTESIAN_POINT('Ctrl Pts',(-4.22567194943,-18.6452377209709,13.));
#10647=CARTESIAN_POINT('Ctrl Pts',(-4.21799814921869,-18.6273802008519,
13.));
#10648=CARTESIAN_POINT('Ctrl Pts',(-4.21040342108815,-18.6095026819575,
13.));
#10649=CARTESIAN_POINT('Ctrl Pts',(-4.2035875060976,-18.5934584408824,13.));
#10650=CARTESIAN_POINT('Ctrl Pts',(-4.1968345819819,-18.5773983085029,13.));
#10651=CARTESIAN_POINT('Ctrl Pts',(-4.19017810368168,-18.5613135378487,
13.));
#10652=CARTESIAN_POINT('Ctrl Pts',(-4.18318081927935,-18.5444052404372,
13.));
#10653=CARTESIAN_POINT('Ctrl Pts',(-4.17628995976621,-18.5274697699669,
13.));
#10654=CARTESIAN_POINT('Ctrl Pts',(-4.16960404102653,-18.5104789585687,
13.));
#10655=CARTESIAN_POINT('Ctrl Pts',(-4.15849874475977,-18.4822572583451,
13.));
#10656=CARTESIAN_POINT('Ctrl Pts',(-4.14796697295268,-18.4538805850219,
13.));
#10657=CARTESIAN_POINT('Ctrl Pts',(-4.13860964460765,-18.4251735640106,
13.));
#10658=CARTESIAN_POINT('Ctrl Pts',(-4.13344968074392,-18.4093434909821,
13.));
#10659=CARTESIAN_POINT('Ctrl Pts',(-4.12864814562055,-18.3934125378936,
13.));
#10660=CARTESIAN_POINT('Ctrl Pts',(-4.1242788981144,-18.3773590065616,13.));
#10661=CARTESIAN_POINT('Ctrl Pts',(-4.1207247406093,-18.3643002867737,13.));
#10662=CARTESIAN_POINT('Ctrl Pts',(-4.11745655843684,-18.3511604736845,
13.));
#10663=CARTESIAN_POINT('Ctrl Pts',(-4.11448919812531,-18.337935196262,13.));
#10664=CARTESIAN_POINT('',(-6.13422273260085,-21.1275013067528,0.));
#10665=CARTESIAN_POINT('Origin',(-1.75106900012182E-12,-5.38923623413286E-12,
0.));
#10666=CARTESIAN_POINT('',(-7.45574324794401,-20.698113262342,0.));
#10667=CARTESIAN_POINT('Origin',(-1.75106900012182E-12,-5.38923623413286E-12,
0.));
#10668=CARTESIAN_POINT('',(-7.45574324794401,-20.698113262342,13.));
#10669=CARTESIAN_POINT('Origin',(-1.75106900012182E-12,-5.38923623413286E-12,
13.));
#10670=CARTESIAN_POINT('',(-7.45574324794401,-20.698113262342,0.));
#10671=CARTESIAN_POINT('Ctrl Pts',(-7.45007618140239,-17.2541372868972,
0.));
#10672=CARTESIAN_POINT('Ctrl Pts',(-7.45007618140239,-17.2541372868972,
21.));
#10673=CARTESIAN_POINT('Ctrl Pts',(-7.45381253347183,-17.2627905583523,
0.));
#10674=CARTESIAN_POINT('Ctrl Pts',(-7.45381253347183,-17.2627905583523,
21.));
#10675=CARTESIAN_POINT('Ctrl Pts',(-7.46105049818251,-17.2801832097582,
0.));
#10676=CARTESIAN_POINT('Ctrl Pts',(-7.46105049818251,-17.2801832097582,
21.));
#10677=CARTESIAN_POINT('Ctrl Pts',(-7.4712032346092,-17.3065305096784,0.));
#10678=CARTESIAN_POINT('Ctrl Pts',(-7.4712032346092,-17.3065305096784,21.));
#10679=CARTESIAN_POINT('Ctrl Pts',(-7.48340100912745,-17.3421522689127,
0.));
#10680=CARTESIAN_POINT('Ctrl Pts',(-7.48340100912745,-17.3421522689127,
21.));
#10681=CARTESIAN_POINT('Ctrl Pts',(-7.49681774451751,-17.3873563447297,
0.));
#10682=CARTESIAN_POINT('Ctrl Pts',(-7.49681774451751,-17.3873563447297,
21.));
#10683=CARTESIAN_POINT('Ctrl Pts',(-7.50891486634214,-17.4330545448126,
0.));
#10684=CARTESIAN_POINT('Ctrl Pts',(-7.50891486634214,-17.4330545448126,
21.));
#10685=CARTESIAN_POINT('Ctrl Pts',(-7.52019696747329,-17.4790653226646,
0.));
#10686=CARTESIAN_POINT('Ctrl Pts',(-7.52019696747329,-17.4790653226646,
21.));
#10687=CARTESIAN_POINT('Ctrl Pts',(-7.53103903007864,-17.5252518287336,
0.));
#10688=CARTESIAN_POINT('Ctrl Pts',(-7.53103903007864,-17.5252518287336,
21.));
#10689=CARTESIAN_POINT('Ctrl Pts',(-7.54158441095318,-17.5715579419204,
0.));
#10690=CARTESIAN_POINT('Ctrl Pts',(-7.54158441095318,-17.5715579419204,
21.));
#10691=CARTESIAN_POINT('Ctrl Pts',(-7.55182125346564,-17.6179818599248,
0.));
#10692=CARTESIAN_POINT('Ctrl Pts',(-7.55182125346564,-17.6179818599248,
21.));
#10693=CARTESIAN_POINT('Ctrl Pts',(-7.56164400295863,-17.6645549117314,
0.));
#10694=CARTESIAN_POINT('Ctrl Pts',(-7.56164400295863,-17.6645549117314,
21.));
#10695=CARTESIAN_POINT('Ctrl Pts',(-7.57091795530424,-17.7113192869136,
0.));
#10696=CARTESIAN_POINT('Ctrl Pts',(-7.57091795530424,-17.7113192869136,
21.));
#10697=CARTESIAN_POINT('Ctrl Pts',(-7.57954834582804,-17.7583042294209,
0.));
#10698=CARTESIAN_POINT('Ctrl Pts',(-7.57954834582804,-17.7583042294209,
21.));
#10699=CARTESIAN_POINT('Ctrl Pts',(-7.58752955799499,-17.8055090348024,
0.));
#10700=CARTESIAN_POINT('Ctrl Pts',(-7.58752955799499,-17.8055090348024,
21.));
#10701=CARTESIAN_POINT('Ctrl Pts',(-7.59491004201956,-17.8529149331931,
0.));
#10702=CARTESIAN_POINT('Ctrl Pts',(-7.59491004201956,-17.8529149331931,
21.));
#10703=CARTESIAN_POINT('Ctrl Pts',(-7.60176928403059,-17.900492838997,0.));
#10704=CARTESIAN_POINT('Ctrl Pts',(-7.60176928403059,-17.900492838997,21.));
#10705=CARTESIAN_POINT('Ctrl Pts',(-7.60819152580111,-17.9482122228183,
0.));
#10706=CARTESIAN_POINT('Ctrl Pts',(-7.60819152580111,-17.9482122228183,
21.));
#10707=CARTESIAN_POINT('Ctrl Pts',(-7.61423755067038,-17.9960506269561,
0.));
#10708=CARTESIAN_POINT('Ctrl Pts',(-7.61423755067038,-17.9960506269561,
21.));
#10709=CARTESIAN_POINT('Ctrl Pts',(-7.61992799636654,-18.0439992897906,
0.));
#10710=CARTESIAN_POINT('Ctrl Pts',(-7.61992799636654,-18.0439992897906,
21.));
#10711=CARTESIAN_POINT('Ctrl Pts',(-7.62525915358074,-18.0920577897363,
0.));
#10712=CARTESIAN_POINT('Ctrl Pts',(-7.62525915358074,-18.0920577897363,
21.));
#10713=CARTESIAN_POINT('Ctrl Pts',(-7.63021285851762,-18.1402306858819,
0.));
#10714=CARTESIAN_POINT('Ctrl Pts',(-7.63021285851762,-18.1402306858819,
21.));
#10715=CARTESIAN_POINT('Ctrl Pts',(-7.63476798969017,-18.1885236169197,
0.));
#10716=CARTESIAN_POINT('Ctrl Pts',(-7.63476798969017,-18.1885236169197,
21.));
#10717=CARTESIAN_POINT('Ctrl Pts',(-7.63891299603827,-18.2369390502576,
0.));
#10718=CARTESIAN_POINT('Ctrl Pts',(-7.63891299603827,-18.2369390502576,
21.));
#10719=CARTESIAN_POINT('Ctrl Pts',(-7.6426522027076,-18.2854741391282,0.));
#10720=CARTESIAN_POINT('Ctrl Pts',(-7.6426522027076,-18.2854741391282,21.));
#10721=CARTESIAN_POINT('Ctrl Pts',(-7.64599903846601,-18.3341230095852,
0.));
#10722=CARTESIAN_POINT('Ctrl Pts',(-7.64599903846601,-18.3341230095852,
21.));
#10723=CARTESIAN_POINT('Ctrl Pts',(-7.6489719793775,-18.3828781275628,0.));
#10724=CARTESIAN_POINT('Ctrl Pts',(-7.6489719793775,-18.3828781275628,21.));
#10725=CARTESIAN_POINT('Ctrl Pts',(-7.65158974829127,-18.4317319183719,
0.));
#10726=CARTESIAN_POINT('Ctrl Pts',(-7.65158974829127,-18.4317319183719,
21.));
#10727=CARTESIAN_POINT('Ctrl Pts',(-7.65386603444743,-18.4806785483052,
0.));
#10728=CARTESIAN_POINT('Ctrl Pts',(-7.65386603444743,-18.4806785483052,
21.));
#10729=CARTESIAN_POINT('Ctrl Pts',(-7.65580722110437,-18.5297146894905,
0.));
#10730=CARTESIAN_POINT('Ctrl Pts',(-7.65580722110437,-18.5297146894905,
21.));
#10731=CARTESIAN_POINT('Ctrl Pts',(-7.65741532450727,-18.5788385228928,
0.));
#10732=CARTESIAN_POINT('Ctrl Pts',(-7.65741532450727,-18.5788385228928,
21.));
#10733=CARTESIAN_POINT('Ctrl Pts',(-7.65868976978872,-18.6280491346907,
0.));
#10734=CARTESIAN_POINT('Ctrl Pts',(-7.65868976978872,-18.6280491346907,
21.));
#10735=CARTESIAN_POINT('Ctrl Pts',(-7.65962948375622,-18.6773458057584,
0.));
#10736=CARTESIAN_POINT('Ctrl Pts',(-7.65962948375622,-18.6773458057584,
21.));
#10737=CARTESIAN_POINT('Ctrl Pts',(-7.66023521705905,-18.7267272235231,
0.));
#10738=CARTESIAN_POINT('Ctrl Pts',(-7.66023521705905,-18.7267272235231,
21.));
#10739=CARTESIAN_POINT('Ctrl Pts',(-7.66051046922541,-18.7761911671591,
0.));
#10740=CARTESIAN_POINT('Ctrl Pts',(-7.66051046922541,-18.7761911671591,
21.));
#10741=CARTESIAN_POINT('Ctrl Pts',(-7.66046025294775,-18.8257349246207,
0.));
#10742=CARTESIAN_POINT('Ctrl Pts',(-7.66046025294775,-18.8257349246207,
21.));
#10743=CARTESIAN_POINT('Ctrl Pts',(-7.66009036321663,-18.8753555389435,
0.));
#10744=CARTESIAN_POINT('Ctrl Pts',(-7.66009036321663,-18.8753555389435,
21.));
#10745=CARTESIAN_POINT('Ctrl Pts',(-7.65940650980099,-18.9250501008887,
0.));
#10746=CARTESIAN_POINT('Ctrl Pts',(-7.65940650980099,-18.9250501008887,
21.));
#10747=CARTESIAN_POINT('Ctrl Pts',(-7.65841335587266,-18.974816073814,0.));
#10748=CARTESIAN_POINT('Ctrl Pts',(-7.65841335587266,-18.974816073814,21.));
#10749=CARTESIAN_POINT('Ctrl Pts',(-7.65711415727855,-19.0246514144531,
0.));
#10750=CARTESIAN_POINT('Ctrl Pts',(-7.65711415727855,-19.0246514144531,
21.));
#10751=CARTESIAN_POINT('Ctrl Pts',(-7.65551129907202,-19.0745543888799,
0.));
#10752=CARTESIAN_POINT('Ctrl Pts',(-7.65551129907202,-19.0745543888799,
21.));
#10753=CARTESIAN_POINT('Ctrl Pts',(-7.65360662280609,-19.1245234597312,
0.));
#10754=CARTESIAN_POINT('Ctrl Pts',(-7.65360662280609,-19.1245234597312,
21.));
#10755=CARTESIAN_POINT('Ctrl Pts',(-7.65140181220526,-19.1745571539291,
0.));
#10756=CARTESIAN_POINT('Ctrl Pts',(-7.65140181220526,-19.1745571539291,
21.));
#10757=CARTESIAN_POINT('Ctrl Pts',(-7.64889882291924,-19.224653915265,0.));
#10758=CARTESIAN_POINT('Ctrl Pts',(-7.64889882291924,-19.224653915265,21.));
#10759=CARTESIAN_POINT('Ctrl Pts',(-7.64610005549614,-19.2748120456486,
0.));
#10760=CARTESIAN_POINT('Ctrl Pts',(-7.64610005549614,-19.2748120456486,
21.));
#10761=CARTESIAN_POINT('Ctrl Pts',(-7.64300812875339,-19.3250297839295,
0.));
#10762=CARTESIAN_POINT('Ctrl Pts',(-7.64300812875339,-19.3250297839295,
21.));
#10763=CARTESIAN_POINT('Ctrl Pts',(-7.63962574822761,-19.3753053524647,
0.));
#10764=CARTESIAN_POINT('Ctrl Pts',(-7.63962574822761,-19.3753053524647,
21.));
#10765=CARTESIAN_POINT('Ctrl Pts',(-7.63595554930654,-19.4256370121006,
0.));
#10766=CARTESIAN_POINT('Ctrl Pts',(-7.63595554930654,-19.4256370121006,
21.));
#10767=CARTESIAN_POINT('Ctrl Pts',(-7.63199992715366,-19.4760231231881,
0.));
#10768=CARTESIAN_POINT('Ctrl Pts',(-7.63199992715366,-19.4760231231881,
21.));
#10769=CARTESIAN_POINT('Ctrl Pts',(-7.62776096538883,-19.5264621687521,
0.));
#10770=CARTESIAN_POINT('Ctrl Pts',(-7.62776096538883,-19.5264621687521,
21.));
#10771=CARTESIAN_POINT('Ctrl Pts',(-7.6232405373522,-19.5769527121826,0.));
#10772=CARTESIAN_POINT('Ctrl Pts',(-7.6232405373522,-19.5769527121826,21.));
#10773=CARTESIAN_POINT('Ctrl Pts',(-7.61844037070591,-19.6274933688524,
0.));
#10774=CARTESIAN_POINT('Ctrl Pts',(-7.61844037070591,-19.6274933688524,
21.));
#10775=CARTESIAN_POINT('Ctrl Pts',(-7.61336212350879,-19.6780827744426,
0.));
#10776=CARTESIAN_POINT('Ctrl Pts',(-7.61336212350879,-19.6780827744426,
21.));
#10777=CARTESIAN_POINT('Ctrl Pts',(-7.60800746969262,-19.7287195480601,
0.));
#10778=CARTESIAN_POINT('Ctrl Pts',(-7.60800746969262,-19.7287195480601,
21.));
#10779=CARTESIAN_POINT('Ctrl Pts',(-7.60237814110187,-19.7794022782484,
0.));
#10780=CARTESIAN_POINT('Ctrl Pts',(-7.60237814110187,-19.7794022782484,
21.));
#10781=CARTESIAN_POINT('Ctrl Pts',(-7.59647587605448,-19.830129556152,0.));
#10782=CARTESIAN_POINT('Ctrl Pts',(-7.59647587605448,-19.830129556152,21.));
#10783=CARTESIAN_POINT('Ctrl Pts',(-7.59030238888852,-19.8808999994024,
0.));
#10784=CARTESIAN_POINT('Ctrl Pts',(-7.59030238888852,-19.8808999994024,
21.));
#10785=CARTESIAN_POINT('Ctrl Pts',(-7.58385933533352,-19.931712276832,0.));
#10786=CARTESIAN_POINT('Ctrl Pts',(-7.58385933533352,-19.931712276832,21.));
#10787=CARTESIAN_POINT('Ctrl Pts',(-7.57714827622806,-19.9825651387294,
0.));
#10788=CARTESIAN_POINT('Ctrl Pts',(-7.57714827622806,-19.9825651387294,
21.));
#10789=CARTESIAN_POINT('Ctrl Pts',(-7.57017066105973,-20.0334574248556,
0.));
#10790=CARTESIAN_POINT('Ctrl Pts',(-7.57017066105973,-20.0334574248556,
21.));
#10791=CARTESIAN_POINT('Ctrl Pts',(-7.56292786549461,-20.0843880130978,
0.));
#10792=CARTESIAN_POINT('Ctrl Pts',(-7.56292786549461,-20.0843880130978,
21.));
#10793=CARTESIAN_POINT('Ctrl Pts',(-7.55542122125495,-20.1353557774357,
0.));
#10794=CARTESIAN_POINT('Ctrl Pts',(-7.55542122125495,-20.1353557774357,
21.));
#10795=CARTESIAN_POINT('Ctrl Pts',(-7.54765204869255,-20.1863595454674,
0.));
#10796=CARTESIAN_POINT('Ctrl Pts',(-7.54765204869255,-20.1863595454674,
21.));
#10797=CARTESIAN_POINT('Ctrl Pts',(-7.53962169534167,-20.2373980474879,
0.));
#10798=CARTESIAN_POINT('Ctrl Pts',(-7.53962169534167,-20.2373980474879,
21.));
#10799=CARTESIAN_POINT('Ctrl Pts',(-7.53133155804008,-20.2884698940944,
0.));
#10800=CARTESIAN_POINT('Ctrl Pts',(-7.53133155804008,-20.2884698940944,
21.));
#10801=CARTESIAN_POINT('Ctrl Pts',(-7.52278303006887,-20.3395736743243,
0.));
#10802=CARTESIAN_POINT('Ctrl Pts',(-7.52278303006887,-20.3395736743243,
21.));
#10803=CARTESIAN_POINT('Ctrl Pts',(-7.51397746081994,-20.3907080367098,
0.));
#10804=CARTESIAN_POINT('Ctrl Pts',(-7.51397746081994,-20.3907080367098,
21.));
#10805=CARTESIAN_POINT('Ctrl Pts',(-7.50491611266253,-20.4418717748497,
0.));
#10806=CARTESIAN_POINT('Ctrl Pts',(-7.50491611266253,-20.4418717748497,
21.));
#10807=CARTESIAN_POINT('Ctrl Pts',(-7.49560012018406,-20.493063915616,0.));
#10808=CARTESIAN_POINT('Ctrl Pts',(-7.49560012018406,-20.493063915616,21.));
#10809=CARTESIAN_POINT('Ctrl Pts',(-7.48603045196745,-20.5442837929044,
0.));
#10810=CARTESIAN_POINT('Ctrl Pts',(-7.48603045196745,-20.5442837929044,
21.));
#10811=CARTESIAN_POINT('Ctrl Pts',(-7.47620789245428,-20.5955309838521,
0.));
#10812=CARTESIAN_POINT('Ctrl Pts',(-7.47620789245428,-20.5955309838521,
21.));
#10813=CARTESIAN_POINT('Ctrl Pts',(-7.46814799701906,-20.6365504027501,
0.));
#10814=CARTESIAN_POINT('Ctrl Pts',(-7.46814799701906,-20.6365504027501,
21.));
#10815=CARTESIAN_POINT('Ctrl Pts',(-7.46198969876654,-20.6673271112931,
0.));
#10816=CARTESIAN_POINT('Ctrl Pts',(-7.46198969876654,-20.6673271112931,
21.));
#10817=CARTESIAN_POINT('Ctrl Pts',(-7.45783379370108,-20.6878503127065,
0.));
#10818=CARTESIAN_POINT('Ctrl Pts',(-7.45783379370108,-20.6878503127065,
21.));
#10819=CARTESIAN_POINT('Ctrl Pts',(-7.45574324794401,-20.698113262342,0.));
#10820=CARTESIAN_POINT('Ctrl Pts',(-7.45574324794401,-20.698113262342,21.));
#10821=CARTESIAN_POINT('Ctrl Pts',(-7.45007618140239,-17.2541372868972,
0.));
#10822=CARTESIAN_POINT('Ctrl Pts',(-7.45381253347183,-17.2627905583523,
0.));
#10823=CARTESIAN_POINT('Ctrl Pts',(-7.46105049818251,-17.2801832097582,
0.));
#10824=CARTESIAN_POINT('Ctrl Pts',(-7.4712032346092,-17.3065305096784,0.));
#10825=CARTESIAN_POINT('Ctrl Pts',(-7.48340100912745,-17.3421522689127,
0.));
#10826=CARTESIAN_POINT('Ctrl Pts',(-7.49681774451751,-17.3873563447297,
0.));
#10827=CARTESIAN_POINT('Ctrl Pts',(-7.50891486634214,-17.4330545448126,
0.));
#10828=CARTESIAN_POINT('Ctrl Pts',(-7.52019696747329,-17.4790653226646,
0.));
#10829=CARTESIAN_POINT('Ctrl Pts',(-7.53103903007864,-17.5252518287336,
0.));
#10830=CARTESIAN_POINT('Ctrl Pts',(-7.54158441095318,-17.5715579419204,
0.));
#10831=CARTESIAN_POINT('Ctrl Pts',(-7.55182125346564,-17.6179818599248,
0.));
#10832=CARTESIAN_POINT('Ctrl Pts',(-7.56164400295863,-17.6645549117314,
0.));
#10833=CARTESIAN_POINT('Ctrl Pts',(-7.57091795530424,-17.7113192869136,
0.));
#10834=CARTESIAN_POINT('Ctrl Pts',(-7.57954834582804,-17.7583042294209,
0.));
#10835=CARTESIAN_POINT('Ctrl Pts',(-7.58752955799499,-17.8055090348024,
0.));
#10836=CARTESIAN_POINT('Ctrl Pts',(-7.59491004201956,-17.8529149331931,
0.));
#10837=CARTESIAN_POINT('Ctrl Pts',(-7.60176928403059,-17.900492838997,0.));
#10838=CARTESIAN_POINT('Ctrl Pts',(-7.60819152580111,-17.9482122228183,
0.));
#10839=CARTESIAN_POINT('Ctrl Pts',(-7.61423755067038,-17.9960506269561,
0.));
#10840=CARTESIAN_POINT('Ctrl Pts',(-7.61992799636654,-18.0439992897906,
0.));
#10841=CARTESIAN_POINT('Ctrl Pts',(-7.62525915358074,-18.0920577897363,
0.));
#10842=CARTESIAN_POINT('Ctrl Pts',(-7.63021285851762,-18.1402306858819,
0.));
#10843=CARTESIAN_POINT('Ctrl Pts',(-7.63476798969017,-18.1885236169197,
0.));
#10844=CARTESIAN_POINT('Ctrl Pts',(-7.63891299603827,-18.2369390502576,
0.));
#10845=CARTESIAN_POINT('Ctrl Pts',(-7.6426522027076,-18.2854741391282,0.));
#10846=CARTESIAN_POINT('Ctrl Pts',(-7.64599903846601,-18.3341230095852,
0.));
#10847=CARTESIAN_POINT('Ctrl Pts',(-7.6489719793775,-18.3828781275628,0.));
#10848=CARTESIAN_POINT('Ctrl Pts',(-7.65158974829127,-18.4317319183719,
0.));
#10849=CARTESIAN_POINT('Ctrl Pts',(-7.65386603444743,-18.4806785483052,
0.));
#10850=CARTESIAN_POINT('Ctrl Pts',(-7.65580722110437,-18.5297146894905,
0.));
#10851=CARTESIAN_POINT('Ctrl Pts',(-7.65741532450727,-18.5788385228928,
0.));
#10852=CARTESIAN_POINT('Ctrl Pts',(-7.65868976978872,-18.6280491346907,
0.));
#10853=CARTESIAN_POINT('Ctrl Pts',(-7.65962948375622,-18.6773458057584,
0.));
#10854=CARTESIAN_POINT('Ctrl Pts',(-7.66023521705905,-18.7267272235231,
0.));
#10855=CARTESIAN_POINT('Ctrl Pts',(-7.66051046922541,-18.7761911671591,
0.));
#10856=CARTESIAN_POINT('Ctrl Pts',(-7.66046025294775,-18.8257349246207,
0.));
#10857=CARTESIAN_POINT('Ctrl Pts',(-7.66009036321663,-18.8753555389435,
0.));
#10858=CARTESIAN_POINT('Ctrl Pts',(-7.65940650980099,-18.9250501008887,
0.));
#10859=CARTESIAN_POINT('Ctrl Pts',(-7.65841335587266,-18.974816073814,0.));
#10860=CARTESIAN_POINT('Ctrl Pts',(-7.65711415727855,-19.0246514144531,
0.));
#10861=CARTESIAN_POINT('Ctrl Pts',(-7.65551129907202,-19.0745543888799,
0.));
#10862=CARTESIAN_POINT('Ctrl Pts',(-7.65360662280609,-19.1245234597312,
0.));
#10863=CARTESIAN_POINT('Ctrl Pts',(-7.65140181220526,-19.1745571539291,
0.));
#10864=CARTESIAN_POINT('Ctrl Pts',(-7.64889882291924,-19.224653915265,0.));
#10865=CARTESIAN_POINT('Ctrl Pts',(-7.64610005549614,-19.2748120456486,
0.));
#10866=CARTESIAN_POINT('Ctrl Pts',(-7.64300812875339,-19.3250297839295,
0.));
#10867=CARTESIAN_POINT('Ctrl Pts',(-7.63962574822761,-19.3753053524647,
0.));
#10868=CARTESIAN_POINT('Ctrl Pts',(-7.63595554930654,-19.4256370121006,
0.));
#10869=CARTESIAN_POINT('Ctrl Pts',(-7.63199992715366,-19.4760231231881,
0.));
#10870=CARTESIAN_POINT('Ctrl Pts',(-7.62776096538883,-19.5264621687521,
0.));
#10871=CARTESIAN_POINT('Ctrl Pts',(-7.6232405373522,-19.5769527121826,0.));
#10872=CARTESIAN_POINT('Ctrl Pts',(-7.61844037070591,-19.6274933688524,
0.));
#10873=CARTESIAN_POINT('Ctrl Pts',(-7.61336212350879,-19.6780827744426,
0.));
#10874=CARTESIAN_POINT('Ctrl Pts',(-7.60800746969262,-19.7287195480601,
0.));
#10875=CARTESIAN_POINT('Ctrl Pts',(-7.60237814110187,-19.7794022782484,
0.));
#10876=CARTESIAN_POINT('Ctrl Pts',(-7.59647587605448,-19.830129556152,0.));
#10877=CARTESIAN_POINT('Ctrl Pts',(-7.59030238888852,-19.8808999994024,
0.));
#10878=CARTESIAN_POINT('Ctrl Pts',(-7.58385933533352,-19.931712276832,0.));
#10879=CARTESIAN_POINT('Ctrl Pts',(-7.57714827622806,-19.9825651387294,
0.));
#10880=CARTESIAN_POINT('Ctrl Pts',(-7.57017066105973,-20.0334574248556,
0.));
#10881=CARTESIAN_POINT('Ctrl Pts',(-7.56292786549461,-20.0843880130978,
0.));
#10882=CARTESIAN_POINT('Ctrl Pts',(-7.55542122125495,-20.1353557774357,
0.));
#10883=CARTESIAN_POINT('Ctrl Pts',(-7.54765204869255,-20.1863595454674,
0.));
#10884=CARTESIAN_POINT('Ctrl Pts',(-7.53962169534167,-20.2373980474879,
0.));
#10885=CARTESIAN_POINT('Ctrl Pts',(-7.53133155804008,-20.2884698940944,
0.));
#10886=CARTESIAN_POINT('Ctrl Pts',(-7.52278303006887,-20.3395736743243,
0.));
#10887=CARTESIAN_POINT('Ctrl Pts',(-7.51397746081994,-20.3907080367098,
0.));
#10888=CARTESIAN_POINT('Ctrl Pts',(-7.50491611266253,-20.4418717748497,
0.));
#10889=CARTESIAN_POINT('Ctrl Pts',(-7.49560012018406,-20.493063915616,0.));
#10890=CARTESIAN_POINT('Ctrl Pts',(-7.48411651832413,-20.5545277683621,
0.));
#10891=CARTESIAN_POINT('Ctrl Pts',(-7.47423073598682,-20.6057817877246,
0.));
#10892=CARTESIAN_POINT('Ctrl Pts',(-7.46612041736314,-20.6468066077586,
0.));
#10893=CARTESIAN_POINT('Ctrl Pts',(-7.45992433946824,-20.6775873630604,
0.));
#10894=CARTESIAN_POINT('Ctrl Pts',(-7.45574324794401,-20.698113262342,0.));
#10895=CARTESIAN_POINT('Ctrl Pts',(-7.45007618140239,-17.2541372868972,
13.));
#10896=CARTESIAN_POINT('Ctrl Pts',(-7.45637364573816,-17.2687220121489,
13.));
#10897=CARTESIAN_POINT('Ctrl Pts',(-7.46226667103919,-17.2834550499008,
13.));
#10898=CARTESIAN_POINT('Ctrl Pts',(-7.46778231425445,-17.2983267669067,
13.));
#10899=CARTESIAN_POINT('Ctrl Pts',(-7.47424706065699,-17.3157575315993,
13.));
#10900=CARTESIAN_POINT('Ctrl Pts',(-7.48019417753821,-17.3333785326113,
13.));
#10901=CARTESIAN_POINT('Ctrl Pts',(-7.48573450280811,-17.3511502187375,
13.));
#10902=CARTESIAN_POINT('Ctrl Pts',(-7.49353000563121,-17.3761558316968,
13.));
#10903=CARTESIAN_POINT('Ctrl Pts',(-7.50052692940225,-17.4014574303076,
13.));
#10904=CARTESIAN_POINT('Ctrl Pts',(-7.50711117101491,-17.4269165094415,
13.));
#10905=CARTESIAN_POINT('Ctrl Pts',(-7.51149073008789,-17.4438508122163,
13.));
#10906=CARTESIAN_POINT('Ctrl Pts',(-7.51568961154288,-17.4608540901313,
13.));
#10907=CARTESIAN_POINT('Ctrl Pts',(-7.51979276933228,-17.477895354957,13.));
#10908=CARTESIAN_POINT('Ctrl Pts',(-7.52411201550939,-17.4958340796489,
13.));
#10909=CARTESIAN_POINT('Ctrl Pts',(-7.52832602172309,-17.5138146001159,
13.));
#10910=CARTESIAN_POINT('Ctrl Pts',(-7.53247314101538,-17.5318219263269,
13.));
#10911=CARTESIAN_POINT('Ctrl Pts',(-7.53707874400482,-17.5518200478141,
13.));
#10912=CARTESIAN_POINT('Ctrl Pts',(-7.54160061545737,-17.5718516505912,
13.));
#10913=CARTESIAN_POINT('Ctrl Pts',(-7.5460260137895,-17.5919190740356,13.));
#10914=CARTESIAN_POINT('Ctrl Pts',(-7.55269751656612,-17.6221716888696,
13.));
#10915=CARTESIAN_POINT('Ctrl Pts',(-7.55914375118857,-17.6525076946371,
13.));
#10916=CARTESIAN_POINT('Ctrl Pts',(-7.56521559976811,-17.6829731243219,
13.));
#10917=CARTESIAN_POINT('Ctrl Pts',(-7.56962666501585,-17.7051055929398,
13.));
#10918=CARTESIAN_POINT('Ctrl Pts',(-7.57383703867015,-17.727307481075,13.));
#10919=CARTESIAN_POINT('Ctrl Pts',(-7.57782678310872,-17.7495842479971,
13.));
#10920=CARTESIAN_POINT('Ctrl Pts',(-7.58270390405109,-17.7768156880447,
13.));
#10921=CARTESIAN_POINT('Ctrl Pts',(-7.58725254420668,-17.8041586050554,
13.));
#10922=CARTESIAN_POINT('Ctrl Pts',(-7.59151733245669,-17.8315958504975,
13.));
#10923=CARTESIAN_POINT('Ctrl Pts',(-7.59612401157578,-17.8612326292199,
13.));
#10924=CARTESIAN_POINT('Ctrl Pts',(-7.60040516926074,-17.890977551337,13.));
#10925=CARTESIAN_POINT('Ctrl Pts',(-7.60444696777948,-17.9207992272247,
13.));
#10926=CARTESIAN_POINT('Ctrl Pts',(-7.60817833718655,-17.9483304583238,
13.));
#10927=CARTESIAN_POINT('Ctrl Pts',(-7.61170808544497,-17.9759263070057,
13.));
#10928=CARTESIAN_POINT('Ctrl Pts',(-7.61506270604885,-18.0035762489904,
13.));
#10929=CARTESIAN_POINT('Ctrl Pts',(-7.61962013038026,-18.0411401148466,
13.));
#10930=CARTESIAN_POINT('Ctrl Pts',(-7.62385245909278,-18.078804438117,13.));
#10931=CARTESIAN_POINT('Ctrl Pts',(-7.62773031180414,-18.1165756810882,
13.));
#10932=CARTESIAN_POINT('Ctrl Pts',(-7.63147235591759,-18.1530241147805,
13.));
#10933=CARTESIAN_POINT('Ctrl Pts',(-7.63487692331431,-18.1895746220981,
13.));
#10934=CARTESIAN_POINT('Ctrl Pts',(-7.63792794642091,-18.226229844125,13.));
#10935=CARTESIAN_POINT('Ctrl Pts',(-7.6420728467942,-18.2760269902476,13.));
#10936=CARTESIAN_POINT('Ctrl Pts',(-7.64556831472346,-18.3260163399595,
13.));
#10937=CARTESIAN_POINT('Ctrl Pts',(-7.64849356609124,-18.3761647741053,
13.));
#10938=CARTESIAN_POINT('Ctrl Pts',(-7.65106479845333,-18.4202441575742,
13.));
#10939=CARTESIAN_POINT('Ctrl Pts',(-7.65320196597273,-18.4644442731323,
13.));
#10940=CARTESIAN_POINT('Ctrl Pts',(-7.65493429570881,-18.5087513218567,
13.));
#10941=CARTESIAN_POINT('Ctrl Pts',(-7.65748817031469,-18.5740706685388,
13.));
#10942=CARTESIAN_POINT('Ctrl Pts',(-7.65915358769517,-18.6396252901705,
13.));
#10943=CARTESIAN_POINT('Ctrl Pts',(-7.65993127489945,-18.7054034394317,
13.));
#10944=CARTESIAN_POINT('Ctrl Pts',(-7.66091272374024,-18.7884161056895,
13.));
#10945=CARTESIAN_POINT('Ctrl Pts',(-7.66048522719283,-18.8717830756661,
13.));
#10946=CARTESIAN_POINT('Ctrl Pts',(-7.65875983806947,-18.9554457129062,
13.));
#10947=CARTESIAN_POINT('Ctrl Pts',(-7.65642266547867,-19.0687732052289,
13.));
#10948=CARTESIAN_POINT('Ctrl Pts',(-7.65169843824266,-19.1826450748833,
13.));
#10949=CARTESIAN_POINT('Ctrl Pts',(-7.64469887386167,-19.2969757396511,
13.));
#10950=CARTESIAN_POINT('Ctrl Pts',(-7.63845857891806,-19.3989045212746,
13.));
#10951=CARTESIAN_POINT('Ctrl Pts',(-7.63041784747171,-19.5011952230427,
13.));
#10952=CARTESIAN_POINT('Ctrl Pts',(-7.62065725315813,-19.6037897795036,
13.));
#10953=CARTESIAN_POINT('Ctrl Pts',(-7.6068238069441,-19.7491944785472,13.));
#10954=CARTESIAN_POINT('Ctrl Pts',(-7.5895301524174,-19.8952104286167,13.));
#10955=CARTESIAN_POINT('Ctrl Pts',(-7.56895177464837,-20.0416957573265,
13.));
#10956=CARTESIAN_POINT('Ctrl Pts',(-7.55296697971251,-20.15548208037,13.));
#10957=CARTESIAN_POINT('Ctrl Pts',(-7.53499708076544,-20.2695554921735,
13.));
#10958=CARTESIAN_POINT('Ctrl Pts',(-7.51511029118453,-20.3838501740658,
13.));
#10959=CARTESIAN_POINT('Ctrl Pts',(-7.4979067159171,-20.482723707906,13.));
#10960=CARTESIAN_POINT('Ctrl Pts',(-7.47927116738907,-20.5817593863818,
13.));
#10961=CARTESIAN_POINT('Ctrl Pts',(-7.45922688157452,-20.6809436221336,
13.));
#10962=CARTESIAN_POINT('Ctrl Pts',(-7.45807037084351,-20.6866663320398,
13.));
#10963=CARTESIAN_POINT('Ctrl Pts',(-7.45690915954643,-20.6923895454539,
13.));
#10964=CARTESIAN_POINT('Ctrl Pts',(-7.45574324794401,-20.698113262342,13.));
#10965=CARTESIAN_POINT('Ctrl Pts',(-12.3627494547115,-18.1978687191668,
0.));
#10966=CARTESIAN_POINT('Ctrl Pts',(-12.3627494547115,-18.1978687191668,
21.));
#10967=CARTESIAN_POINT('Ctrl Pts',(-12.3532177620787,-18.1935275957711,
0.));
#10968=CARTESIAN_POINT('Ctrl Pts',(-12.3532177620787,-18.1935275957711,
21.));
#10969=CARTESIAN_POINT('Ctrl Pts',(-12.3341713636489,-18.1848265584754,
0.));
#10970=CARTESIAN_POINT('Ctrl Pts',(-12.3341713636489,-18.1848265584754,
21.));
#10971=CARTESIAN_POINT('Ctrl Pts',(-12.3056527265146,-18.1717186310224,
0.));
#10972=CARTESIAN_POINT('Ctrl Pts',(-12.3056527265146,-18.1717186310224,
21.));
#10973=CARTESIAN_POINT('Ctrl Pts',(-12.2677298318549,-18.1541286139166,
0.));
#10974=CARTESIAN_POINT('Ctrl Pts',(-12.2677298318549,-18.1541286139166,
21.));
#10975=CARTESIAN_POINT('Ctrl Pts',(-12.2204964278426,-18.1319528884305,
0.));
#10976=CARTESIAN_POINT('Ctrl Pts',(-12.2204964278426,-18.1319528884305,
21.));
#10977=CARTESIAN_POINT('Ctrl Pts',(-12.1734337668195,-18.109588624154,0.));
#10978=CARTESIAN_POINT('Ctrl Pts',(-12.1734337668195,-18.109588624154,21.));
#10979=CARTESIAN_POINT('Ctrl Pts',(-12.1265426519718,-18.0870354350128,
0.));
#10980=CARTESIAN_POINT('Ctrl Pts',(-12.1265426519718,-18.0870354350128,
21.));
#10981=CARTESIAN_POINT('Ctrl Pts',(-12.0798241915081,-18.0642929289333,
0.));
#10982=CARTESIAN_POINT('Ctrl Pts',(-12.0798241915081,-18.0642929289333,
21.));
#10983=CARTESIAN_POINT('Ctrl Pts',(-12.0332798395991,-18.0413607600052,
0.));
#10984=CARTESIAN_POINT('Ctrl Pts',(-12.0332798395991,-18.0413607600052,
21.));
#10985=CARTESIAN_POINT('Ctrl Pts',(-11.986911314246,-18.0182386160553,0.));
#10986=CARTESIAN_POINT('Ctrl Pts',(-11.986911314246,-18.0182386160553,21.));
#10987=CARTESIAN_POINT('Ctrl Pts',(-11.9407205019619,-17.9949261997754,
0.));
#10988=CARTESIAN_POINT('Ctrl Pts',(-11.9407205019619,-17.9949261997754,
21.));
#10989=CARTESIAN_POINT('Ctrl Pts',(-11.8947093631895,-17.9714232133203,
0.));
#10990=CARTESIAN_POINT('Ctrl Pts',(-11.8947093631895,-17.9714232133203,
21.));
#10991=CARTESIAN_POINT('Ctrl Pts',(-11.8488798430201,-17.9477293432951,
0.));
#10992=CARTESIAN_POINT('Ctrl Pts',(-11.8488798430201,-17.9477293432951,
21.));
#10993=CARTESIAN_POINT('Ctrl Pts',(-11.8032337607271,-17.9238442458356,
0.));
#10994=CARTESIAN_POINT('Ctrl Pts',(-11.8032337607271,-17.9238442458356,
21.));
#10995=CARTESIAN_POINT('Ctrl Pts',(-11.7577728408871,-17.8997675418752,
0.));
#10996=CARTESIAN_POINT('Ctrl Pts',(-11.7577728408871,-17.8997675418752,
21.));
#10997=CARTESIAN_POINT('Ctrl Pts',(-11.7124987772363,-17.8754988158862,
0.));
#10998=CARTESIAN_POINT('Ctrl Pts',(-11.7124987772363,-17.8754988158862,
21.));
#10999=CARTESIAN_POINT('Ctrl Pts',(-11.6674132861792,-17.8510376144926,
0.));
#11000=CARTESIAN_POINT('Ctrl Pts',(-11.6674132861792,-17.8510376144926,
21.));
#11001=CARTESIAN_POINT('Ctrl Pts',(-11.6225181583564,-17.8263834470057,
0.));
#11002=CARTESIAN_POINT('Ctrl Pts',(-11.6225181583564,-17.8263834470057,
21.));
#11003=CARTESIAN_POINT('Ctrl Pts',(-11.5778153222435,-17.8015357852426,
0.));
#11004=CARTESIAN_POINT('Ctrl Pts',(-11.5778153222435,-17.8015357852426,
21.));
#11005=CARTESIAN_POINT('Ctrl Pts',(-11.5333068279911,-17.7764940721306,
0.));
#11006=CARTESIAN_POINT('Ctrl Pts',(-11.5333068279911,-17.7764940721306,
21.));
#11007=CARTESIAN_POINT('Ctrl Pts',(-11.4889948016216,-17.7512577332768,
0.));
#11008=CARTESIAN_POINT('Ctrl Pts',(-11.4889948016216,-17.7512577332768,
21.));
#11009=CARTESIAN_POINT('Ctrl Pts',(-11.4448814046804,-17.725826190457,0.));
#11010=CARTESIAN_POINT('Ctrl Pts',(-11.4448814046804,-17.725826190457,21.));
#11011=CARTESIAN_POINT('Ctrl Pts',(-11.4009687970126,-17.700198872213,0.));
#11012=CARTESIAN_POINT('Ctrl Pts',(-11.4009687970126,-17.700198872213,21.));
#11013=CARTESIAN_POINT('Ctrl Pts',(-11.3572590796967,-17.674375235974,0.));
#11014=CARTESIAN_POINT('Ctrl Pts',(-11.3572590796967,-17.674375235974,21.));
#11015=CARTESIAN_POINT('Ctrl Pts',(-11.3137543310722,-17.6483547422688,
0.));
#11016=CARTESIAN_POINT('Ctrl Pts',(-11.3137543310722,-17.6483547422688,
21.));
#11017=CARTESIAN_POINT('Ctrl Pts',(-11.2704566868205,-17.6221368072528,
0.));
#11018=CARTESIAN_POINT('Ctrl Pts',(-11.2704566868205,-17.6221368072528,
21.));
#11019=CARTESIAN_POINT('Ctrl Pts',(-11.2273684103051,-17.5957207597803,
0.));
#11020=CARTESIAN_POINT('Ctrl Pts',(-11.2273684103051,-17.5957207597803,
21.));
#11021=CARTESIAN_POINT('Ctrl Pts',(-11.1844919535058,-17.5691058058227,
0.));
#11022=CARTESIAN_POINT('Ctrl Pts',(-11.1844919535058,-17.5691058058227,
21.));
#11023=CARTESIAN_POINT('Ctrl Pts',(-11.1418300507683,-17.5422909714139,
0.));
#11024=CARTESIAN_POINT('Ctrl Pts',(-11.1418300507683,-17.5422909714139,
21.));
#11025=CARTESIAN_POINT('Ctrl Pts',(-11.0993856581394,-17.5152751467292,
0.));
#11026=CARTESIAN_POINT('Ctrl Pts',(-11.0993856581394,-17.5152751467292,
21.));
#11027=CARTESIAN_POINT('Ctrl Pts',(-11.0571618040371,-17.4880571878157,
0.));
#11028=CARTESIAN_POINT('Ctrl Pts',(-11.0571618040371,-17.4880571878157,
21.));
#11029=CARTESIAN_POINT('Ctrl Pts',(-11.0151614525642,-17.460636011184,0.));
#11030=CARTESIAN_POINT('Ctrl Pts',(-11.0151614525642,-17.460636011184,21.));
#11031=CARTESIAN_POINT('Ctrl Pts',(-10.9733873885115,-17.4330106728622,
0.));
#11032=CARTESIAN_POINT('Ctrl Pts',(-10.9733873885115,-17.4330106728622,
21.));
#11033=CARTESIAN_POINT('Ctrl Pts',(-10.9318420203801,-17.4051805054129,
0.));
#11034=CARTESIAN_POINT('Ctrl Pts',(-10.9318420203801,-17.4051805054129,
21.));
#11035=CARTESIAN_POINT('Ctrl Pts',(-10.8905275295837,-17.377145012528,0.));
#11036=CARTESIAN_POINT('Ctrl Pts',(-10.8905275295837,-17.377145012528,21.));
#11037=CARTESIAN_POINT('Ctrl Pts',(-10.8494462423128,-17.3489036079991,
0.));
#11038=CARTESIAN_POINT('Ctrl Pts',(-10.8494462423128,-17.3489036079991,
21.));
#11039=CARTESIAN_POINT('Ctrl Pts',(-10.8086009632423,-17.3204553814537,
0.));
#11040=CARTESIAN_POINT('Ctrl Pts',(-10.8086009632423,-17.3204553814537,
21.));
#11041=CARTESIAN_POINT('Ctrl Pts',(-10.7679952591482,-17.2917988998581,
0.));
#11042=CARTESIAN_POINT('Ctrl Pts',(-10.7679952591482,-17.2917988998581,
21.));
#11043=CARTESIAN_POINT('Ctrl Pts',(-10.7276339231608,-17.2629318816279,
0.));
#11044=CARTESIAN_POINT('Ctrl Pts',(-10.7276339231608,-17.2629318816279,
21.));
#11045=CARTESIAN_POINT('Ctrl Pts',(-10.6875226650217,-17.2338514174708,
0.));
#11046=CARTESIAN_POINT('Ctrl Pts',(-10.6875226650217,-17.2338514174708,
21.));
#11047=CARTESIAN_POINT('Ctrl Pts',(-10.6476672831754,-17.2045545572011,
0.));
#11048=CARTESIAN_POINT('Ctrl Pts',(-10.6476672831754,-17.2045545572011,
21.));
#11049=CARTESIAN_POINT('Ctrl Pts',(-10.6080729180997,-17.1750388395657,
0.));
#11050=CARTESIAN_POINT('Ctrl Pts',(-10.6080729180997,-17.1750388395657,
21.));
#11051=CARTESIAN_POINT('Ctrl Pts',(-10.5687434234512,-17.1453027387554,
0.));
#11052=CARTESIAN_POINT('Ctrl Pts',(-10.5687434234512,-17.1453027387554,
21.));
#11053=CARTESIAN_POINT('Ctrl Pts',(-10.5296803023445,-17.1153464189932,
0.));
#11054=CARTESIAN_POINT('Ctrl Pts',(-10.5296803023445,-17.1153464189932,
21.));
#11055=CARTESIAN_POINT('Ctrl Pts',(-10.4908835057575,-17.0851711712016,
0.));
#11056=CARTESIAN_POINT('Ctrl Pts',(-10.4908835057575,-17.0851711712016,
21.));
#11057=CARTESIAN_POINT('Ctrl Pts',(-10.452353435089,-17.0547779975888,0.));
#11058=CARTESIAN_POINT('Ctrl Pts',(-10.452353435089,-17.0547779975888,21.));
#11059=CARTESIAN_POINT('Ctrl Pts',(-10.4140927470882,-17.0241663361802,
0.));
#11060=CARTESIAN_POINT('Ctrl Pts',(-10.4140927470882,-17.0241663361802,
21.));
#11061=CARTESIAN_POINT('Ctrl Pts',(-10.3761078860454,-16.9933329788855,
0.));
#11062=CARTESIAN_POINT('Ctrl Pts',(-10.3761078860454,-16.9933329788855,
21.));
#11063=CARTESIAN_POINT('Ctrl Pts',(-10.3384116178624,-16.9622702798438,
0.));
#11064=CARTESIAN_POINT('Ctrl Pts',(-10.3384116178624,-16.9622702798438,
21.));
#11065=CARTESIAN_POINT('Ctrl Pts',(-10.3010210756062,-16.9309675442425,
0.));
#11066=CARTESIAN_POINT('Ctrl Pts',(-10.3010210756062,-16.9309675442425,
21.));
#11067=CARTESIAN_POINT('Ctrl Pts',(-10.2639532144219,-16.8994142530447,
0.));
#11068=CARTESIAN_POINT('Ctrl Pts',(-10.2639532144219,-16.8994142530447,
21.));
#11069=CARTESIAN_POINT('Ctrl Pts',(-10.2272206796636,-16.8676029947679,
0.));
#11070=CARTESIAN_POINT('Ctrl Pts',(-10.2272206796636,-16.8676029947679,
21.));
#11071=CARTESIAN_POINT('Ctrl Pts',(-10.1908283166713,-16.8355319435838,
0.));
#11072=CARTESIAN_POINT('Ctrl Pts',(-10.1908283166713,-16.8355319435838,
21.));
#11073=CARTESIAN_POINT('Ctrl Pts',(-10.1547673397274,-16.8032089941901,
0.));
#11074=CARTESIAN_POINT('Ctrl Pts',(-10.1547673397274,-16.8032089941901,
21.));
#11075=CARTESIAN_POINT('Ctrl Pts',(-10.1190207721353,-16.7706479198888,
0.));
#11076=CARTESIAN_POINT('Ctrl Pts',(-10.1190207721353,-16.7706479198888,
21.));
#11077=CARTESIAN_POINT('Ctrl Pts',(-10.0835742491038,-16.7378607357337,
0.));
#11078=CARTESIAN_POINT('Ctrl Pts',(-10.0835742491038,-16.7378607357337,
21.));
#11079=CARTESIAN_POINT('Ctrl Pts',(-10.0484259314257,-16.7048506904207,
0.));
#11080=CARTESIAN_POINT('Ctrl Pts',(-10.0484259314257,-16.7048506904207,
21.));
#11081=CARTESIAN_POINT('Ctrl Pts',(-10.0135950379525,-16.6716062376277,
0.));
#11082=CARTESIAN_POINT('Ctrl Pts',(-10.0135950379525,-16.6716062376277,
21.));
#11083=CARTESIAN_POINT('Ctrl Pts',(-9.97913546489641,-16.6380914029057,
0.));
#11084=CARTESIAN_POINT('Ctrl Pts',(-9.97913546489641,-16.6380914029057,
21.));
#11085=CARTESIAN_POINT('Ctrl Pts',(-9.9451214271291,-16.6042559779574,0.));
#11086=CARTESIAN_POINT('Ctrl Pts',(-9.9451214271291,-16.6042559779574,21.));
#11087=CARTESIAN_POINT('Ctrl Pts',(-9.91162317616649,-16.5700527532381,
0.));
#11088=CARTESIAN_POINT('Ctrl Pts',(-9.91162317616649,-16.5700527532381,
21.));
#11089=CARTESIAN_POINT('Ctrl Pts',(-9.8786843754698,-16.5354535643506,0.));
#11090=CARTESIAN_POINT('Ctrl Pts',(-9.8786843754698,-16.5354535643506,21.));
#11091=CARTESIAN_POINT('Ctrl Pts',(-9.84630229363522,-16.5004633692332,
0.));
#11092=CARTESIAN_POINT('Ctrl Pts',(-9.84630229363522,-16.5004633692332,
21.));
#11093=CARTESIAN_POINT('Ctrl Pts',(-9.81439757053279,-16.4651416449558,
0.));
#11094=CARTESIAN_POINT('Ctrl Pts',(-9.81439757053279,-16.4651416449558,
21.));
#11095=CARTESIAN_POINT('Ctrl Pts',(-9.78285689698057,-16.4295725710378,
0.));
#11096=CARTESIAN_POINT('Ctrl Pts',(-9.78285689698057,-16.4295725710378,
21.));
#11097=CARTESIAN_POINT('Ctrl Pts',(-9.75159288382685,-16.3938231282759,
0.));
#11098=CARTESIAN_POINT('Ctrl Pts',(-9.75159288382685,-16.3938231282759,
21.));
#11099=CARTESIAN_POINT('Ctrl Pts',(-9.72060002001012,-16.3579039682519,
0.));
#11100=CARTESIAN_POINT('Ctrl Pts',(-9.72060002001012,-16.3579039682519,
21.));
#11101=CARTESIAN_POINT('Ctrl Pts',(-9.69000797146315,-16.3217321000366,
0.));
#11102=CARTESIAN_POINT('Ctrl Pts',(-9.69000797146315,-16.3217321000366,
21.));
#11103=CARTESIAN_POINT('Ctrl Pts',(-9.66014786078746,-16.2850845948324,
0.));
#11104=CARTESIAN_POINT('Ctrl Pts',(-9.66014786078746,-16.2850845948324,
21.));
#11105=CARTESIAN_POINT('Ctrl Pts',(-9.63146315443273,-16.2476599387841,
0.));
#11106=CARTESIAN_POINT('Ctrl Pts',(-9.63146315443273,-16.2476599387841,
21.));
#11107=CARTESIAN_POINT('Ctrl Pts',(-9.60981421781524,-16.2168537871666,
0.));
#11108=CARTESIAN_POINT('Ctrl Pts',(-9.60981421781524,-16.2168537871666,
21.));
#11109=CARTESIAN_POINT('Ctrl Pts',(-9.59446643316597,-16.1931534965272,
0.));
#11110=CARTESIAN_POINT('Ctrl Pts',(-9.59446643316597,-16.1931534965272,
21.));
#11111=CARTESIAN_POINT('Ctrl Pts',(-9.58464985151483,-16.1770747160769,
0.));
#11112=CARTESIAN_POINT('Ctrl Pts',(-9.58464985151483,-16.1770747160769,
21.));
#11113=CARTESIAN_POINT('Ctrl Pts',(-9.57984538049455,-16.1689656784104,
0.));
#11114=CARTESIAN_POINT('Ctrl Pts',(-9.57984538049455,-16.1689656784104,
21.));
#11115=CARTESIAN_POINT('',(-12.3627494547114,-18.1978687191669,0.));
#11116=CARTESIAN_POINT('Ctrl Pts',(-9.57984538049455,-16.1689656784104,
0.));
#11117=CARTESIAN_POINT('Ctrl Pts',(-9.58464985151483,-16.1770747160769,
0.));
#11118=CARTESIAN_POINT('Ctrl Pts',(-9.59446643316597,-16.1931534965272,
0.));
#11119=CARTESIAN_POINT('Ctrl Pts',(-9.60981421781524,-16.2168537871666,
0.));
#11120=CARTESIAN_POINT('Ctrl Pts',(-9.63146315443273,-16.2476599387841,
0.));
#11121=CARTESIAN_POINT('Ctrl Pts',(-9.66014786078746,-16.2850845948324,
0.));
#11122=CARTESIAN_POINT('Ctrl Pts',(-9.69000797146315,-16.3217321000366,
0.));
#11123=CARTESIAN_POINT('Ctrl Pts',(-9.72060002001012,-16.3579039682519,
0.));
#11124=CARTESIAN_POINT('Ctrl Pts',(-9.75159288382685,-16.3938231282759,
0.));
#11125=CARTESIAN_POINT('Ctrl Pts',(-9.78285689698057,-16.4295725710378,
0.));
#11126=CARTESIAN_POINT('Ctrl Pts',(-9.81439757053279,-16.4651416449558,
0.));
#11127=CARTESIAN_POINT('Ctrl Pts',(-9.84630229363522,-16.5004633692332,
0.));
#11128=CARTESIAN_POINT('Ctrl Pts',(-9.8786843754698,-16.5354535643506,0.));
#11129=CARTESIAN_POINT('Ctrl Pts',(-9.91162317616649,-16.5700527532381,
0.));
#11130=CARTESIAN_POINT('Ctrl Pts',(-9.9451214271291,-16.6042559779574,0.));
#11131=CARTESIAN_POINT('Ctrl Pts',(-9.97913546489641,-16.6380914029057,
0.));
#11132=CARTESIAN_POINT('Ctrl Pts',(-10.0135950379525,-16.6716062376277,
0.));
#11133=CARTESIAN_POINT('Ctrl Pts',(-10.0484259314257,-16.7048506904207,
0.));
#11134=CARTESIAN_POINT('Ctrl Pts',(-10.0835742491038,-16.7378607357337,
0.));
#11135=CARTESIAN_POINT('Ctrl Pts',(-10.1190207721353,-16.7706479198888,
0.));
#11136=CARTESIAN_POINT('Ctrl Pts',(-10.1547673397274,-16.8032089941901,
0.));
#11137=CARTESIAN_POINT('Ctrl Pts',(-10.1908283166713,-16.8355319435838,
0.));
#11138=CARTESIAN_POINT('Ctrl Pts',(-10.2272206796636,-16.8676029947679,
0.));
#11139=CARTESIAN_POINT('Ctrl Pts',(-10.2639532144219,-16.8994142530447,
0.));
#11140=CARTESIAN_POINT('Ctrl Pts',(-10.3010210756062,-16.9309675442425,
0.));
#11141=CARTESIAN_POINT('Ctrl Pts',(-10.3384116178624,-16.9622702798438,
0.));
#11142=CARTESIAN_POINT('Ctrl Pts',(-10.3761078860454,-16.9933329788855,
0.));
#11143=CARTESIAN_POINT('Ctrl Pts',(-10.4140927470882,-17.0241663361802,
0.));
#11144=CARTESIAN_POINT('Ctrl Pts',(-10.452353435089,-17.0547779975888,0.));
#11145=CARTESIAN_POINT('Ctrl Pts',(-10.4908835057575,-17.0851711712016,
0.));
#11146=CARTESIAN_POINT('Ctrl Pts',(-10.5296803023445,-17.1153464189932,
0.));
#11147=CARTESIAN_POINT('Ctrl Pts',(-10.5687434234512,-17.1453027387554,
0.));
#11148=CARTESIAN_POINT('Ctrl Pts',(-10.6080729180997,-17.1750388395657,
0.));
#11149=CARTESIAN_POINT('Ctrl Pts',(-10.6476672831754,-17.2045545572011,
0.));
#11150=CARTESIAN_POINT('Ctrl Pts',(-10.6875226650217,-17.2338514174708,
0.));
#11151=CARTESIAN_POINT('Ctrl Pts',(-10.7276339231608,-17.2629318816279,
0.));
#11152=CARTESIAN_POINT('Ctrl Pts',(-10.7679952591482,-17.2917988998581,
0.));
#11153=CARTESIAN_POINT('Ctrl Pts',(-10.8086009632423,-17.3204553814537,
0.));
#11154=CARTESIAN_POINT('Ctrl Pts',(-10.8494462423128,-17.3489036079991,
0.));
#11155=CARTESIAN_POINT('Ctrl Pts',(-10.8905275295837,-17.377145012528,0.));
#11156=CARTESIAN_POINT('Ctrl Pts',(-10.9318420203801,-17.4051805054129,
0.));
#11157=CARTESIAN_POINT('Ctrl Pts',(-10.9733873885115,-17.4330106728622,
0.));
#11158=CARTESIAN_POINT('Ctrl Pts',(-11.0151614525642,-17.460636011184,0.));
#11159=CARTESIAN_POINT('Ctrl Pts',(-11.0571618040371,-17.4880571878157,
0.));
#11160=CARTESIAN_POINT('Ctrl Pts',(-11.0993856581394,-17.5152751467292,
0.));
#11161=CARTESIAN_POINT('Ctrl Pts',(-11.1418300507683,-17.5422909714139,
0.));
#11162=CARTESIAN_POINT('Ctrl Pts',(-11.1844919535058,-17.5691058058227,
0.));
#11163=CARTESIAN_POINT('Ctrl Pts',(-11.2273684103051,-17.5957207597803,
0.));
#11164=CARTESIAN_POINT('Ctrl Pts',(-11.2704566868205,-17.6221368072528,
0.));
#11165=CARTESIAN_POINT('Ctrl Pts',(-11.3137543310722,-17.6483547422688,
0.));
#11166=CARTESIAN_POINT('Ctrl Pts',(-11.3572590796967,-17.674375235974,0.));
#11167=CARTESIAN_POINT('Ctrl Pts',(-11.4009687970126,-17.700198872213,0.));
#11168=CARTESIAN_POINT('Ctrl Pts',(-11.4448814046804,-17.725826190457,0.));
#11169=CARTESIAN_POINT('Ctrl Pts',(-11.4889948016216,-17.7512577332768,
0.));
#11170=CARTESIAN_POINT('Ctrl Pts',(-11.5333068279911,-17.7764940721306,
0.));
#11171=CARTESIAN_POINT('Ctrl Pts',(-11.5778153222435,-17.8015357852426,
0.));
#11172=CARTESIAN_POINT('Ctrl Pts',(-11.6225181583564,-17.8263834470057,
0.));
#11173=CARTESIAN_POINT('Ctrl Pts',(-11.6674132861792,-17.8510376144926,
0.));
#11174=CARTESIAN_POINT('Ctrl Pts',(-11.7124987772363,-17.8754988158862,
0.));
#11175=CARTESIAN_POINT('Ctrl Pts',(-11.7577728408871,-17.8997675418752,
0.));
#11176=CARTESIAN_POINT('Ctrl Pts',(-11.8032337607271,-17.9238442458356,
0.));
#11177=CARTESIAN_POINT('Ctrl Pts',(-11.8488798430201,-17.9477293432951,
0.));
#11178=CARTESIAN_POINT('Ctrl Pts',(-11.8947093631895,-17.9714232133203,
0.));
#11179=CARTESIAN_POINT('Ctrl Pts',(-11.9407205019619,-17.9949261997754,
0.));
#11180=CARTESIAN_POINT('Ctrl Pts',(-11.986911314246,-18.0182386160553,0.));
#11181=CARTESIAN_POINT('Ctrl Pts',(-12.0332798395991,-18.0413607600052,
0.));
#11182=CARTESIAN_POINT('Ctrl Pts',(-12.0798241915081,-18.0642929289333,
0.));
#11183=CARTESIAN_POINT('Ctrl Pts',(-12.1265426519718,-18.0870354350128,
0.));
#11184=CARTESIAN_POINT('Ctrl Pts',(-12.1734337668195,-18.109588624154,0.));
#11185=CARTESIAN_POINT('Ctrl Pts',(-12.2299089600472,-18.1364257412858,
0.));
#11186=CARTESIAN_POINT('Ctrl Pts',(-12.2771850498068,-18.1585543320743,
0.));
#11187=CARTESIAN_POINT('Ctrl Pts',(-12.3151419520839,-18.1761067306718,
0.));
#11188=CARTESIAN_POINT('Ctrl Pts',(-12.3436860694314,-18.1891864723772,
0.));
#11189=CARTESIAN_POINT('Ctrl Pts',(-12.3627494547115,-18.1978687191668,
0.));
#11190=CARTESIAN_POINT('',(-12.3627494547114,-18.1978687191669,13.));
#11191=CARTESIAN_POINT('Ctrl Pts',(-12.3627494547115,-18.1978687191668,
13.));
#11192=CARTESIAN_POINT('Ctrl Pts',(-12.2689088964153,-18.1551298837072,
13.));
#11193=CARTESIAN_POINT('Ctrl Pts',(-12.1760519707549,-18.111299637656,13.));
#11194=CARTESIAN_POINT('Ctrl Pts',(-12.0842021157222,-18.0663670681848,
13.));
#11195=CARTESIAN_POINT('Ctrl Pts',(-11.9320029094011,-17.9919118454842,
13.));
#11196=CARTESIAN_POINT('Ctrl Pts',(-11.7825824042094,-17.9144310022929,
13.));
#11197=CARTESIAN_POINT('Ctrl Pts',(-11.6362239728201,-17.8338669529311,
13.));
#11198=CARTESIAN_POINT('Ctrl Pts',(-11.523724298462,-17.7719406994714,13.));
#11199=CARTESIAN_POINT('Ctrl Pts',(-11.4130324604454,-17.708190453754,13.));
#11200=CARTESIAN_POINT('Ctrl Pts',(-11.3042990938976,-17.6425762029941,
13.));
#11201=CARTESIAN_POINT('Ctrl Pts',(-11.1872502400868,-17.571944040219,13.));
#11202=CARTESIAN_POINT('Ctrl Pts',(-11.0724652191949,-17.499154807149,13.));
#11203=CARTESIAN_POINT('Ctrl Pts',(-10.9601920980076,-17.4241207695605,
13.));
#11204=CARTESIAN_POINT('Ctrl Pts',(-10.8980346540897,-17.3825798919753,
13.));
#11205=CARTESIAN_POINT('Ctrl Pts',(-10.8366430107889,-17.3403540655037,
13.));
#11206=CARTESIAN_POINT('Ctrl Pts',(-10.7760628634082,-17.2974271318847,
13.));
#11207=CARTESIAN_POINT('Ctrl Pts',(-10.71768544558,-17.2560610466519,13.));
#11208=CARTESIAN_POINT('Ctrl Pts',(-10.6600671046061,-17.2140399833079,
13.));
#11209=CARTESIAN_POINT('Ctrl Pts',(-10.6032772242041,-17.1713305004863,
13.));
#11210=CARTESIAN_POINT('Ctrl Pts',(-10.5541933587631,-17.1344164148599,
13.));
#11211=CARTESIAN_POINT('Ctrl Pts',(-10.5057257098335,-17.096989955235,13.));
#11212=CARTESIAN_POINT('Ctrl Pts',(-10.4578814177545,-17.0590571075016,
13.));
#11213=CARTESIAN_POINT('Ctrl Pts',(-10.423545733757,-17.0318344187272,13.));
#11214=CARTESIAN_POINT('Ctrl Pts',(-10.3895287972434,-17.004352569251,13.));
#11215=CARTESIAN_POINT('Ctrl Pts',(-10.3558648787318,-16.9765917293735,
13.));
#11216=CARTESIAN_POINT('Ctrl Pts',(-10.3227491363857,-16.9492829411712,
13.));
#11217=CARTESIAN_POINT('Ctrl Pts',(-10.2899802165512,-16.9217004795811,
13.));
#11218=CARTESIAN_POINT('Ctrl Pts',(-10.257603002843,-16.8938171684013,13.));
#11219=CARTESIAN_POINT('Ctrl Pts',(-10.2295300560935,-16.8696406992028,
13.));
#11220=CARTESIAN_POINT('Ctrl Pts',(-10.2017536135352,-16.8452366235594,
13.));
#11221=CARTESIAN_POINT('Ctrl Pts',(-10.1742626909659,-16.8206160301345,
13.));
#11222=CARTESIAN_POINT('Ctrl Pts',(-10.1493622215735,-16.7983154204895,
13.));
#11223=CARTESIAN_POINT('Ctrl Pts',(-10.1246914564006,-16.7758403904972,
13.));
#11224=CARTESIAN_POINT('Ctrl Pts',(-10.1002324979069,-16.7532063442149,
13.));
#11225=CARTESIAN_POINT('Ctrl Pts',(-10.079629563683,-16.7341406196096,13.));
#11226=CARTESIAN_POINT('Ctrl Pts',(-10.0591755003946,-16.7149630708293,
13.));
#11227=CARTESIAN_POINT('Ctrl Pts',(-10.0388873687047,-16.6956634327229,
13.));
#11228=CARTESIAN_POINT('Ctrl Pts',(-10.0095282357399,-16.6677347574757,
13.));
#11229=CARTESIAN_POINT('Ctrl Pts',(-9.98051721208624,-16.6395499070626,
13.));
#11230=CARTESIAN_POINT('Ctrl Pts',(-9.95203577377263,-16.6109867038064,
13.));
#11231=CARTESIAN_POINT('Ctrl Pts',(-9.9348261830604,-16.5937277075416,13.));
#11232=CARTESIAN_POINT('Ctrl Pts',(-9.91781279953151,-16.5763285722608,
13.));
#11233=CARTESIAN_POINT('Ctrl Pts',(-9.90101792991858,-16.5587751451304,
13.));
#11234=CARTESIAN_POINT('Ctrl Pts',(-9.88552833553625,-16.5425859473257,
13.));
#11235=CARTESIAN_POINT('Ctrl Pts',(-9.87022569084434,-16.5262647433908,
13.));
#11236=CARTESIAN_POINT('Ctrl Pts',(-9.85509024411449,-16.5098269904329,
13.));
#11237=CARTESIAN_POINT('Ctrl Pts',(-9.83426990258338,-16.4872151946467,
13.));
#11238=CARTESIAN_POINT('Ctrl Pts',(-9.81375991310154,-16.4643869859202,
13.));
#11239=CARTESIAN_POINT('Ctrl Pts',(-9.7934396802235,-16.4414328801903,13.));
#11240=CARTESIAN_POINT('Ctrl Pts',(-9.7805481624305,-16.4268703865311,13.));
#11241=CARTESIAN_POINT('Ctrl Pts',(-9.76773166757831,-16.4122582103724,
13.));
#11242=CARTESIAN_POINT('Ctrl Pts',(-9.75498419478216,-16.3976025796313,
13.));
#11243=CARTESIAN_POINT('Ctrl Pts',(-9.74354393127652,-16.3844498331849,
13.));
#11244=CARTESIAN_POINT('Ctrl Pts',(-9.73215866496981,-16.3712625079592,
13.));
#11245=CARTESIAN_POINT('Ctrl Pts',(-9.72085751043954,-16.3580219469452,
13.));
#11246=CARTESIAN_POINT('Ctrl Pts',(-9.70897774622862,-16.3441034802572,
13.));
#11247=CARTESIAN_POINT('Ctrl Pts',(-9.69719080116679,-16.330126283354,13.));
#11248=CARTESIAN_POINT('Ctrl Pts',(-9.68558166507924,-16.3160331239166,
13.));
#11249=CARTESIAN_POINT('Ctrl Pts',(-9.66629891585391,-16.292624417431,13.));
#11250=CARTESIAN_POINT('Ctrl Pts',(-9.64751373148189,-16.268891093964,13.));
#11251=CARTESIAN_POINT('Ctrl Pts',(-9.62974342615828,-16.2444806681934,
13.));
#11252=CARTESIAN_POINT('Ctrl Pts',(-9.61994424733045,-16.231019890619,13.));
#11253=CARTESIAN_POINT('Ctrl Pts',(-9.61045478083913,-16.2173524098339,
13.));
#11254=CARTESIAN_POINT('Ctrl Pts',(-9.60133856554245,-16.2034347659916,
13.));
#11255=CARTESIAN_POINT('Ctrl Pts',(-9.59392299464928,-16.1921134806533,
13.));
#11256=CARTESIAN_POINT('Ctrl Pts',(-9.58675434324541,-16.1806266997688,
13.));
#11257=CARTESIAN_POINT('Ctrl Pts',(-9.57984538049455,-16.1689656784104,
13.));
#11258=CARTESIAN_POINT('',(-12.3627494547114,-18.1978687191669,0.));
#11259=CARTESIAN_POINT('Origin',(-3.33073116609659E-12,-4.58435815896522E-12,
0.));
#11260=CARTESIAN_POINT('',(-13.4869019493419,-17.3811241238545,0.));
#11261=CARTESIAN_POINT('Origin',(-3.33073116609659E-12,-4.58435815896522E-12,
0.));
#11262=CARTESIAN_POINT('',(-13.4869019493419,-17.3811241238545,13.));
#11263=CARTESIAN_POINT('Origin',(-3.33073116609659E-12,-4.58435815896522E-12,
13.));
#11264=CARTESIAN_POINT('',(-13.4869019493419,-17.3811241238545,0.));
#11265=CARTESIAN_POINT('Ctrl Pts',(-12.4172651441477,-14.1074595503134,
0.));
#11266=CARTESIAN_POINT('Ctrl Pts',(-12.4172651441477,-14.1074595503134,
21.));
#11267=CARTESIAN_POINT('Ctrl Pts',(-12.4234926340671,-14.1145347042316,
0.));
#11268=CARTESIAN_POINT('Ctrl Pts',(-12.4234926340671,-14.1145347042316,
21.));
#11269=CARTESIAN_POINT('Ctrl Pts',(-12.4357509724316,-14.1288394445866,
0.));
#11270=CARTESIAN_POINT('Ctrl Pts',(-12.4357509724316,-14.1288394445866,
21.));
#11271=CARTESIAN_POINT('Ctrl Pts',(-12.4535485619996,-14.1507598477672,
0.));
#11272=CARTESIAN_POINT('Ctrl Pts',(-12.4535485619996,-14.1507598477672,
21.));
#11273=CARTESIAN_POINT('Ctrl Pts',(-12.4761570639125,-14.1808688343892,
0.));
#11274=CARTESIAN_POINT('Ctrl Pts',(-12.4761570639125,-14.1808688343892,
21.));
#11275=CARTESIAN_POINT('Ctrl Pts',(-12.5028859651751,-14.2197144660135,
0.));
#11276=CARTESIAN_POINT('Ctrl Pts',(-12.5028859651751,-14.2197144660135,
21.));
#11277=CARTESIAN_POINT('Ctrl Pts',(-12.5285125321527,-14.2594378207584,
0.));
#11278=CARTESIAN_POINT('Ctrl Pts',(-12.5285125321527,-14.2594378207584,
21.));
#11279=CARTESIAN_POINT('Ctrl Pts',(-12.5534605602317,-14.2997103098726,
0.));
#11280=CARTESIAN_POINT('Ctrl Pts',(-12.5534605602317,-14.2997103098726,
21.));
#11281=CARTESIAN_POINT('Ctrl Pts',(-12.5780443898087,-14.3402859058353,
0.));
#11282=CARTESIAN_POINT('Ctrl Pts',(-12.5780443898087,-14.3402859058353,
21.));
#11283=CARTESIAN_POINT('Ctrl Pts',(-12.6023830189244,-14.3810669346235,
0.));
#11284=CARTESIAN_POINT('Ctrl Pts',(-12.6023830189244,-14.3810669346235,
21.));
#11285=CARTESIAN_POINT('Ctrl Pts',(-12.626464614311,-14.4220553460485,0.));
#11286=CARTESIAN_POINT('Ctrl Pts',(-12.626464614311,-14.4220553460485,21.));
#11287=CARTESIAN_POINT('Ctrl Pts',(-12.6501984687124,-14.463313553928,0.));
#11288=CARTESIAN_POINT('Ctrl Pts',(-12.6501984687124,-14.463313553928,21.));
#11289=CARTESIAN_POINT('Ctrl Pts',(-12.6734695081852,-14.5049233087958,
0.));
#11290=CARTESIAN_POINT('Ctrl Pts',(-12.6734695081852,-14.5049233087958,
21.));
#11291=CARTESIAN_POINT('Ctrl Pts',(-12.6961966430455,-14.5469417071951,
0.));
#11292=CARTESIAN_POINT('Ctrl Pts',(-12.6961966430455,-14.5469417071951,
21.));
#11293=CARTESIAN_POINT('Ctrl Pts',(-12.7183743139638,-14.5893698147583,
0.));
#11294=CARTESIAN_POINT('Ctrl Pts',(-12.7183743139638,-14.5893698147583,
21.));
#11295=CARTESIAN_POINT('Ctrl Pts',(-12.7400427996251,-14.6321748083434,
0.));
#11296=CARTESIAN_POINT('Ctrl Pts',(-12.7400427996251,-14.6321748083434,
21.));
#11297=CARTESIAN_POINT('Ctrl Pts',(-12.7612687078867,-14.6753044633399,
0.));
#11298=CARTESIAN_POINT('Ctrl Pts',(-12.7612687078867,-14.6753044633399,
21.));
#11299=CARTESIAN_POINT('Ctrl Pts',(-12.7821227233337,-14.7187037124277,
0.));
#11300=CARTESIAN_POINT('Ctrl Pts',(-12.7821227233337,-14.7187037124277,
21.));
#11301=CARTESIAN_POINT('Ctrl Pts',(-12.8026557145457,-14.7623324139791,
0.));
#11302=CARTESIAN_POINT('Ctrl Pts',(-12.8026557145457,-14.7623324139791,
21.));
#11303=CARTESIAN_POINT('Ctrl Pts',(-12.8228846016791,-14.8061758577898,
0.));
#11304=CARTESIAN_POINT('Ctrl Pts',(-12.8228846016791,-14.8061758577898,
21.));
#11305=CARTESIAN_POINT('Ctrl Pts',(-12.8428057266944,-14.8502347891476,
0.));
#11306=CARTESIAN_POINT('Ctrl Pts',(-12.8428057266944,-14.8502347891476,
21.));
#11307=CARTESIAN_POINT('Ctrl Pts',(-12.8624032236317,-14.8945191569251,
0.));
#11308=CARTESIAN_POINT('Ctrl Pts',(-12.8624032236317,-14.8945191569251,
21.));
#11309=CARTESIAN_POINT('Ctrl Pts',(-12.8816587472147,-14.9390408507356,
0.));
#11310=CARTESIAN_POINT('Ctrl Pts',(-12.8816587472147,-14.9390408507356,
21.));
#11311=CARTESIAN_POINT('Ctrl Pts',(-12.9005620742036,-14.9838057866976,
0.));
#11312=CARTESIAN_POINT('Ctrl Pts',(-12.9005620742036,-14.9838057866976,
21.));
#11313=CARTESIAN_POINT('Ctrl Pts',(-12.9191164383568,-15.0288099208306,
0.));
#11314=CARTESIAN_POINT('Ctrl Pts',(-12.9191164383568,-15.0288099208306,
21.));
#11315=CARTESIAN_POINT('Ctrl Pts',(-12.9373327960422,-15.0740435169624,
0.));
#11316=CARTESIAN_POINT('Ctrl Pts',(-12.9373327960422,-15.0740435169624,
21.));
#11317=CARTESIAN_POINT('Ctrl Pts',(-12.9552263908864,-15.1194937003528,
0.));
#11318=CARTESIAN_POINT('Ctrl Pts',(-12.9552263908864,-15.1194937003528,
21.));
#11319=CARTESIAN_POINT('Ctrl Pts',(-12.9728126886697,-15.1651474813659,
0.));
#11320=CARTESIAN_POINT('Ctrl Pts',(-12.9728126886697,-15.1651474813659,
21.));
#11321=CARTESIAN_POINT('Ctrl Pts',(-12.9901029059182,-15.2109950816083,
0.));
#11322=CARTESIAN_POINT('Ctrl Pts',(-12.9901029059182,-15.2109950816083,
21.));
#11323=CARTESIAN_POINT('Ctrl Pts',(-13.0071020851025,-15.2570313635503,
0.));
#11324=CARTESIAN_POINT('Ctrl Pts',(-13.0071020851025,-15.2570313635503,
21.));
#11325=CARTESIAN_POINT('Ctrl Pts',(-13.0238115816728,-15.3032539741328,
0.));
#11326=CARTESIAN_POINT('Ctrl Pts',(-13.0238115816728,-15.3032539741328,
21.));
#11327=CARTESIAN_POINT('Ctrl Pts',(-13.0402305665115,-15.3496622219036,
0.));
#11328=CARTESIAN_POINT('Ctrl Pts',(-13.0402305665115,-15.3496622219036,
21.));
#11329=CARTESIAN_POINT('Ctrl Pts',(-13.0563577967298,-15.3962557545684,
0.));
#11330=CARTESIAN_POINT('Ctrl Pts',(-13.0563577967298,-15.3962557545684,
21.));
#11331=CARTESIAN_POINT('Ctrl Pts',(-13.0721935806302,-15.4430330918328,
0.));
#11332=CARTESIAN_POINT('Ctrl Pts',(-13.0721935806302,-15.4430330918328,
21.));
#11333=CARTESIAN_POINT('Ctrl Pts',(-13.087740560189,-15.4899910401523,0.));
#11334=CARTESIAN_POINT('Ctrl Pts',(-13.087740560189,-15.4899910401523,21.));
#11335=CARTESIAN_POINT('Ctrl Pts',(-13.1030026646917,-15.5371254712111,
0.));
#11336=CARTESIAN_POINT('Ctrl Pts',(-13.1030026646917,-15.5371254712111,
21.));
#11337=CARTESIAN_POINT('Ctrl Pts',(-13.1179844917497,-15.5844317820184,
0.));
#11338=CARTESIAN_POINT('Ctrl Pts',(-13.1179844917497,-15.5844317820184,
21.));
#11339=CARTESIAN_POINT('Ctrl Pts',(-13.1326905726717,-15.6319054413079,
0.));
#11340=CARTESIAN_POINT('Ctrl Pts',(-13.1326905726717,-15.6319054413079,
21.));
#11341=CARTESIAN_POINT('Ctrl Pts',(-13.147124558532,-15.6795425955901,0.));
#11342=CARTESIAN_POINT('Ctrl Pts',(-13.147124558532,-15.6795425955901,21.));
#11343=CARTESIAN_POINT('Ctrl Pts',(-13.161288914421,-15.7273402954914,0.));
#11344=CARTESIAN_POINT('Ctrl Pts',(-13.161288914421,-15.7273402954914,21.));
#11345=CARTESIAN_POINT('Ctrl Pts',(-13.1751853728467,-15.7752961549278,
0.));
#11346=CARTESIAN_POINT('Ctrl Pts',(-13.1751853728467,-15.7752961549278,
21.));
#11347=CARTESIAN_POINT('Ctrl Pts',(-13.1888152101588,-15.8234081427091,
0.));
#11348=CARTESIAN_POINT('Ctrl Pts',(-13.1888152101588,-15.8234081427091,
21.));
#11349=CARTESIAN_POINT('Ctrl Pts',(-13.2021795724682,-15.8716743375555,
0.));
#11350=CARTESIAN_POINT('Ctrl Pts',(-13.2021795724682,-15.8716743375555,
21.));
#11351=CARTESIAN_POINT('Ctrl Pts',(-13.2152798388134,-15.9200926550954,
0.));
#11352=CARTESIAN_POINT('Ctrl Pts',(-13.2152798388134,-15.9200926550954,
21.));
#11353=CARTESIAN_POINT('Ctrl Pts',(-13.2281177675127,-15.9686607385389,
0.));
#11354=CARTESIAN_POINT('Ctrl Pts',(-13.2281177675127,-15.9686607385389,
21.));
#11355=CARTESIAN_POINT('Ctrl Pts',(-13.240695304984,-16.0173761036734,0.));
#11356=CARTESIAN_POINT('Ctrl Pts',(-13.240695304984,-16.0173761036734,21.));
#11357=CARTESIAN_POINT('Ctrl Pts',(-13.2530144750236,-16.0662362238032,
0.));
#11358=CARTESIAN_POINT('Ctrl Pts',(-13.2530144750236,-16.0662362238032,
21.));
#11359=CARTESIAN_POINT('Ctrl Pts',(-13.2650772466062,-16.1152386305152,
0.));
#11360=CARTESIAN_POINT('Ctrl Pts',(-13.2650772466062,-16.1152386305152,
21.));
#11361=CARTESIAN_POINT('Ctrl Pts',(-13.2768853909882,-16.1643810242643,
0.));
#11362=CARTESIAN_POINT('Ctrl Pts',(-13.2768853909882,-16.1643810242643,
21.));
#11363=CARTESIAN_POINT('Ctrl Pts',(-13.2884404210388,-16.2136613184475,
0.));
#11364=CARTESIAN_POINT('Ctrl Pts',(-13.2884404210388,-16.2136613184475,
21.));
#11365=CARTESIAN_POINT('Ctrl Pts',(-13.2997436744733,-16.2630775678735,
0.));
#11366=CARTESIAN_POINT('Ctrl Pts',(-13.2997436744733,-16.2630775678735,
21.));
#11367=CARTESIAN_POINT('Ctrl Pts',(-13.3107963665229,-16.3126279218067,
0.));
#11368=CARTESIAN_POINT('Ctrl Pts',(-13.3107963665229,-16.3126279218067,
21.));
#11369=CARTESIAN_POINT('Ctrl Pts',(-13.3215996524974,-16.3623105703343,
0.));
#11370=CARTESIAN_POINT('Ctrl Pts',(-13.3215996524974,-16.3623105703343,
21.));
#11371=CARTESIAN_POINT('Ctrl Pts',(-13.3321546976812,-16.4121236828756,
0.));
#11372=CARTESIAN_POINT('Ctrl Pts',(-13.3321546976812,-16.4121236828756,
21.));
#11373=CARTESIAN_POINT('Ctrl Pts',(-13.3424627129921,-16.4620653818862,
0.));
#11374=CARTESIAN_POINT('Ctrl Pts',(-13.3424627129921,-16.4620653818862,
21.));
#11375=CARTESIAN_POINT('Ctrl Pts',(-13.3525249163084,-16.5121337902953,
0.));
#11376=CARTESIAN_POINT('Ctrl Pts',(-13.3525249163084,-16.5121337902953,
21.));
#11377=CARTESIAN_POINT('Ctrl Pts',(-13.3623425108873,-16.5623270636327,
0.));
#11378=CARTESIAN_POINT('Ctrl Pts',(-13.3623425108873,-16.5623270636327,
21.));
#11379=CARTESIAN_POINT('Ctrl Pts',(-13.3719166600676,-16.612643424234,0.));
#11380=CARTESIAN_POINT('Ctrl Pts',(-13.3719166600676,-16.612643424234,21.));
#11381=CARTESIAN_POINT('Ctrl Pts',(-13.381248462113,-16.6630812012276,0.));
#11382=CARTESIAN_POINT('Ctrl Pts',(-13.381248462113,-16.6630812012276,21.));
#11383=CARTESIAN_POINT('Ctrl Pts',(-13.3903389370346,-16.7136388432444,
0.));
#11384=CARTESIAN_POINT('Ctrl Pts',(-13.3903389370346,-16.7136388432444,
21.));
#11385=CARTESIAN_POINT('Ctrl Pts',(-13.3991890464165,-16.7643148579872,
0.));
#11386=CARTESIAN_POINT('Ctrl Pts',(-13.3991890464165,-16.7643148579872,
21.));
#11387=CARTESIAN_POINT('Ctrl Pts',(-13.4077997088426,-16.8151077630226,
0.));
#11388=CARTESIAN_POINT('Ctrl Pts',(-13.4077997088426,-16.8151077630226,
21.));
#11389=CARTESIAN_POINT('Ctrl Pts',(-13.4161718177499,-16.8660160353187,
0.));
#11390=CARTESIAN_POINT('Ctrl Pts',(-13.4161718177499,-16.8660160353187,
21.));
#11391=CARTESIAN_POINT('Ctrl Pts',(-13.4243062623592,-16.9170380509036,
0.));
#11392=CARTESIAN_POINT('Ctrl Pts',(-13.4243062623592,-16.9170380509036,
21.));
#11393=CARTESIAN_POINT('Ctrl Pts',(-13.432203941793,-16.9681720567298,0.));
#11394=CARTESIAN_POINT('Ctrl Pts',(-13.432203941793,-16.9681720567298,21.));
#11395=CARTESIAN_POINT('Ctrl Pts',(-13.4398657451291,-17.0194162803447,
0.));
#11396=CARTESIAN_POINT('Ctrl Pts',(-13.4398657451291,-17.0194162803447,
21.));
#11397=CARTESIAN_POINT('Ctrl Pts',(-13.4472925380889,-17.0707690194411,
0.));
#11398=CARTESIAN_POINT('Ctrl Pts',(-13.4472925380889,-17.0707690194411,
21.));
#11399=CARTESIAN_POINT('Ctrl Pts',(-13.4544851484583,-17.1222287365697,
0.));
#11400=CARTESIAN_POINT('Ctrl Pts',(-13.4544851484583,-17.1222287365697,
21.));
#11401=CARTESIAN_POINT('Ctrl Pts',(-13.4614443545811,-17.1737941556239,
0.));
#11402=CARTESIAN_POINT('Ctrl Pts',(-13.4614443545811,-17.1737941556239,
21.));
#11403=CARTESIAN_POINT('Ctrl Pts',(-13.4681708717969,-17.2254643437923,
0.));
#11404=CARTESIAN_POINT('Ctrl Pts',(-13.4681708717969,-17.2254643437923,
21.));
#11405=CARTESIAN_POINT('Ctrl Pts',(-13.474665315482,-17.2772386565028,0.));
#11406=CARTESIAN_POINT('Ctrl Pts',(-13.474665315482,-17.2772386565028,21.));
#11407=CARTESIAN_POINT('Ctrl Pts',(-13.4796755969465,-17.3187410868027,
0.));
#11408=CARTESIAN_POINT('Ctrl Pts',(-13.4796755969465,-17.3187410868027,
21.));
#11409=CARTESIAN_POINT('Ctrl Pts',(-13.4833292332349,-17.3499144948292,
0.));
#11410=CARTESIAN_POINT('Ctrl Pts',(-13.4833292332349,-17.3499144948292,
21.));
#11411=CARTESIAN_POINT('Ctrl Pts',(-13.485718750657,-17.3707174645609,0.));
#11412=CARTESIAN_POINT('Ctrl Pts',(-13.485718750657,-17.3707174645609,21.));
#11413=CARTESIAN_POINT('Ctrl Pts',(-13.4869019493419,-17.3811241238545,
0.));
#11414=CARTESIAN_POINT('Ctrl Pts',(-13.4869019493419,-17.3811241238545,
21.));
#11415=CARTESIAN_POINT('Ctrl Pts',(-12.4172651441477,-14.1074595503134,
0.));
#11416=CARTESIAN_POINT('Ctrl Pts',(-12.4234926340671,-14.1145347042316,
0.));
#11417=CARTESIAN_POINT('Ctrl Pts',(-12.4357509724316,-14.1288394445866,
0.));
#11418=CARTESIAN_POINT('Ctrl Pts',(-12.4535485619996,-14.1507598477672,
0.));
#11419=CARTESIAN_POINT('Ctrl Pts',(-12.4761570639125,-14.1808688343892,
0.));
#11420=CARTESIAN_POINT('Ctrl Pts',(-12.5028859651751,-14.2197144660135,
0.));
#11421=CARTESIAN_POINT('Ctrl Pts',(-12.5285125321527,-14.2594378207584,
0.));
#11422=CARTESIAN_POINT('Ctrl Pts',(-12.5534605602317,-14.2997103098726,
0.));
#11423=CARTESIAN_POINT('Ctrl Pts',(-12.5780443898087,-14.3402859058353,
0.));
#11424=CARTESIAN_POINT('Ctrl Pts',(-12.6023830189244,-14.3810669346235,
0.));
#11425=CARTESIAN_POINT('Ctrl Pts',(-12.626464614311,-14.4220553460485,0.));
#11426=CARTESIAN_POINT('Ctrl Pts',(-12.6501984687124,-14.463313553928,0.));
#11427=CARTESIAN_POINT('Ctrl Pts',(-12.6734695081852,-14.5049233087958,
0.));
#11428=CARTESIAN_POINT('Ctrl Pts',(-12.6961966430455,-14.5469417071951,
0.));
#11429=CARTESIAN_POINT('Ctrl Pts',(-12.7183743139638,-14.5893698147583,
0.));
#11430=CARTESIAN_POINT('Ctrl Pts',(-12.7400427996251,-14.6321748083434,
0.));
#11431=CARTESIAN_POINT('Ctrl Pts',(-12.7612687078867,-14.6753044633399,
0.));
#11432=CARTESIAN_POINT('Ctrl Pts',(-12.7821227233337,-14.7187037124277,
0.));
#11433=CARTESIAN_POINT('Ctrl Pts',(-12.8026557145457,-14.7623324139791,
0.));
#11434=CARTESIAN_POINT('Ctrl Pts',(-12.8228846016791,-14.8061758577898,
0.));
#11435=CARTESIAN_POINT('Ctrl Pts',(-12.8428057266944,-14.8502347891476,
0.));
#11436=CARTESIAN_POINT('Ctrl Pts',(-12.8624032236317,-14.8945191569251,
0.));
#11437=CARTESIAN_POINT('Ctrl Pts',(-12.8816587472147,-14.9390408507356,
0.));
#11438=CARTESIAN_POINT('Ctrl Pts',(-12.9005620742036,-14.9838057866976,
0.));
#11439=CARTESIAN_POINT('Ctrl Pts',(-12.9191164383568,-15.0288099208306,
0.));
#11440=CARTESIAN_POINT('Ctrl Pts',(-12.9373327960422,-15.0740435169624,
0.));
#11441=CARTESIAN_POINT('Ctrl Pts',(-12.9552263908864,-15.1194937003528,
0.));
#11442=CARTESIAN_POINT('Ctrl Pts',(-12.9728126886697,-15.1651474813659,
0.));
#11443=CARTESIAN_POINT('Ctrl Pts',(-12.9901029059182,-15.2109950816083,
0.));
#11444=CARTESIAN_POINT('Ctrl Pts',(-13.0071020851025,-15.2570313635503,
0.));
#11445=CARTESIAN_POINT('Ctrl Pts',(-13.0238115816728,-15.3032539741328,
0.));
#11446=CARTESIAN_POINT('Ctrl Pts',(-13.0402305665115,-15.3496622219036,
0.));
#11447=CARTESIAN_POINT('Ctrl Pts',(-13.0563577967298,-15.3962557545684,
0.));
#11448=CARTESIAN_POINT('Ctrl Pts',(-13.0721935806302,-15.4430330918328,
0.));
#11449=CARTESIAN_POINT('Ctrl Pts',(-13.087740560189,-15.4899910401523,0.));
#11450=CARTESIAN_POINT('Ctrl Pts',(-13.1030026646917,-15.5371254712111,
0.));
#11451=CARTESIAN_POINT('Ctrl Pts',(-13.1179844917497,-15.5844317820184,
0.));
#11452=CARTESIAN_POINT('Ctrl Pts',(-13.1326905726717,-15.6319054413079,
0.));
#11453=CARTESIAN_POINT('Ctrl Pts',(-13.147124558532,-15.6795425955901,0.));
#11454=CARTESIAN_POINT('Ctrl Pts',(-13.161288914421,-15.7273402954914,0.));
#11455=CARTESIAN_POINT('Ctrl Pts',(-13.1751853728467,-15.7752961549278,
0.));
#11456=CARTESIAN_POINT('Ctrl Pts',(-13.1888152101588,-15.8234081427091,
0.));
#11457=CARTESIAN_POINT('Ctrl Pts',(-13.2021795724682,-15.8716743375555,
0.));
#11458=CARTESIAN_POINT('Ctrl Pts',(-13.2152798388134,-15.9200926550954,
0.));
#11459=CARTESIAN_POINT('Ctrl Pts',(-13.2281177675127,-15.9686607385389,
0.));
#11460=CARTESIAN_POINT('Ctrl Pts',(-13.240695304984,-16.0173761036734,0.));
#11461=CARTESIAN_POINT('Ctrl Pts',(-13.2530144750236,-16.0662362238032,
0.));
#11462=CARTESIAN_POINT('Ctrl Pts',(-13.2650772466062,-16.1152386305152,
0.));
#11463=CARTESIAN_POINT('Ctrl Pts',(-13.2768853909882,-16.1643810242643,
0.));
#11464=CARTESIAN_POINT('Ctrl Pts',(-13.2884404210388,-16.2136613184475,
0.));
#11465=CARTESIAN_POINT('Ctrl Pts',(-13.2997436744733,-16.2630775678735,
0.));
#11466=CARTESIAN_POINT('Ctrl Pts',(-13.3107963665229,-16.3126279218067,
0.));
#11467=CARTESIAN_POINT('Ctrl Pts',(-13.3215996524974,-16.3623105703343,
0.));
#11468=CARTESIAN_POINT('Ctrl Pts',(-13.3321546976812,-16.4121236828756,
0.));
#11469=CARTESIAN_POINT('Ctrl Pts',(-13.3424627129921,-16.4620653818862,
0.));
#11470=CARTESIAN_POINT('Ctrl Pts',(-13.3525249163084,-16.5121337902953,
0.));
#11471=CARTESIAN_POINT('Ctrl Pts',(-13.3623425108873,-16.5623270636327,
0.));
#11472=CARTESIAN_POINT('Ctrl Pts',(-13.3719166600676,-16.612643424234,0.));
#11473=CARTESIAN_POINT('Ctrl Pts',(-13.381248462113,-16.6630812012276,0.));
#11474=CARTESIAN_POINT('Ctrl Pts',(-13.3903389370346,-16.7136388432444,
0.));
#11475=CARTESIAN_POINT('Ctrl Pts',(-13.3991890464165,-16.7643148579872,
0.));
#11476=CARTESIAN_POINT('Ctrl Pts',(-13.4077997088426,-16.8151077630226,
0.));
#11477=CARTESIAN_POINT('Ctrl Pts',(-13.4161718177499,-16.8660160353187,
0.));
#11478=CARTESIAN_POINT('Ctrl Pts',(-13.4243062623592,-16.9170380509036,
0.));
#11479=CARTESIAN_POINT('Ctrl Pts',(-13.432203941793,-16.9681720567298,0.));
#11480=CARTESIAN_POINT('Ctrl Pts',(-13.4398657451291,-17.0194162803447,
0.));
#11481=CARTESIAN_POINT('Ctrl Pts',(-13.4472925380889,-17.0707690194411,
0.));
#11482=CARTESIAN_POINT('Ctrl Pts',(-13.4544851484583,-17.1222287365697,
0.));
#11483=CARTESIAN_POINT('Ctrl Pts',(-13.4614443545811,-17.1737941556239,
0.));
#11484=CARTESIAN_POINT('Ctrl Pts',(-13.4695161752401,-17.235798381426,0.));
#11485=CARTESIAN_POINT('Ctrl Pts',(-13.4759526005425,-17.287598725272,0.));
#11486=CARTESIAN_POINT('Ctrl Pts',(-13.4809165957478,-17.3291218739796,
0.));
#11487=CARTESIAN_POINT('Ctrl Pts',(-13.4845355519784,-17.360310805254,0.));
#11488=CARTESIAN_POINT('Ctrl Pts',(-13.4869019493419,-17.3811241238545,
0.));
#11489=CARTESIAN_POINT('Ctrl Pts',(-12.4172651441477,-14.1074595503134,
13.));
#11490=CARTESIAN_POINT('Ctrl Pts',(-12.4277613166149,-14.1193844248164,
13.));
#11491=CARTESIAN_POINT('Ctrl Pts',(-12.4379186757848,-14.1315753314249,
13.));
#11492=CARTESIAN_POINT('Ctrl Pts',(-12.4477599775084,-14.14401474732,13.));
#11493=CARTESIAN_POINT('Ctrl Pts',(-12.45929471922,-14.1585946731696,13.));
#11494=CARTESIAN_POINT('Ctrl Pts',(-12.4703959522577,-14.1735154808295,
13.));
#11495=CARTESIAN_POINT('Ctrl Pts',(-12.4811568677436,-14.1887053040703,
13.));
#11496=CARTESIAN_POINT('Ctrl Pts',(-12.4962979908344,-14.2100781123335,
13.));
#11497=CARTESIAN_POINT('Ctrl Pts',(-12.5107710847127,-14.2319791941756,
13.));
#11498=CARTESIAN_POINT('Ctrl Pts',(-12.5249003586941,-14.254157574695,13.));
#11499=CARTESIAN_POINT('Ctrl Pts',(-12.5342985542355,-14.2689096955178,
13.));
#11500=CARTESIAN_POINT('Ctrl Pts',(-12.5435462296413,-14.2837832480516,
13.));
#11501=CARTESIAN_POINT('Ctrl Pts',(-12.5527146050322,-14.298722508524,13.));
#11502=CARTESIAN_POINT('Ctrl Pts',(-12.5623658230416,-14.3144485290642,
13.));
#11503=CARTESIAN_POINT('Ctrl Pts',(-12.5719298675028,-14.330246820686,13.));
#11504=CARTESIAN_POINT('Ctrl Pts',(-12.5814385821519,-14.3460912752807,
13.));
#11505=CARTESIAN_POINT('Ctrl Pts',(-12.5919985302804,-14.3636874094394,
13.));
#11506=CARTESIAN_POINT('Ctrl Pts',(-12.6024891912727,-14.381341260665,13.));
#11507=CARTESIAN_POINT('Ctrl Pts',(-12.6128991700701,-14.3990589912032,
13.));
#11508=CARTESIAN_POINT('Ctrl Pts',(-12.6285927183677,-14.4257693299403,
13.));
#11509=CARTESIAN_POINT('Ctrl Pts',(-12.6440977931351,-14.452628589856,13.));
#11510=CARTESIAN_POINT('Ctrl Pts',(-12.6592867998067,-14.4797266308813,
13.));
#11511=CARTESIAN_POINT('Ctrl Pts',(-12.6703212810873,-14.4994127652612,
13.));
#11512=CARTESIAN_POINT('Ctrl Pts',(-12.6811863451307,-14.5192269386383,
13.));
#11513=CARTESIAN_POINT('Ctrl Pts',(-12.6918647171384,-14.5391805041508,
13.));
#11514=CARTESIAN_POINT('Ctrl Pts',(-12.7049181125412,-14.5635720293892,
13.));
#11515=CARTESIAN_POINT('Ctrl Pts',(-12.7176935524276,-14.5881710816651,
13.));
#11516=CARTESIAN_POINT('Ctrl Pts',(-12.7302281821981,-14.612947560673,13.));
#11517=CARTESIAN_POINT('Ctrl Pts',(-12.7437676626773,-14.6397102700639,
13.));
#11518=CARTESIAN_POINT('Ctrl Pts',(-12.7570309720221,-14.6666764215902,
13.));
#11519=CARTESIAN_POINT('Ctrl Pts',(-12.7700903554915,-14.6937895363403,
13.));
#11520=CARTESIAN_POINT('Ctrl Pts',(-12.7821467169645,-14.7188202365146,
13.));
#11521=CARTESIAN_POINT('Ctrl Pts',(-12.7940312932614,-14.7439746960234,
13.));
#11522=CARTESIAN_POINT('Ctrl Pts',(-12.8057660290113,-14.7692347187417,
13.));
#11523=CARTESIAN_POINT('Ctrl Pts',(-12.8217082700361,-14.803551756556,13.));
#11524=CARTESIAN_POINT('Ctrl Pts',(-12.8373723698026,-14.8380647951195,
13.));
#11525=CARTESIAN_POINT('Ctrl Pts',(-12.8527323828632,-14.8727890594695,
13.));
#11526=CARTESIAN_POINT('Ctrl Pts',(-12.8675544637349,-14.9062972246235,
13.));
#11527=CARTESIAN_POINT('Ctrl Pts',(-12.8820871276608,-14.9400067536049,
13.));
#11528=CARTESIAN_POINT('Ctrl Pts',(-12.8963159096104,-14.9739251233868,
13.));
#11529=CARTESIAN_POINT('Ctrl Pts',(-12.9156461084266,-15.0200041787641,
13.));
#11530=CARTESIAN_POINT('Ctrl Pts',(-12.9344180544673,-15.0664667162746,
13.));
#11531=CARTESIAN_POINT('Ctrl Pts',(-12.9526968521306,-15.1132567586771,
13.));
#11532=CARTESIAN_POINT('Ctrl Pts',(-12.968763518006,-15.1543841890161,13.));
#11533=CARTESIAN_POINT('Ctrl Pts',(-12.9844546719519,-15.195760575808,13.));
#11534=CARTESIAN_POINT('Ctrl Pts',(-12.9997938464524,-15.2373637638391,
13.));
#11535=CARTESIAN_POINT('Ctrl Pts',(-13.0224075138791,-15.298696963875,13.));
#11536=CARTESIAN_POINT('Ctrl Pts',(-13.0442489122199,-15.3605284720727,
13.));
#11537=CARTESIAN_POINT('Ctrl Pts',(-13.0653151028182,-15.4228468913963,
13.));
#11538=CARTESIAN_POINT('Ctrl Pts',(-13.0919008408175,-15.501493344391,13.));
#11539=CARTESIAN_POINT('Ctrl Pts',(-13.1172560779889,-15.580912148319,13.));
#11540=CARTESIAN_POINT('Ctrl Pts',(-13.1414683121723,-15.6610132193903,
13.));
#11541=CARTESIAN_POINT('Ctrl Pts',(-13.1742656500639,-15.7695162957074,
13.));
#11542=CARTESIAN_POINT('Ctrl Pts',(-13.2049609859192,-15.8792747460898,
13.));
#11543=CARTESIAN_POINT('Ctrl Pts',(-13.2336341230354,-15.9901726544041,
13.));
#11544=CARTESIAN_POINT('Ctrl Pts',(-13.2591969755247,-16.089041043312,13.));
#11545=CARTESIAN_POINT('Ctrl Pts',(-13.2831593506295,-16.1888100042035,
13.));
#11546=CARTESIAN_POINT('Ctrl Pts',(-13.305579935219,-16.2893994149303,13.));
#11547=CARTESIAN_POINT('Ctrl Pts',(-13.3373560692807,-16.4319622721867,
13.));
#11548=CARTESIAN_POINT('Ctrl Pts',(-13.3660302366011,-16.5761757269041,
13.));
#11549=CARTESIAN_POINT('Ctrl Pts',(-13.3917254924233,-16.7218506225541,
13.));
#11550=CARTESIAN_POINT('Ctrl Pts',(-13.4116849587284,-16.8350074321741,
13.));
#11551=CARTESIAN_POINT('Ctrl Pts',(-13.4298451938425,-16.9490507104974,
13.));
#11552=CARTESIAN_POINT('Ctrl Pts',(-13.4462507334689,-17.063896781128,13.));
#11553=CARTESIAN_POINT('Ctrl Pts',(-13.4604427664362,-17.1632473211086,
13.));
#11554=CARTESIAN_POINT('Ctrl Pts',(-13.4733230167208,-17.2631945741556,
13.));
#11555=CARTESIAN_POINT('Ctrl Pts',(-13.4849093843288,-17.363718437608,13.));
#11556=CARTESIAN_POINT('Ctrl Pts',(-13.4855778874423,-17.3695184016672,
13.));
#11557=CARTESIAN_POINT('Ctrl Pts',(-13.4862420757008,-17.3753202971203,
13.));
#11558=CARTESIAN_POINT('Ctrl Pts',(-13.4869019493419,-17.3811241238545,
13.));
#11559=CARTESIAN_POINT('Ctrl Pts',(-17.3811241238545,-13.4869019493419,
0.));
#11560=CARTESIAN_POINT('Ctrl Pts',(-17.3811241238545,-13.4869019493419,
21.));
#11561=CARTESIAN_POINT('Ctrl Pts',(-17.3707174645609,-13.485718750657,0.));
#11562=CARTESIAN_POINT('Ctrl Pts',(-17.3707174645609,-13.485718750657,21.));
#11563=CARTESIAN_POINT('Ctrl Pts',(-17.3499144948292,-13.4833292332349,
0.));
#11564=CARTESIAN_POINT('Ctrl Pts',(-17.3499144948292,-13.4833292332349,
21.));
#11565=CARTESIAN_POINT('Ctrl Pts',(-17.3187410868027,-13.4796755969465,
0.));
#11566=CARTESIAN_POINT('Ctrl Pts',(-17.3187410868027,-13.4796755969465,
21.));
#11567=CARTESIAN_POINT('Ctrl Pts',(-17.2772386565028,-13.474665315482,0.));
#11568=CARTESIAN_POINT('Ctrl Pts',(-17.2772386565028,-13.474665315482,21.));
#11569=CARTESIAN_POINT('Ctrl Pts',(-17.2254643437923,-13.4681708717969,
0.));
#11570=CARTESIAN_POINT('Ctrl Pts',(-17.2254643437923,-13.4681708717969,
21.));
#11571=CARTESIAN_POINT('Ctrl Pts',(-17.173794155624,-13.4614443545811,0.));
#11572=CARTESIAN_POINT('Ctrl Pts',(-17.173794155624,-13.4614443545811,21.));
#11573=CARTESIAN_POINT('Ctrl Pts',(-17.1222287365697,-13.4544851484583,
0.));
#11574=CARTESIAN_POINT('Ctrl Pts',(-17.1222287365697,-13.4544851484583,
21.));
#11575=CARTESIAN_POINT('Ctrl Pts',(-17.0707690194412,-13.4472925380889,
0.));
#11576=CARTESIAN_POINT('Ctrl Pts',(-17.0707690194412,-13.4472925380889,
21.));
#11577=CARTESIAN_POINT('Ctrl Pts',(-17.0194162803447,-13.4398657451291,
0.));
#11578=CARTESIAN_POINT('Ctrl Pts',(-17.0194162803447,-13.4398657451291,
21.));
#11579=CARTESIAN_POINT('Ctrl Pts',(-16.9681720567298,-13.432203941793,0.));
#11580=CARTESIAN_POINT('Ctrl Pts',(-16.9681720567298,-13.432203941793,21.));
#11581=CARTESIAN_POINT('Ctrl Pts',(-16.9170380509036,-13.4243062623592,
0.));
#11582=CARTESIAN_POINT('Ctrl Pts',(-16.9170380509036,-13.4243062623592,
21.));
#11583=CARTESIAN_POINT('Ctrl Pts',(-16.8660160353187,-13.4161718177499,
0.));
#11584=CARTESIAN_POINT('Ctrl Pts',(-16.8660160353187,-13.4161718177499,
21.));
#11585=CARTESIAN_POINT('Ctrl Pts',(-16.8151077630226,-13.4077997088426,
0.));
#11586=CARTESIAN_POINT('Ctrl Pts',(-16.8151077630226,-13.4077997088426,
21.));
#11587=CARTESIAN_POINT('Ctrl Pts',(-16.7643148579873,-13.3991890464165,
0.));
#11588=CARTESIAN_POINT('Ctrl Pts',(-16.7643148579873,-13.3991890464165,
21.));
#11589=CARTESIAN_POINT('Ctrl Pts',(-16.7136388432444,-13.3903389370346,
0.));
#11590=CARTESIAN_POINT('Ctrl Pts',(-16.7136388432444,-13.3903389370346,
21.));
#11591=CARTESIAN_POINT('Ctrl Pts',(-16.6630812012276,-13.381248462113,0.));
#11592=CARTESIAN_POINT('Ctrl Pts',(-16.6630812012276,-13.381248462113,21.));
#11593=CARTESIAN_POINT('Ctrl Pts',(-16.612643424234,-13.3719166600676,0.));
#11594=CARTESIAN_POINT('Ctrl Pts',(-16.612643424234,-13.3719166600676,21.));
#11595=CARTESIAN_POINT('Ctrl Pts',(-16.5623270636327,-13.3623425108873,
0.));
#11596=CARTESIAN_POINT('Ctrl Pts',(-16.5623270636327,-13.3623425108873,
21.));
#11597=CARTESIAN_POINT('Ctrl Pts',(-16.5121337902953,-13.3525249163084,
0.));
#11598=CARTESIAN_POINT('Ctrl Pts',(-16.5121337902953,-13.3525249163084,
21.));
#11599=CARTESIAN_POINT('Ctrl Pts',(-16.4620653818862,-13.3424627129921,
0.));
#11600=CARTESIAN_POINT('Ctrl Pts',(-16.4620653818862,-13.3424627129921,
21.));
#11601=CARTESIAN_POINT('Ctrl Pts',(-16.4121236828756,-13.3321546976812,
0.));
#11602=CARTESIAN_POINT('Ctrl Pts',(-16.4121236828756,-13.3321546976812,
21.));
#11603=CARTESIAN_POINT('Ctrl Pts',(-16.3623105703343,-13.3215996524974,
0.));
#11604=CARTESIAN_POINT('Ctrl Pts',(-16.3623105703343,-13.3215996524974,
21.));
#11605=CARTESIAN_POINT('Ctrl Pts',(-16.3126279218067,-13.3107963665229,
0.));
#11606=CARTESIAN_POINT('Ctrl Pts',(-16.3126279218067,-13.3107963665229,
21.));
#11607=CARTESIAN_POINT('Ctrl Pts',(-16.2630775678735,-13.2997436744733,
0.));
#11608=CARTESIAN_POINT('Ctrl Pts',(-16.2630775678735,-13.2997436744733,
21.));
#11609=CARTESIAN_POINT('Ctrl Pts',(-16.2136613184475,-13.2884404210387,
0.));
#11610=CARTESIAN_POINT('Ctrl Pts',(-16.2136613184475,-13.2884404210387,
21.));
#11611=CARTESIAN_POINT('Ctrl Pts',(-16.1643810242643,-13.2768853909882,
0.));
#11612=CARTESIAN_POINT('Ctrl Pts',(-16.1643810242643,-13.2768853909882,
21.));
#11613=CARTESIAN_POINT('Ctrl Pts',(-16.1152386305152,-13.2650772466062,
0.));
#11614=CARTESIAN_POINT('Ctrl Pts',(-16.1152386305152,-13.2650772466062,
21.));
#11615=CARTESIAN_POINT('Ctrl Pts',(-16.0662362238032,-13.2530144750236,
0.));
#11616=CARTESIAN_POINT('Ctrl Pts',(-16.0662362238032,-13.2530144750236,
21.));
#11617=CARTESIAN_POINT('Ctrl Pts',(-16.0173761036734,-13.240695304984,0.));
#11618=CARTESIAN_POINT('Ctrl Pts',(-16.0173761036734,-13.240695304984,21.));
#11619=CARTESIAN_POINT('Ctrl Pts',(-15.9686607385389,-13.2281177675127,
0.));
#11620=CARTESIAN_POINT('Ctrl Pts',(-15.9686607385389,-13.2281177675127,
21.));
#11621=CARTESIAN_POINT('Ctrl Pts',(-15.9200926550954,-13.2152798388134,
0.));
#11622=CARTESIAN_POINT('Ctrl Pts',(-15.9200926550954,-13.2152798388134,
21.));
#11623=CARTESIAN_POINT('Ctrl Pts',(-15.8716743375555,-13.2021795724682,
0.));
#11624=CARTESIAN_POINT('Ctrl Pts',(-15.8716743375555,-13.2021795724682,
21.));
#11625=CARTESIAN_POINT('Ctrl Pts',(-15.8234081427091,-13.1888152101588,
0.));
#11626=CARTESIAN_POINT('Ctrl Pts',(-15.8234081427091,-13.1888152101588,
21.));
#11627=CARTESIAN_POINT('Ctrl Pts',(-15.7752961549278,-13.1751853728467,
0.));
#11628=CARTESIAN_POINT('Ctrl Pts',(-15.7752961549278,-13.1751853728467,
21.));
#11629=CARTESIAN_POINT('Ctrl Pts',(-15.7273402954914,-13.161288914421,0.));
#11630=CARTESIAN_POINT('Ctrl Pts',(-15.7273402954914,-13.161288914421,21.));
#11631=CARTESIAN_POINT('Ctrl Pts',(-15.6795425955901,-13.147124558532,0.));
#11632=CARTESIAN_POINT('Ctrl Pts',(-15.6795425955901,-13.147124558532,21.));
#11633=CARTESIAN_POINT('Ctrl Pts',(-15.6319054413079,-13.1326905726717,
0.));
#11634=CARTESIAN_POINT('Ctrl Pts',(-15.6319054413079,-13.1326905726717,
21.));
#11635=CARTESIAN_POINT('Ctrl Pts',(-15.5844317820184,-13.1179844917497,
0.));
#11636=CARTESIAN_POINT('Ctrl Pts',(-15.5844317820184,-13.1179844917497,
21.));
#11637=CARTESIAN_POINT('Ctrl Pts',(-15.5371254712111,-13.1030026646917,
0.));
#11638=CARTESIAN_POINT('Ctrl Pts',(-15.5371254712111,-13.1030026646917,
21.));
#11639=CARTESIAN_POINT('Ctrl Pts',(-15.4899910401523,-13.087740560189,0.));
#11640=CARTESIAN_POINT('Ctrl Pts',(-15.4899910401523,-13.087740560189,21.));
#11641=CARTESIAN_POINT('Ctrl Pts',(-15.4430330918328,-13.0721935806302,
0.));
#11642=CARTESIAN_POINT('Ctrl Pts',(-15.4430330918328,-13.0721935806302,
21.));
#11643=CARTESIAN_POINT('Ctrl Pts',(-15.3962557545684,-13.0563577967298,
0.));
#11644=CARTESIAN_POINT('Ctrl Pts',(-15.3962557545684,-13.0563577967298,
21.));
#11645=CARTESIAN_POINT('Ctrl Pts',(-15.3496622219036,-13.0402305665115,
0.));
#11646=CARTESIAN_POINT('Ctrl Pts',(-15.3496622219036,-13.0402305665115,
21.));
#11647=CARTESIAN_POINT('Ctrl Pts',(-15.3032539741328,-13.0238115816728,
0.));
#11648=CARTESIAN_POINT('Ctrl Pts',(-15.3032539741328,-13.0238115816728,
21.));
#11649=CARTESIAN_POINT('Ctrl Pts',(-15.2570313635503,-13.0071020851025,
0.));
#11650=CARTESIAN_POINT('Ctrl Pts',(-15.2570313635503,-13.0071020851025,
21.));
#11651=CARTESIAN_POINT('Ctrl Pts',(-15.2109950816083,-12.9901029059182,
0.));
#11652=CARTESIAN_POINT('Ctrl Pts',(-15.2109950816083,-12.9901029059182,
21.));
#11653=CARTESIAN_POINT('Ctrl Pts',(-15.1651474813659,-12.9728126886697,
0.));
#11654=CARTESIAN_POINT('Ctrl Pts',(-15.1651474813659,-12.9728126886697,
21.));
#11655=CARTESIAN_POINT('Ctrl Pts',(-15.1194937003528,-12.9552263908864,
0.));
#11656=CARTESIAN_POINT('Ctrl Pts',(-15.1194937003528,-12.9552263908864,
21.));
#11657=CARTESIAN_POINT('Ctrl Pts',(-15.0740435169624,-12.9373327960422,
0.));
#11658=CARTESIAN_POINT('Ctrl Pts',(-15.0740435169624,-12.9373327960422,
21.));
#11659=CARTESIAN_POINT('Ctrl Pts',(-15.0288099208306,-12.9191164383568,
0.));
#11660=CARTESIAN_POINT('Ctrl Pts',(-15.0288099208306,-12.9191164383568,
21.));
#11661=CARTESIAN_POINT('Ctrl Pts',(-14.9838057866976,-12.9005620742036,
0.));
#11662=CARTESIAN_POINT('Ctrl Pts',(-14.9838057866976,-12.9005620742036,
21.));
#11663=CARTESIAN_POINT('Ctrl Pts',(-14.9390408507356,-12.8816587472147,
0.));
#11664=CARTESIAN_POINT('Ctrl Pts',(-14.9390408507356,-12.8816587472147,
21.));
#11665=CARTESIAN_POINT('Ctrl Pts',(-14.8945191569251,-12.8624032236317,
0.));
#11666=CARTESIAN_POINT('Ctrl Pts',(-14.8945191569251,-12.8624032236317,
21.));
#11667=CARTESIAN_POINT('Ctrl Pts',(-14.8502347891476,-12.8428057266944,
0.));
#11668=CARTESIAN_POINT('Ctrl Pts',(-14.8502347891476,-12.8428057266944,
21.));
#11669=CARTESIAN_POINT('Ctrl Pts',(-14.8061758577898,-12.8228846016791,
0.));
#11670=CARTESIAN_POINT('Ctrl Pts',(-14.8061758577898,-12.8228846016791,
21.));
#11671=CARTESIAN_POINT('Ctrl Pts',(-14.7623324139791,-12.8026557145457,
0.));
#11672=CARTESIAN_POINT('Ctrl Pts',(-14.7623324139791,-12.8026557145457,
21.));
#11673=CARTESIAN_POINT('Ctrl Pts',(-14.7187037124277,-12.7821227233337,
0.));
#11674=CARTESIAN_POINT('Ctrl Pts',(-14.7187037124277,-12.7821227233337,
21.));
#11675=CARTESIAN_POINT('Ctrl Pts',(-14.6753044633399,-12.7612687078867,
0.));
#11676=CARTESIAN_POINT('Ctrl Pts',(-14.6753044633399,-12.7612687078867,
21.));
#11677=CARTESIAN_POINT('Ctrl Pts',(-14.6321748083434,-12.7400427996251,
0.));
#11678=CARTESIAN_POINT('Ctrl Pts',(-14.6321748083434,-12.7400427996251,
21.));
#11679=CARTESIAN_POINT('Ctrl Pts',(-14.5893698147583,-12.7183743139638,
0.));
#11680=CARTESIAN_POINT('Ctrl Pts',(-14.5893698147583,-12.7183743139638,
21.));
#11681=CARTESIAN_POINT('Ctrl Pts',(-14.5469417071952,-12.6961966430455,
0.));
#11682=CARTESIAN_POINT('Ctrl Pts',(-14.5469417071952,-12.6961966430455,
21.));
#11683=CARTESIAN_POINT('Ctrl Pts',(-14.5049233087958,-12.6734695081852,
0.));
#11684=CARTESIAN_POINT('Ctrl Pts',(-14.5049233087958,-12.6734695081852,
21.));
#11685=CARTESIAN_POINT('Ctrl Pts',(-14.463313553928,-12.6501984687124,0.));
#11686=CARTESIAN_POINT('Ctrl Pts',(-14.463313553928,-12.6501984687124,21.));
#11687=CARTESIAN_POINT('Ctrl Pts',(-14.4220553460485,-12.626464614311,0.));
#11688=CARTESIAN_POINT('Ctrl Pts',(-14.4220553460485,-12.626464614311,21.));
#11689=CARTESIAN_POINT('Ctrl Pts',(-14.3810669346235,-12.6023830189244,
0.));
#11690=CARTESIAN_POINT('Ctrl Pts',(-14.3810669346235,-12.6023830189244,
21.));
#11691=CARTESIAN_POINT('Ctrl Pts',(-14.3402859058353,-12.5780443898087,
0.));
#11692=CARTESIAN_POINT('Ctrl Pts',(-14.3402859058353,-12.5780443898087,
21.));
#11693=CARTESIAN_POINT('Ctrl Pts',(-14.2997103098726,-12.5534605602317,
0.));
#11694=CARTESIAN_POINT('Ctrl Pts',(-14.2997103098726,-12.5534605602317,
21.));
#11695=CARTESIAN_POINT('Ctrl Pts',(-14.2594378207584,-12.5285125321527,
0.));
#11696=CARTESIAN_POINT('Ctrl Pts',(-14.2594378207584,-12.5285125321527,
21.));
#11697=CARTESIAN_POINT('Ctrl Pts',(-14.2197144660135,-12.502885965175,0.));
#11698=CARTESIAN_POINT('Ctrl Pts',(-14.2197144660135,-12.502885965175,21.));
#11699=CARTESIAN_POINT('Ctrl Pts',(-14.1808688343892,-12.4761570639125,
0.));
#11700=CARTESIAN_POINT('Ctrl Pts',(-14.1808688343892,-12.4761570639125,
21.));
#11701=CARTESIAN_POINT('Ctrl Pts',(-14.1507598477672,-12.4535485619996,
0.));
#11702=CARTESIAN_POINT('Ctrl Pts',(-14.1507598477672,-12.4535485619996,
21.));
#11703=CARTESIAN_POINT('Ctrl Pts',(-14.1288394445866,-12.4357509724316,
0.));
#11704=CARTESIAN_POINT('Ctrl Pts',(-14.1288394445866,-12.4357509724316,
21.));
#11705=CARTESIAN_POINT('Ctrl Pts',(-14.1145347042316,-12.4234926340671,
0.));
#11706=CARTESIAN_POINT('Ctrl Pts',(-14.1145347042316,-12.4234926340671,
21.));
#11707=CARTESIAN_POINT('Ctrl Pts',(-14.1074595503134,-12.4172651441477,
0.));
#11708=CARTESIAN_POINT('Ctrl Pts',(-14.1074595503134,-12.4172651441477,
21.));
#11709=CARTESIAN_POINT('',(-17.3811241238545,-13.486901949342,0.));
#11710=CARTESIAN_POINT('Ctrl Pts',(-14.1074595503134,-12.4172651441477,
0.));
#11711=CARTESIAN_POINT('Ctrl Pts',(-14.1145347042316,-12.4234926340671,
0.));
#11712=CARTESIAN_POINT('Ctrl Pts',(-14.1288394445866,-12.4357509724316,
0.));
#11713=CARTESIAN_POINT('Ctrl Pts',(-14.1507598477672,-12.4535485619996,
0.));
#11714=CARTESIAN_POINT('Ctrl Pts',(-14.1808688343892,-12.4761570639125,
0.));
#11715=CARTESIAN_POINT('Ctrl Pts',(-14.2197144660135,-12.502885965175,0.));
#11716=CARTESIAN_POINT('Ctrl Pts',(-14.2594378207584,-12.5285125321527,
0.));
#11717=CARTESIAN_POINT('Ctrl Pts',(-14.2997103098726,-12.5534605602317,
0.));
#11718=CARTESIAN_POINT('Ctrl Pts',(-14.3402859058353,-12.5780443898087,
0.));
#11719=CARTESIAN_POINT('Ctrl Pts',(-14.3810669346235,-12.6023830189244,
0.));
#11720=CARTESIAN_POINT('Ctrl Pts',(-14.4220553460485,-12.626464614311,0.));
#11721=CARTESIAN_POINT('Ctrl Pts',(-14.463313553928,-12.6501984687124,0.));
#11722=CARTESIAN_POINT('Ctrl Pts',(-14.5049233087958,-12.6734695081852,
0.));
#11723=CARTESIAN_POINT('Ctrl Pts',(-14.5469417071952,-12.6961966430455,
0.));
#11724=CARTESIAN_POINT('Ctrl Pts',(-14.5893698147583,-12.7183743139638,
0.));
#11725=CARTESIAN_POINT('Ctrl Pts',(-14.6321748083434,-12.7400427996251,
0.));
#11726=CARTESIAN_POINT('Ctrl Pts',(-14.6753044633399,-12.7612687078867,
0.));
#11727=CARTESIAN_POINT('Ctrl Pts',(-14.7187037124277,-12.7821227233337,
0.));
#11728=CARTESIAN_POINT('Ctrl Pts',(-14.7623324139791,-12.8026557145457,
0.));
#11729=CARTESIAN_POINT('Ctrl Pts',(-14.8061758577898,-12.8228846016791,
0.));
#11730=CARTESIAN_POINT('Ctrl Pts',(-14.8502347891476,-12.8428057266944,
0.));
#11731=CARTESIAN_POINT('Ctrl Pts',(-14.8945191569251,-12.8624032236317,
0.));
#11732=CARTESIAN_POINT('Ctrl Pts',(-14.9390408507356,-12.8816587472147,
0.));
#11733=CARTESIAN_POINT('Ctrl Pts',(-14.9838057866976,-12.9005620742036,
0.));
#11734=CARTESIAN_POINT('Ctrl Pts',(-15.0288099208306,-12.9191164383568,
0.));
#11735=CARTESIAN_POINT('Ctrl Pts',(-15.0740435169624,-12.9373327960422,
0.));
#11736=CARTESIAN_POINT('Ctrl Pts',(-15.1194937003528,-12.9552263908864,
0.));
#11737=CARTESIAN_POINT('Ctrl Pts',(-15.1651474813659,-12.9728126886697,
0.));
#11738=CARTESIAN_POINT('Ctrl Pts',(-15.2109950816083,-12.9901029059182,
0.));
#11739=CARTESIAN_POINT('Ctrl Pts',(-15.2570313635503,-13.0071020851025,
0.));
#11740=CARTESIAN_POINT('Ctrl Pts',(-15.3032539741328,-13.0238115816728,
0.));
#11741=CARTESIAN_POINT('Ctrl Pts',(-15.3496622219036,-13.0402305665115,
0.));
#11742=CARTESIAN_POINT('Ctrl Pts',(-15.3962557545684,-13.0563577967298,
0.));
#11743=CARTESIAN_POINT('Ctrl Pts',(-15.4430330918328,-13.0721935806302,
0.));
#11744=CARTESIAN_POINT('Ctrl Pts',(-15.4899910401523,-13.087740560189,0.));
#11745=CARTESIAN_POINT('Ctrl Pts',(-15.5371254712111,-13.1030026646917,
0.));
#11746=CARTESIAN_POINT('Ctrl Pts',(-15.5844317820184,-13.1179844917497,
0.));
#11747=CARTESIAN_POINT('Ctrl Pts',(-15.6319054413079,-13.1326905726717,
0.));
#11748=CARTESIAN_POINT('Ctrl Pts',(-15.6795425955901,-13.147124558532,0.));
#11749=CARTESIAN_POINT('Ctrl Pts',(-15.7273402954914,-13.161288914421,0.));
#11750=CARTESIAN_POINT('Ctrl Pts',(-15.7752961549278,-13.1751853728467,
0.));
#11751=CARTESIAN_POINT('Ctrl Pts',(-15.8234081427091,-13.1888152101588,
0.));
#11752=CARTESIAN_POINT('Ctrl Pts',(-15.8716743375555,-13.2021795724682,
0.));
#11753=CARTESIAN_POINT('Ctrl Pts',(-15.9200926550954,-13.2152798388134,
0.));
#11754=CARTESIAN_POINT('Ctrl Pts',(-15.9686607385389,-13.2281177675127,
0.));
#11755=CARTESIAN_POINT('Ctrl Pts',(-16.0173761036734,-13.240695304984,0.));
#11756=CARTESIAN_POINT('Ctrl Pts',(-16.0662362238032,-13.2530144750236,
0.));
#11757=CARTESIAN_POINT('Ctrl Pts',(-16.1152386305152,-13.2650772466062,
0.));
#11758=CARTESIAN_POINT('Ctrl Pts',(-16.1643810242643,-13.2768853909882,
0.));
#11759=CARTESIAN_POINT('Ctrl Pts',(-16.2136613184475,-13.2884404210387,
0.));
#11760=CARTESIAN_POINT('Ctrl Pts',(-16.2630775678735,-13.2997436744733,
0.));
#11761=CARTESIAN_POINT('Ctrl Pts',(-16.3126279218067,-13.3107963665229,
0.));
#11762=CARTESIAN_POINT('Ctrl Pts',(-16.3623105703343,-13.3215996524974,
0.));
#11763=CARTESIAN_POINT('Ctrl Pts',(-16.4121236828756,-13.3321546976812,
0.));
#11764=CARTESIAN_POINT('Ctrl Pts',(-16.4620653818862,-13.3424627129921,
0.));
#11765=CARTESIAN_POINT('Ctrl Pts',(-16.5121337902953,-13.3525249163084,
0.));
#11766=CARTESIAN_POINT('Ctrl Pts',(-16.5623270636327,-13.3623425108873,
0.));
#11767=CARTESIAN_POINT('Ctrl Pts',(-16.612643424234,-13.3719166600676,0.));
#11768=CARTESIAN_POINT('Ctrl Pts',(-16.6630812012276,-13.381248462113,0.));
#11769=CARTESIAN_POINT('Ctrl Pts',(-16.7136388432444,-13.3903389370346,
0.));
#11770=CARTESIAN_POINT('Ctrl Pts',(-16.7643148579873,-13.3991890464165,
0.));
#11771=CARTESIAN_POINT('Ctrl Pts',(-16.8151077630226,-13.4077997088426,
0.));
#11772=CARTESIAN_POINT('Ctrl Pts',(-16.8660160353187,-13.4161718177499,
0.));
#11773=CARTESIAN_POINT('Ctrl Pts',(-16.9170380509036,-13.4243062623592,
0.));
#11774=CARTESIAN_POINT('Ctrl Pts',(-16.9681720567298,-13.432203941793,0.));
#11775=CARTESIAN_POINT('Ctrl Pts',(-17.0194162803447,-13.4398657451291,
0.));
#11776=CARTESIAN_POINT('Ctrl Pts',(-17.0707690194412,-13.4472925380889,
0.));
#11777=CARTESIAN_POINT('Ctrl Pts',(-17.1222287365697,-13.4544851484583,
0.));
#11778=CARTESIAN_POINT('Ctrl Pts',(-17.173794155624,-13.4614443545811,0.));
#11779=CARTESIAN_POINT('Ctrl Pts',(-17.235798381426,-13.4695161752401,0.));
#11780=CARTESIAN_POINT('Ctrl Pts',(-17.287598725272,-13.4759526005425,0.));
#11781=CARTESIAN_POINT('Ctrl Pts',(-17.3291218739796,-13.4809165957478,
0.));
#11782=CARTESIAN_POINT('Ctrl Pts',(-17.360310805254,-13.4845355519784,0.));
#11783=CARTESIAN_POINT('Ctrl Pts',(-17.3811241238545,-13.4869019493419,
0.));
#11784=CARTESIAN_POINT('',(-17.3811241238545,-13.486901949342,13.));
#11785=CARTESIAN_POINT('Ctrl Pts',(-17.3811241238545,-13.4869019493419,
13.));
#11786=CARTESIAN_POINT('Ctrl Pts',(-17.2786694026925,-13.475253226354,13.));
#11787=CARTESIAN_POINT('Ctrl Pts',(-17.1768129075703,-13.4622625504827,
13.));
#11788=CARTESIAN_POINT('Ctrl Pts',(-17.0755735571127,-13.4479123002588,
13.));
#11789=CARTESIAN_POINT('Ctrl Pts',(-16.9078155768783,-13.4241333152838,
13.));
#11790=CARTESIAN_POINT('Ctrl Pts',(-16.7417653304334,-13.3966181281356,
13.));
#11791=CARTESIAN_POINT('Ctrl Pts',(-16.57767452627,-13.365224404591,13.));
#11792=CARTESIAN_POINT('Ctrl Pts',(-16.4515447134285,-13.341093348038,13.));
#11793=CARTESIAN_POINT('Ctrl Pts',(-16.3265706105421,-13.3146689195875,
13.));
#11794=CARTESIAN_POINT('Ctrl Pts',(-16.2028831155019,-13.2858665160047,
13.));
#11795=CARTESIAN_POINT('Ctrl Pts',(-16.06973651931,-13.2548614253288,13.));
#11796=CARTESIAN_POINT('Ctrl Pts',(-15.9380763844413,-13.221105276728,13.));
#11797=CARTESIAN_POINT('Ctrl Pts',(-15.8081115249869,-13.1844379732027,
13.));
#11798=CARTESIAN_POINT('Ctrl Pts',(-15.7361594390004,-13.1641379552808,
13.));
#11799=CARTESIAN_POINT('Ctrl Pts',(-15.6647240119351,-13.1429498666824,
13.));
#11800=CARTESIAN_POINT('Ctrl Pts',(-15.5938437094451,-13.1208442193483,
13.));
#11801=CARTESIAN_POINT('Ctrl Pts',(-15.5255406814322,-13.0995423541465,
13.));
#11802=CARTESIAN_POINT('Ctrl Pts',(-15.4577571787665,-13.0773830005559,
13.));
#11803=CARTESIAN_POINT('Ctrl Pts',(-15.3905488552889,-13.0543129132427,
13.));
#11804=CARTESIAN_POINT('Ctrl Pts',(-15.33246024466,-13.0343732800281,13.));
#11805=CARTESIAN_POINT('Ctrl Pts',(-15.2747993584962,-13.0137559287927,
13.));
#11806=CARTESIAN_POINT('Ctrl Pts',(-15.2175748374047,-12.9924643459712,
13.));
#11807=CARTESIAN_POINT('Ctrl Pts',(-15.1765073882052,-12.9771843404906,
13.));
#11808=CARTESIAN_POINT('Ctrl Pts',(-15.1356630008116,-12.9615593601525,
13.));
#11809=CARTESIAN_POINT('Ctrl Pts',(-15.0950681407047,-12.9455599556256,
13.));
#11810=CARTESIAN_POINT('Ctrl Pts',(-15.0551343157937,-12.9298210808671,
13.));
#11811=CARTESIAN_POINT('Ctrl Pts',(-15.0154457689919,-12.9137147531571,
13.));
#11812=CARTESIAN_POINT('Ctrl Pts',(-14.9760367892541,-12.8972012565818,
13.));
#11813=CARTESIAN_POINT('Ctrl Pts',(-14.9418668889764,-12.8828830850643,
13.));
#11814=CARTESIAN_POINT('Ctrl Pts',(-14.9079086467,-12.8682568220943,13.));
#11815=CARTESIAN_POINT('Ctrl Pts',(-14.8741550424141,-12.853336407922,13.));
#11816=CARTESIAN_POINT('Ctrl Pts',(-14.8435820222663,-12.8398219364233,
13.));
#11817=CARTESIAN_POINT('Ctrl Pts',(-14.8131735649528,-12.8260705988221,
13.));
#11818=CARTESIAN_POINT('Ctrl Pts',(-14.782917409017,-12.8121025758909,13.));
#11819=CARTESIAN_POINT('Ctrl Pts',(-14.7574312210357,-12.8003366510026,
13.));
#11820=CARTESIAN_POINT('Ctrl Pts',(-14.7320520621591,-12.7884183713523,
13.));
#11821=CARTESIAN_POINT('Ctrl Pts',(-14.7067929859341,-12.7763327021684,
13.));
#11822=CARTESIAN_POINT('Ctrl Pts',(-14.6702403530813,-12.7588434232842,
13.));
#11823=CARTESIAN_POINT('Ctrl Pts',(-14.6339396294117,-12.7410029355977,
13.));
#11824=CARTESIAN_POINT('Ctrl Pts',(-14.5980256539368,-12.7226389620173,
13.));
#11825=CARTESIAN_POINT('Ctrl Pts',(-14.5763250375761,-12.7115427372118,
13.));
#11826=CARTESIAN_POINT('Ctrl Pts',(-14.5547677199977,-12.7002526009286,
13.));
#11827=CARTESIAN_POINT('Ctrl Pts',(-14.533370542697,-12.6887481998661,13.));
#11828=CARTESIAN_POINT('Ctrl Pts',(-14.513636325704,-12.6781379056319,13.));
#11829=CARTESIAN_POINT('Ctrl Pts',(-14.494039116296,-12.6673442954742,13.));
#11830=CARTESIAN_POINT('Ctrl Pts',(-14.4745649059699,-12.656388173598,13.));
#11831=CARTESIAN_POINT('Ctrl Pts',(-14.4477761569858,-12.6413169181342,
13.));
#11832=CARTESIAN_POINT('Ctrl Pts',(-14.4212156950323,-12.6259439377184,
13.));
#11833=CARTESIAN_POINT('Ctrl Pts',(-14.3947967980035,-12.610392584142,13.));
#11834=CARTESIAN_POINT('Ctrl Pts',(-14.3780361779186,-12.6005265277046,
13.));
#11835=CARTESIAN_POINT('Ctrl Pts',(-14.3613315561545,-12.5905900370373,
13.));
#11836=CARTESIAN_POINT('Ctrl Pts',(-14.3446791500623,-12.5805908896179,
13.));
#11837=CARTESIAN_POINT('Ctrl Pts',(-14.3297343907096,-12.5716171202366,
13.));
#11838=CARTESIAN_POINT('Ctrl Pts',(-14.3148312513707,-12.5625934694128,
13.));
#11839=CARTESIAN_POINT('Ctrl Pts',(-14.2999916563209,-12.5534931963782,
13.));
#11840=CARTESIAN_POINT('Ctrl Pts',(-14.2843922864836,-12.543926997017,13.));
#11841=CARTESIAN_POINT('Ctrl Pts',(-14.2688630442666,-12.5342762592095,
13.));
#11842=CARTESIAN_POINT('Ctrl Pts',(-14.2534670740361,-12.5244602884878,
13.));
#11843=CARTESIAN_POINT('Ctrl Pts',(-14.2278944013872,-12.5081559827352,
13.));
#11844=CARTESIAN_POINT('Ctrl Pts',(-14.2026946288704,-12.4913891918921,
13.));
#11845=CARTESIAN_POINT('Ctrl Pts',(-14.1782508275765,-12.4736648236058,
13.));
#11846=CARTESIAN_POINT('Ctrl Pts',(-14.1647716456531,-12.4638909761696,
13.));
#11847=CARTESIAN_POINT('Ctrl Pts',(-14.1515231428601,-12.4538248359232,
13.));
#11848=CARTESIAN_POINT('Ctrl Pts',(-14.1385523184119,-12.443405435509,13.));
#11849=CARTESIAN_POINT('Ctrl Pts',(-14.1280012216313,-12.4349297906026,
13.));
#11850=CARTESIAN_POINT('Ctrl Pts',(-14.1176338183099,-12.4262204477521,
13.));
#11851=CARTESIAN_POINT('Ctrl Pts',(-14.1074595503134,-12.4172651441477,
13.));
#11852=CARTESIAN_POINT('',(-17.3811241238545,-13.486901949342,0.));
#11853=CARTESIAN_POINT('Origin',(-4.58435815896522E-12,-3.33073116609659E-12,
0.));
#11854=CARTESIAN_POINT('',(-18.1978687191668,-12.3627494547115,0.));
#11855=CARTESIAN_POINT('Origin',(-4.58435815896522E-12,-3.33073116609659E-12,
0.));
#11856=CARTESIAN_POINT('',(-18.1978687191668,-12.3627494547115,13.));
#11857=CARTESIAN_POINT('Origin',(-4.58435815896522E-12,-3.33073116609659E-12,
13.));
#11858=CARTESIAN_POINT('',(-18.1978687191668,-12.3627494547115,0.));
#11859=CARTESIAN_POINT('Ctrl Pts',(-16.1689656784104,-9.57984538049455,
0.));
#11860=CARTESIAN_POINT('Ctrl Pts',(-16.1689656784104,-9.57984538049455,
21.));
#11861=CARTESIAN_POINT('Ctrl Pts',(-16.1770747160769,-9.58464985151482,
0.));
#11862=CARTESIAN_POINT('Ctrl Pts',(-16.1770747160769,-9.58464985151482,
21.));
#11863=CARTESIAN_POINT('Ctrl Pts',(-16.1931534965272,-9.59446643316596,
0.));
#11864=CARTESIAN_POINT('Ctrl Pts',(-16.1931534965272,-9.59446643316596,
21.));
#11865=CARTESIAN_POINT('Ctrl Pts',(-16.2168537871666,-9.60981421781524,
0.));
#11866=CARTESIAN_POINT('Ctrl Pts',(-16.2168537871666,-9.60981421781524,
21.));
#11867=CARTESIAN_POINT('Ctrl Pts',(-16.2476599387841,-9.63146315443273,
0.));
#11868=CARTESIAN_POINT('Ctrl Pts',(-16.2476599387841,-9.63146315443273,
21.));
#11869=CARTESIAN_POINT('Ctrl Pts',(-16.2850845948324,-9.66014786078746,
0.));
#11870=CARTESIAN_POINT('Ctrl Pts',(-16.2850845948324,-9.66014786078746,
21.));
#11871=CARTESIAN_POINT('Ctrl Pts',(-16.3217321000366,-9.69000797146315,
0.));
#11872=CARTESIAN_POINT('Ctrl Pts',(-16.3217321000366,-9.69000797146315,
21.));
#11873=CARTESIAN_POINT('Ctrl Pts',(-16.3579039682519,-9.72060002001012,
0.));
#11874=CARTESIAN_POINT('Ctrl Pts',(-16.3579039682519,-9.72060002001012,
21.));
#11875=CARTESIAN_POINT('Ctrl Pts',(-16.3938231282759,-9.75159288382684,
0.));
#11876=CARTESIAN_POINT('Ctrl Pts',(-16.3938231282759,-9.75159288382684,
21.));
#11877=CARTESIAN_POINT('Ctrl Pts',(-16.4295725710378,-9.78285689698057,
0.));
#11878=CARTESIAN_POINT('Ctrl Pts',(-16.4295725710378,-9.78285689698057,
21.));
#11879=CARTESIAN_POINT('Ctrl Pts',(-16.4651416449558,-9.81439757053278,
0.));
#11880=CARTESIAN_POINT('Ctrl Pts',(-16.4651416449558,-9.81439757053278,
21.));
#11881=CARTESIAN_POINT('Ctrl Pts',(-16.5004633692332,-9.84630229363521,
0.));
#11882=CARTESIAN_POINT('Ctrl Pts',(-16.5004633692332,-9.84630229363521,
21.));
#11883=CARTESIAN_POINT('Ctrl Pts',(-16.5354535643506,-9.8786843754698,0.));
#11884=CARTESIAN_POINT('Ctrl Pts',(-16.5354535643506,-9.8786843754698,21.));
#11885=CARTESIAN_POINT('Ctrl Pts',(-16.5700527532381,-9.91162317616648,
0.));
#11886=CARTESIAN_POINT('Ctrl Pts',(-16.5700527532381,-9.91162317616648,
21.));
#11887=CARTESIAN_POINT('Ctrl Pts',(-16.6042559779574,-9.9451214271291,0.));
#11888=CARTESIAN_POINT('Ctrl Pts',(-16.6042559779574,-9.9451214271291,21.));
#11889=CARTESIAN_POINT('Ctrl Pts',(-16.6380914029057,-9.97913546489641,
0.));
#11890=CARTESIAN_POINT('Ctrl Pts',(-16.6380914029057,-9.97913546489641,
21.));
#11891=CARTESIAN_POINT('Ctrl Pts',(-16.6716062376277,-10.0135950379525,
0.));
#11892=CARTESIAN_POINT('Ctrl Pts',(-16.6716062376277,-10.0135950379525,
21.));
#11893=CARTESIAN_POINT('Ctrl Pts',(-16.7048506904207,-10.0484259314257,
0.));
#11894=CARTESIAN_POINT('Ctrl Pts',(-16.7048506904207,-10.0484259314257,
21.));
#11895=CARTESIAN_POINT('Ctrl Pts',(-16.7378607357337,-10.0835742491038,
0.));
#11896=CARTESIAN_POINT('Ctrl Pts',(-16.7378607357337,-10.0835742491038,
21.));
#11897=CARTESIAN_POINT('Ctrl Pts',(-16.7706479198888,-10.1190207721353,
0.));
#11898=CARTESIAN_POINT('Ctrl Pts',(-16.7706479198888,-10.1190207721353,
21.));
#11899=CARTESIAN_POINT('Ctrl Pts',(-16.8032089941901,-10.1547673397274,
0.));
#11900=CARTESIAN_POINT('Ctrl Pts',(-16.8032089941901,-10.1547673397274,
21.));
#11901=CARTESIAN_POINT('Ctrl Pts',(-16.8355319435838,-10.1908283166713,
0.));
#11902=CARTESIAN_POINT('Ctrl Pts',(-16.8355319435838,-10.1908283166713,
21.));
#11903=CARTESIAN_POINT('Ctrl Pts',(-16.8676029947679,-10.2272206796636,
0.));
#11904=CARTESIAN_POINT('Ctrl Pts',(-16.8676029947679,-10.2272206796636,
21.));
#11905=CARTESIAN_POINT('Ctrl Pts',(-16.8994142530447,-10.2639532144219,
0.));
#11906=CARTESIAN_POINT('Ctrl Pts',(-16.8994142530447,-10.2639532144219,
21.));
#11907=CARTESIAN_POINT('Ctrl Pts',(-16.9309675442426,-10.3010210756062,
0.));
#11908=CARTESIAN_POINT('Ctrl Pts',(-16.9309675442426,-10.3010210756062,
21.));
#11909=CARTESIAN_POINT('Ctrl Pts',(-16.9622702798438,-10.3384116178624,
0.));
#11910=CARTESIAN_POINT('Ctrl Pts',(-16.9622702798438,-10.3384116178624,
21.));
#11911=CARTESIAN_POINT('Ctrl Pts',(-16.9933329788855,-10.3761078860454,
0.));
#11912=CARTESIAN_POINT('Ctrl Pts',(-16.9933329788855,-10.3761078860454,
21.));
#11913=CARTESIAN_POINT('Ctrl Pts',(-17.0241663361802,-10.4140927470882,
0.));
#11914=CARTESIAN_POINT('Ctrl Pts',(-17.0241663361802,-10.4140927470882,
21.));
#11915=CARTESIAN_POINT('Ctrl Pts',(-17.0547779975888,-10.452353435089,0.));
#11916=CARTESIAN_POINT('Ctrl Pts',(-17.0547779975888,-10.452353435089,21.));
#11917=CARTESIAN_POINT('Ctrl Pts',(-17.0851711712016,-10.4908835057575,
0.));
#11918=CARTESIAN_POINT('Ctrl Pts',(-17.0851711712016,-10.4908835057575,
21.));
#11919=CARTESIAN_POINT('Ctrl Pts',(-17.1153464189932,-10.5296803023445,
0.));
#11920=CARTESIAN_POINT('Ctrl Pts',(-17.1153464189932,-10.5296803023445,
21.));
#11921=CARTESIAN_POINT('Ctrl Pts',(-17.1453027387554,-10.5687434234512,
0.));
#11922=CARTESIAN_POINT('Ctrl Pts',(-17.1453027387554,-10.5687434234512,
21.));
#11923=CARTESIAN_POINT('Ctrl Pts',(-17.1750388395657,-10.6080729180997,
0.));
#11924=CARTESIAN_POINT('Ctrl Pts',(-17.1750388395657,-10.6080729180997,
21.));
#11925=CARTESIAN_POINT('Ctrl Pts',(-17.2045545572011,-10.6476672831754,
0.));
#11926=CARTESIAN_POINT('Ctrl Pts',(-17.2045545572011,-10.6476672831754,
21.));
#11927=CARTESIAN_POINT('Ctrl Pts',(-17.2338514174709,-10.6875226650217,
0.));
#11928=CARTESIAN_POINT('Ctrl Pts',(-17.2338514174709,-10.6875226650217,
21.));
#11929=CARTESIAN_POINT('Ctrl Pts',(-17.2629318816279,-10.7276339231608,
0.));
#11930=CARTESIAN_POINT('Ctrl Pts',(-17.2629318816279,-10.7276339231608,
21.));
#11931=CARTESIAN_POINT('Ctrl Pts',(-17.2917988998581,-10.7679952591482,
0.));
#11932=CARTESIAN_POINT('Ctrl Pts',(-17.2917988998581,-10.7679952591482,
21.));
#11933=CARTESIAN_POINT('Ctrl Pts',(-17.3204553814537,-10.8086009632423,
0.));
#11934=CARTESIAN_POINT('Ctrl Pts',(-17.3204553814537,-10.8086009632423,
21.));
#11935=CARTESIAN_POINT('Ctrl Pts',(-17.3489036079991,-10.8494462423128,
0.));
#11936=CARTESIAN_POINT('Ctrl Pts',(-17.3489036079991,-10.8494462423128,
21.));
#11937=CARTESIAN_POINT('Ctrl Pts',(-17.377145012528,-10.8905275295837,0.));
#11938=CARTESIAN_POINT('Ctrl Pts',(-17.377145012528,-10.8905275295837,21.));
#11939=CARTESIAN_POINT('Ctrl Pts',(-17.405180505413,-10.9318420203801,0.));
#11940=CARTESIAN_POINT('Ctrl Pts',(-17.405180505413,-10.9318420203801,21.));
#11941=CARTESIAN_POINT('Ctrl Pts',(-17.4330106728622,-10.9733873885115,
0.));
#11942=CARTESIAN_POINT('Ctrl Pts',(-17.4330106728622,-10.9733873885115,
21.));
#11943=CARTESIAN_POINT('Ctrl Pts',(-17.460636011184,-11.0151614525642,0.));
#11944=CARTESIAN_POINT('Ctrl Pts',(-17.460636011184,-11.0151614525642,21.));
#11945=CARTESIAN_POINT('Ctrl Pts',(-17.4880571878157,-11.0571618040371,
0.));
#11946=CARTESIAN_POINT('Ctrl Pts',(-17.4880571878157,-11.0571618040371,
21.));
#11947=CARTESIAN_POINT('Ctrl Pts',(-17.5152751467292,-11.0993856581394,
0.));
#11948=CARTESIAN_POINT('Ctrl Pts',(-17.5152751467292,-11.0993856581394,
21.));
#11949=CARTESIAN_POINT('Ctrl Pts',(-17.5422909714139,-11.1418300507683,
0.));
#11950=CARTESIAN_POINT('Ctrl Pts',(-17.5422909714139,-11.1418300507683,
21.));
#11951=CARTESIAN_POINT('Ctrl Pts',(-17.5691058058227,-11.1844919535058,
0.));
#11952=CARTESIAN_POINT('Ctrl Pts',(-17.5691058058227,-11.1844919535058,
21.));
#11953=CARTESIAN_POINT('Ctrl Pts',(-17.5957207597803,-11.2273684103051,
0.));
#11954=CARTESIAN_POINT('Ctrl Pts',(-17.5957207597803,-11.2273684103051,
21.));
#11955=CARTESIAN_POINT('Ctrl Pts',(-17.6221368072528,-11.2704566868205,
0.));
#11956=CARTESIAN_POINT('Ctrl Pts',(-17.6221368072528,-11.2704566868205,
21.));
#11957=CARTESIAN_POINT('Ctrl Pts',(-17.6483547422688,-11.3137543310722,
0.));
#11958=CARTESIAN_POINT('Ctrl Pts',(-17.6483547422688,-11.3137543310722,
21.));
#11959=CARTESIAN_POINT('Ctrl Pts',(-17.674375235974,-11.3572590796967,0.));
#11960=CARTESIAN_POINT('Ctrl Pts',(-17.674375235974,-11.3572590796967,21.));
#11961=CARTESIAN_POINT('Ctrl Pts',(-17.700198872213,-11.4009687970126,0.));
#11962=CARTESIAN_POINT('Ctrl Pts',(-17.700198872213,-11.4009687970126,21.));
#11963=CARTESIAN_POINT('Ctrl Pts',(-17.725826190457,-11.4448814046804,0.));
#11964=CARTESIAN_POINT('Ctrl Pts',(-17.725826190457,-11.4448814046804,21.));
#11965=CARTESIAN_POINT('Ctrl Pts',(-17.7512577332768,-11.4889948016216,
0.));
#11966=CARTESIAN_POINT('Ctrl Pts',(-17.7512577332768,-11.4889948016216,
21.));
#11967=CARTESIAN_POINT('Ctrl Pts',(-17.7764940721306,-11.5333068279911,
0.));
#11968=CARTESIAN_POINT('Ctrl Pts',(-17.7764940721306,-11.5333068279911,
21.));
#11969=CARTESIAN_POINT('Ctrl Pts',(-17.8015357852426,-11.5778153222435,
0.));
#11970=CARTESIAN_POINT('Ctrl Pts',(-17.8015357852426,-11.5778153222435,
21.));
#11971=CARTESIAN_POINT('Ctrl Pts',(-17.8263834470057,-11.6225181583564,
0.));
#11972=CARTESIAN_POINT('Ctrl Pts',(-17.8263834470057,-11.6225181583564,
21.));
#11973=CARTESIAN_POINT('Ctrl Pts',(-17.8510376144926,-11.6674132861792,
0.));
#11974=CARTESIAN_POINT('Ctrl Pts',(-17.8510376144926,-11.6674132861792,
21.));
#11975=CARTESIAN_POINT('Ctrl Pts',(-17.8754988158862,-11.7124987772363,
0.));
#11976=CARTESIAN_POINT('Ctrl Pts',(-17.8754988158862,-11.7124987772363,
21.));
#11977=CARTESIAN_POINT('Ctrl Pts',(-17.8997675418752,-11.7577728408871,
0.));
#11978=CARTESIAN_POINT('Ctrl Pts',(-17.8997675418752,-11.7577728408871,
21.));
#11979=CARTESIAN_POINT('Ctrl Pts',(-17.9238442458356,-11.8032337607271,
0.));
#11980=CARTESIAN_POINT('Ctrl Pts',(-17.9238442458356,-11.8032337607271,
21.));
#11981=CARTESIAN_POINT('Ctrl Pts',(-17.9477293432951,-11.8488798430201,
0.));
#11982=CARTESIAN_POINT('Ctrl Pts',(-17.9477293432951,-11.8488798430201,
21.));
#11983=CARTESIAN_POINT('Ctrl Pts',(-17.9714232133203,-11.8947093631895,
0.));
#11984=CARTESIAN_POINT('Ctrl Pts',(-17.9714232133203,-11.8947093631895,
21.));
#11985=CARTESIAN_POINT('Ctrl Pts',(-17.9949261997754,-11.9407205019619,
0.));
#11986=CARTESIAN_POINT('Ctrl Pts',(-17.9949261997754,-11.9407205019619,
21.));
#11987=CARTESIAN_POINT('Ctrl Pts',(-18.0182386160553,-11.986911314246,0.));
#11988=CARTESIAN_POINT('Ctrl Pts',(-18.0182386160553,-11.986911314246,21.));
#11989=CARTESIAN_POINT('Ctrl Pts',(-18.0413607600052,-12.0332798395991,
0.));
#11990=CARTESIAN_POINT('Ctrl Pts',(-18.0413607600052,-12.0332798395991,
21.));
#11991=CARTESIAN_POINT('Ctrl Pts',(-18.0642929289333,-12.0798241915081,
0.));
#11992=CARTESIAN_POINT('Ctrl Pts',(-18.0642929289333,-12.0798241915081,
21.));
#11993=CARTESIAN_POINT('Ctrl Pts',(-18.0870354350128,-12.1265426519718,
0.));
#11994=CARTESIAN_POINT('Ctrl Pts',(-18.0870354350128,-12.1265426519718,
21.));
#11995=CARTESIAN_POINT('Ctrl Pts',(-18.109588624154,-12.1734337668195,0.));
#11996=CARTESIAN_POINT('Ctrl Pts',(-18.109588624154,-12.1734337668195,21.));
#11997=CARTESIAN_POINT('Ctrl Pts',(-18.1319528884305,-12.2204964278426,
0.));
#11998=CARTESIAN_POINT('Ctrl Pts',(-18.1319528884305,-12.2204964278426,
21.));
#11999=CARTESIAN_POINT('Ctrl Pts',(-18.1541286139166,-12.2677298318549,
0.));
#12000=CARTESIAN_POINT('Ctrl Pts',(-18.1541286139166,-12.2677298318549,
21.));
#12001=CARTESIAN_POINT('Ctrl Pts',(-18.1717186310224,-12.3056527265146,
0.));
#12002=CARTESIAN_POINT('Ctrl Pts',(-18.1717186310224,-12.3056527265146,
21.));
#12003=CARTESIAN_POINT('Ctrl Pts',(-18.1848265584754,-12.3341713636489,
0.));
#12004=CARTESIAN_POINT('Ctrl Pts',(-18.1848265584754,-12.3341713636489,
21.));
#12005=CARTESIAN_POINT('Ctrl Pts',(-18.1935275957711,-12.3532177620787,
0.));
#12006=CARTESIAN_POINT('Ctrl Pts',(-18.1935275957711,-12.3532177620787,
21.));
#12007=CARTESIAN_POINT('Ctrl Pts',(-18.1978687191668,-12.3627494547115,
0.));
#12008=CARTESIAN_POINT('Ctrl Pts',(-18.1978687191668,-12.3627494547115,
21.));
#12009=CARTESIAN_POINT('Ctrl Pts',(-16.1689656784104,-9.57984538049455,
0.));
#12010=CARTESIAN_POINT('Ctrl Pts',(-16.1770747160769,-9.58464985151482,
0.));
#12011=CARTESIAN_POINT('Ctrl Pts',(-16.1931534965272,-9.59446643316596,
0.));
#12012=CARTESIAN_POINT('Ctrl Pts',(-16.2168537871666,-9.60981421781524,
0.));
#12013=CARTESIAN_POINT('Ctrl Pts',(-16.2476599387841,-9.63146315443273,
0.));
#12014=CARTESIAN_POINT('Ctrl Pts',(-16.2850845948324,-9.66014786078746,
0.));
#12015=CARTESIAN_POINT('Ctrl Pts',(-16.3217321000366,-9.69000797146315,
0.));
#12016=CARTESIAN_POINT('Ctrl Pts',(-16.3579039682519,-9.72060002001012,
0.));
#12017=CARTESIAN_POINT('Ctrl Pts',(-16.3938231282759,-9.75159288382684,
0.));
#12018=CARTESIAN_POINT('Ctrl Pts',(-16.4295725710378,-9.78285689698057,
0.));
#12019=CARTESIAN_POINT('Ctrl Pts',(-16.4651416449558,-9.81439757053278,
0.));
#12020=CARTESIAN_POINT('Ctrl Pts',(-16.5004633692332,-9.84630229363521,
0.));
#12021=CARTESIAN_POINT('Ctrl Pts',(-16.5354535643506,-9.8786843754698,0.));
#12022=CARTESIAN_POINT('Ctrl Pts',(-16.5700527532381,-9.91162317616648,
0.));
#12023=CARTESIAN_POINT('Ctrl Pts',(-16.6042559779574,-9.9451214271291,0.));
#12024=CARTESIAN_POINT('Ctrl Pts',(-16.6380914029057,-9.97913546489641,
0.));
#12025=CARTESIAN_POINT('Ctrl Pts',(-16.6716062376277,-10.0135950379525,
0.));
#12026=CARTESIAN_POINT('Ctrl Pts',(-16.7048506904207,-10.0484259314257,
0.));
#12027=CARTESIAN_POINT('Ctrl Pts',(-16.7378607357337,-10.0835742491038,
0.));
#12028=CARTESIAN_POINT('Ctrl Pts',(-16.7706479198888,-10.1190207721353,
0.));
#12029=CARTESIAN_POINT('Ctrl Pts',(-16.8032089941901,-10.1547673397274,
0.));
#12030=CARTESIAN_POINT('Ctrl Pts',(-16.8355319435838,-10.1908283166713,
0.));
#12031=CARTESIAN_POINT('Ctrl Pts',(-16.8676029947679,-10.2272206796636,
0.));
#12032=CARTESIAN_POINT('Ctrl Pts',(-16.8994142530447,-10.2639532144219,
0.));
#12033=CARTESIAN_POINT('Ctrl Pts',(-16.9309675442426,-10.3010210756062,
0.));
#12034=CARTESIAN_POINT('Ctrl Pts',(-16.9622702798438,-10.3384116178624,
0.));
#12035=CARTESIAN_POINT('Ctrl Pts',(-16.9933329788855,-10.3761078860454,
0.));
#12036=CARTESIAN_POINT('Ctrl Pts',(-17.0241663361802,-10.4140927470882,
0.));
#12037=CARTESIAN_POINT('Ctrl Pts',(-17.0547779975888,-10.452353435089,0.));
#12038=CARTESIAN_POINT('Ctrl Pts',(-17.0851711712016,-10.4908835057575,
0.));
#12039=CARTESIAN_POINT('Ctrl Pts',(-17.1153464189932,-10.5296803023445,
0.));
#12040=CARTESIAN_POINT('Ctrl Pts',(-17.1453027387554,-10.5687434234512,
0.));
#12041=CARTESIAN_POINT('Ctrl Pts',(-17.1750388395657,-10.6080729180997,
0.));
#12042=CARTESIAN_POINT('Ctrl Pts',(-17.2045545572011,-10.6476672831754,
0.));
#12043=CARTESIAN_POINT('Ctrl Pts',(-17.2338514174709,-10.6875226650217,
0.));
#12044=CARTESIAN_POINT('Ctrl Pts',(-17.2629318816279,-10.7276339231608,
0.));
#12045=CARTESIAN_POINT('Ctrl Pts',(-17.2917988998581,-10.7679952591482,
0.));
#12046=CARTESIAN_POINT('Ctrl Pts',(-17.3204553814537,-10.8086009632423,
0.));
#12047=CARTESIAN_POINT('Ctrl Pts',(-17.3489036079991,-10.8494462423128,
0.));
#12048=CARTESIAN_POINT('Ctrl Pts',(-17.377145012528,-10.8905275295837,0.));
#12049=CARTESIAN_POINT('Ctrl Pts',(-17.405180505413,-10.9318420203801,0.));
#12050=CARTESIAN_POINT('Ctrl Pts',(-17.4330106728622,-10.9733873885115,
0.));
#12051=CARTESIAN_POINT('Ctrl Pts',(-17.460636011184,-11.0151614525642,0.));
#12052=CARTESIAN_POINT('Ctrl Pts',(-17.4880571878157,-11.0571618040371,
0.));
#12053=CARTESIAN_POINT('Ctrl Pts',(-17.5152751467292,-11.0993856581394,
0.));
#12054=CARTESIAN_POINT('Ctrl Pts',(-17.5422909714139,-11.1418300507683,
0.));
#12055=CARTESIAN_POINT('Ctrl Pts',(-17.5691058058227,-11.1844919535058,
0.));
#12056=CARTESIAN_POINT('Ctrl Pts',(-17.5957207597803,-11.2273684103051,
0.));
#12057=CARTESIAN_POINT('Ctrl Pts',(-17.6221368072528,-11.2704566868205,
0.));
#12058=CARTESIAN_POINT('Ctrl Pts',(-17.6483547422688,-11.3137543310722,
0.));
#12059=CARTESIAN_POINT('Ctrl Pts',(-17.674375235974,-11.3572590796967,0.));
#12060=CARTESIAN_POINT('Ctrl Pts',(-17.700198872213,-11.4009687970126,0.));
#12061=CARTESIAN_POINT('Ctrl Pts',(-17.725826190457,-11.4448814046804,0.));
#12062=CARTESIAN_POINT('Ctrl Pts',(-17.7512577332768,-11.4889948016216,
0.));
#12063=CARTESIAN_POINT('Ctrl Pts',(-17.7764940721306,-11.5333068279911,
0.));
#12064=CARTESIAN_POINT('Ctrl Pts',(-17.8015357852426,-11.5778153222435,
0.));
#12065=CARTESIAN_POINT('Ctrl Pts',(-17.8263834470057,-11.6225181583564,
0.));
#12066=CARTESIAN_POINT('Ctrl Pts',(-17.8510376144926,-11.6674132861792,
0.));
#12067=CARTESIAN_POINT('Ctrl Pts',(-17.8754988158862,-11.7124987772363,
0.));
#12068=CARTESIAN_POINT('Ctrl Pts',(-17.8997675418752,-11.7577728408871,
0.));
#12069=CARTESIAN_POINT('Ctrl Pts',(-17.9238442458356,-11.8032337607271,
0.));
#12070=CARTESIAN_POINT('Ctrl Pts',(-17.9477293432951,-11.8488798430201,
0.));
#12071=CARTESIAN_POINT('Ctrl Pts',(-17.9714232133203,-11.8947093631895,
0.));
#12072=CARTESIAN_POINT('Ctrl Pts',(-17.9949261997754,-11.9407205019619,
0.));
#12073=CARTESIAN_POINT('Ctrl Pts',(-18.0182386160553,-11.986911314246,0.));
#12074=CARTESIAN_POINT('Ctrl Pts',(-18.0413607600052,-12.0332798395991,
0.));
#12075=CARTESIAN_POINT('Ctrl Pts',(-18.0642929289333,-12.0798241915081,
0.));
#12076=CARTESIAN_POINT('Ctrl Pts',(-18.0870354350128,-12.1265426519718,
0.));
#12077=CARTESIAN_POINT('Ctrl Pts',(-18.109588624154,-12.1734337668195,0.));
#12078=CARTESIAN_POINT('Ctrl Pts',(-18.1364257412858,-12.2299089600472,
0.));
#12079=CARTESIAN_POINT('Ctrl Pts',(-18.1585543320743,-12.2771850498068,
0.));
#12080=CARTESIAN_POINT('Ctrl Pts',(-18.1761067306718,-12.3151419520839,
0.));
#12081=CARTESIAN_POINT('Ctrl Pts',(-18.1891864723772,-12.3436860694314,
0.));
#12082=CARTESIAN_POINT('Ctrl Pts',(-18.1978687191668,-12.3627494547115,
0.));
#12083=CARTESIAN_POINT('Ctrl Pts',(-16.1689656784104,-9.57984538049455,
13.));
#12084=CARTESIAN_POINT('Ctrl Pts',(-16.1826331205334,-9.58794311444298,
13.));
#12085=CARTESIAN_POINT('Ctrl Pts',(-16.1960605405031,-9.59639855902712,
13.));
#12086=CARTESIAN_POINT('Ctrl Pts',(-16.209264165571,-9.60518801711085,13.));
#12087=CARTESIAN_POINT('Ctrl Pts',(-16.224739801703,-9.6154899193841,13.));
#12088=CARTESIAN_POINT('Ctrl Pts',(-16.2399084848584,-9.62624998107167,
13.));
#12089=CARTESIAN_POINT('Ctrl Pts',(-16.254836637175,-9.63737105568732,13.));
#12090=CARTESIAN_POINT('Ctrl Pts',(-16.2758412618972,-9.65301893989002,
13.));
#12091=CARTESIAN_POINT('Ctrl Pts',(-16.296373798599,-9.66937567449949,13.));
#12092=CARTESIAN_POINT('Ctrl Pts',(-16.3166650331518,-9.68610238201322,
13.));
#12093=CARTESIAN_POINT('Ctrl Pts',(-16.3301619042985,-9.69722828051063,
13.));
#12094=CARTESIAN_POINT('Ctrl Pts',(-16.3435531467518,-9.70851618070807,
13.));
#12095=CARTESIAN_POINT('Ctrl Pts',(-16.3568892752788,-9.7198910779208,13.));
#12096=CARTESIAN_POINT('Ctrl Pts',(-16.3709277366574,-9.73186502184932,
13.));
#12097=CARTESIAN_POINT('Ctrl Pts',(-16.3849056240572,-9.74393463776872,
13.));
#12098=CARTESIAN_POINT('Ctrl Pts',(-16.3988451548219,-9.75606525513648,
13.));
#12099=CARTESIAN_POINT('Ctrl Pts',(-16.414325766791,-9.76953696975778,13.));
#12100=CARTESIAN_POINT('Ctrl Pts',(-16.4297583183324,-9.78308498747417,
13.));
#12101=CARTESIAN_POINT('Ctrl Pts',(-16.4451338763398,-9.79671869019648,
13.));
#12102=CARTESIAN_POINT('Ctrl Pts',(-16.4683132763075,-9.8172721587789,13.));
#12103=CARTESIAN_POINT('Ctrl Pts',(-16.4913594464712,-9.83802550134249,
13.));
#12104=CARTESIAN_POINT('Ctrl Pts',(-16.5141788054336,-9.85910360864921,
13.));
#12105=CARTESIAN_POINT('Ctrl Pts',(-16.5307565708362,-9.87441639279172,
13.));
#12106=CARTESIAN_POINT('Ctrl Pts',(-16.5472127770975,-9.88990330206224,
13.));
#12107=CARTESIAN_POINT('Ctrl Pts',(-16.5635345032205,-9.90558047214324,
13.));
#12108=CARTESIAN_POINT('Ctrl Pts',(-16.5834864158081,-9.92474447016175,
13.));
#12109=CARTESIAN_POINT('Ctrl Pts',(-16.6032381063718,-9.9441917311001,13.));
#12110=CARTESIAN_POINT('Ctrl Pts',(-16.6228156007807,-9.96388214930656,
13.));
#12111=CARTESIAN_POINT('Ctrl Pts',(-16.6439625439398,-9.9851510689085,13.));
#12112=CARTESIAN_POINT('Ctrl Pts',(-16.6649096998191,-10.006698815053,13.));
#12113=CARTESIAN_POINT('Ctrl Pts',(-16.6857083247995,-10.0284493480904,
13.));
#12114=CARTESIAN_POINT('Ctrl Pts',(-16.7049095176705,-10.0485293380076,
13.));
#12115=CARTESIAN_POINT('Ctrl Pts',(-16.7239855768682,-10.0687801145851,
13.));
#12116=CARTESIAN_POINT('Ctrl Pts',(-16.7429517500628,-10.0891775910162,
13.));
#12117=CARTESIAN_POINT('Ctrl Pts',(-16.7687182701337,-10.1168886100216,
13.));
#12118=CARTESIAN_POINT('Ctrl Pts',(-16.7942808297111,-10.1448719871919,
13.));
#12119=CARTESIAN_POINT('Ctrl Pts',(-16.8196194580034,-10.1731502199822,
13.));
#12120=CARTESIAN_POINT('Ctrl Pts',(-16.844070687064,-10.2004381038963,13.));
#12121=CARTESIAN_POINT('Ctrl Pts',(-16.8683088890975,-10.2280069309447,
13.));
#12122=CARTESIAN_POINT('Ctrl Pts',(-16.8923226175541,-10.2558682820918,
13.));
#12123=CARTESIAN_POINT('Ctrl Pts',(-16.9249459403096,-10.2937187080479,
13.));
#12124=CARTESIAN_POINT('Ctrl Pts',(-16.9571568356211,-10.3321063567812,
13.));
#12125=CARTESIAN_POINT('Ctrl Pts',(-16.9889999235317,-10.3709578724058,
13.));
#12126=CARTESIAN_POINT('Ctrl Pts',(-17.0169893055707,-10.4051075100498,
13.));
#12127=CARTESIAN_POINT('Ctrl Pts',(-17.04469848632,-10.4396099589146,13.));
#12128=CARTESIAN_POINT('Ctrl Pts',(-17.0721430001642,-10.474436876203,13.));
#12129=CARTESIAN_POINT('Ctrl Pts',(-17.112602877017,-10.5257802081583,13.));
#12130=CARTESIAN_POINT('Ctrl Pts',(-17.1524822680152,-10.5778361036082,
13.));
#12131=CARTESIAN_POINT('Ctrl Pts',(-17.1917748564523,-10.6305946314222,
13.));
#12132=CARTESIAN_POINT('Ctrl Pts',(-17.2413624862848,-10.6971764080832,
13.));
#12133=CARTESIAN_POINT('Ctrl Pts',(-17.2900185098528,-10.7648729797973,
13.));
#12134=CARTESIAN_POINT('Ctrl Pts',(-17.3377983051247,-10.8335716334697,
13.));
#12135=CARTESIAN_POINT('Ctrl Pts',(-17.4025197212104,-10.9266292559136,
13.));
#12136=CARTESIAN_POINT('Ctrl Pts',(-17.465629946501,-11.0215303643735,13.));
#12137=CARTESIAN_POINT('Ctrl Pts',(-17.5271690583862,-11.1181400554829,
13.));
#12138=CARTESIAN_POINT('Ctrl Pts',(-17.5820327885162,-11.2042701255893,
13.));
#12139=CARTESIAN_POINT('Ctrl Pts',(-17.6356526662346,-11.2917512652755,
13.));
#12140=CARTESIAN_POINT('Ctrl Pts',(-17.6880597469658,-11.3804891386083,
13.));
#12141=CARTESIAN_POINT('Ctrl Pts',(-17.7623349917623,-11.5062551071101,
13.));
#12142=CARTESIAN_POINT('Ctrl Pts',(-17.8341701535583,-11.6345494475067,
13.));
#12143=CARTESIAN_POINT('Ctrl Pts',(-17.9036238122623,-11.7651542350891,
13.));
#12144=CARTESIAN_POINT('Ctrl Pts',(-17.9575737615728,-11.8666049261148,
13.));
#12145=CARTESIAN_POINT('Ctrl Pts',(-18.0100864746768,-11.9694546915569,
13.));
#12146=CARTESIAN_POINT('Ctrl Pts',(-18.0611784501095,-12.0736101881878,
13.));
#12147=CARTESIAN_POINT('Ctrl Pts',(-18.1053768649439,-12.163712553743,13.));
#12148=CARTESIAN_POINT('Ctrl Pts',(-18.1485120955669,-12.2547877895871,
13.));
#12149=CARTESIAN_POINT('Ctrl Pts',(-18.1905949538241,-12.346811245556,13.));
#12150=CARTESIAN_POINT('Ctrl Pts',(-18.1930230491134,-12.3521208117116,
13.));
#12151=CARTESIAN_POINT('Ctrl Pts',(-18.1954476374973,-12.357433548157,13.));
#12152=CARTESIAN_POINT('Ctrl Pts',(-18.1978687191668,-12.3627494547115,
13.));
#12153=CARTESIAN_POINT('Ctrl Pts',(-20.698113262342,-7.455743247944,0.));
#12154=CARTESIAN_POINT('Ctrl Pts',(-20.698113262342,-7.455743247944,21.));
#12155=CARTESIAN_POINT('Ctrl Pts',(-20.6878503127065,-7.45783379370107,
0.));
#12156=CARTESIAN_POINT('Ctrl Pts',(-20.6878503127065,-7.45783379370107,
21.));
#12157=CARTESIAN_POINT('Ctrl Pts',(-20.6673271112931,-7.46198969876653,
0.));
#12158=CARTESIAN_POINT('Ctrl Pts',(-20.6673271112931,-7.46198969876653,
21.));
#12159=CARTESIAN_POINT('Ctrl Pts',(-20.6365504027501,-7.46814799701905,
0.));
#12160=CARTESIAN_POINT('Ctrl Pts',(-20.6365504027501,-7.46814799701905,
21.));
#12161=CARTESIAN_POINT('Ctrl Pts',(-20.5955309838521,-7.47620789245427,
0.));
#12162=CARTESIAN_POINT('Ctrl Pts',(-20.5955309838521,-7.47620789245427,
21.));
#12163=CARTESIAN_POINT('Ctrl Pts',(-20.5442837929044,-7.48603045196744,
0.));
#12164=CARTESIAN_POINT('Ctrl Pts',(-20.5442837929044,-7.48603045196744,
21.));
#12165=CARTESIAN_POINT('Ctrl Pts',(-20.4930639156161,-7.49560012018405,
0.));
#12166=CARTESIAN_POINT('Ctrl Pts',(-20.4930639156161,-7.49560012018405,
21.));
#12167=CARTESIAN_POINT('Ctrl Pts',(-20.4418717748497,-7.50491611266253,
0.));
#12168=CARTESIAN_POINT('Ctrl Pts',(-20.4418717748497,-7.50491611266253,
21.));
#12169=CARTESIAN_POINT('Ctrl Pts',(-20.3907080367098,-7.51397746081993,
0.));
#12170=CARTESIAN_POINT('Ctrl Pts',(-20.3907080367098,-7.51397746081993,
21.));
#12171=CARTESIAN_POINT('Ctrl Pts',(-20.3395736743243,-7.52278303006887,
0.));
#12172=CARTESIAN_POINT('Ctrl Pts',(-20.3395736743243,-7.52278303006887,
21.));
#12173=CARTESIAN_POINT('Ctrl Pts',(-20.2884698940944,-7.53133155804007,
0.));
#12174=CARTESIAN_POINT('Ctrl Pts',(-20.2884698940944,-7.53133155804007,
21.));
#12175=CARTESIAN_POINT('Ctrl Pts',(-20.2373980474879,-7.53962169534166,
0.));
#12176=CARTESIAN_POINT('Ctrl Pts',(-20.2373980474879,-7.53962169534166,
21.));
#12177=CARTESIAN_POINT('Ctrl Pts',(-20.1863595454674,-7.54765204869254,
0.));
#12178=CARTESIAN_POINT('Ctrl Pts',(-20.1863595454674,-7.54765204869254,
21.));
#12179=CARTESIAN_POINT('Ctrl Pts',(-20.1353557774357,-7.55542122125494,
0.));
#12180=CARTESIAN_POINT('Ctrl Pts',(-20.1353557774357,-7.55542122125494,
21.));
#12181=CARTESIAN_POINT('Ctrl Pts',(-20.0843880130978,-7.5629278654946,0.));
#12182=CARTESIAN_POINT('Ctrl Pts',(-20.0843880130978,-7.5629278654946,21.));
#12183=CARTESIAN_POINT('Ctrl Pts',(-20.0334574248557,-7.57017066105972,
0.));
#12184=CARTESIAN_POINT('Ctrl Pts',(-20.0334574248557,-7.57017066105972,
21.));
#12185=CARTESIAN_POINT('Ctrl Pts',(-19.9825651387294,-7.57714827622806,
0.));
#12186=CARTESIAN_POINT('Ctrl Pts',(-19.9825651387294,-7.57714827622806,
21.));
#12187=CARTESIAN_POINT('Ctrl Pts',(-19.931712276832,-7.58385933533351,0.));
#12188=CARTESIAN_POINT('Ctrl Pts',(-19.931712276832,-7.58385933533351,21.));
#12189=CARTESIAN_POINT('Ctrl Pts',(-19.8808999994024,-7.59030238888852,
0.));
#12190=CARTESIAN_POINT('Ctrl Pts',(-19.8808999994024,-7.59030238888852,
21.));
#12191=CARTESIAN_POINT('Ctrl Pts',(-19.830129556152,-7.59647587605448,0.));
#12192=CARTESIAN_POINT('Ctrl Pts',(-19.830129556152,-7.59647587605448,21.));
#12193=CARTESIAN_POINT('Ctrl Pts',(-19.7794022782484,-7.60237814110186,
0.));
#12194=CARTESIAN_POINT('Ctrl Pts',(-19.7794022782484,-7.60237814110186,
21.));
#12195=CARTESIAN_POINT('Ctrl Pts',(-19.7287195480601,-7.60800746969261,
0.));
#12196=CARTESIAN_POINT('Ctrl Pts',(-19.7287195480601,-7.60800746969261,
21.));
#12197=CARTESIAN_POINT('Ctrl Pts',(-19.6780827744426,-7.61336212350879,
0.));
#12198=CARTESIAN_POINT('Ctrl Pts',(-19.6780827744426,-7.61336212350879,
21.));
#12199=CARTESIAN_POINT('Ctrl Pts',(-19.6274933688524,-7.6184403707059,0.));
#12200=CARTESIAN_POINT('Ctrl Pts',(-19.6274933688524,-7.6184403707059,21.));
#12201=CARTESIAN_POINT('Ctrl Pts',(-19.5769527121826,-7.62324053735219,
0.));
#12202=CARTESIAN_POINT('Ctrl Pts',(-19.5769527121826,-7.62324053735219,
21.));
#12203=CARTESIAN_POINT('Ctrl Pts',(-19.5264621687521,-7.62776096538882,
0.));
#12204=CARTESIAN_POINT('Ctrl Pts',(-19.5264621687521,-7.62776096538882,
21.));
#12205=CARTESIAN_POINT('Ctrl Pts',(-19.4760231231881,-7.63199992715365,
0.));
#12206=CARTESIAN_POINT('Ctrl Pts',(-19.4760231231881,-7.63199992715365,
21.));
#12207=CARTESIAN_POINT('Ctrl Pts',(-19.4256370121006,-7.63595554930653,
0.));
#12208=CARTESIAN_POINT('Ctrl Pts',(-19.4256370121006,-7.63595554930653,
21.));
#12209=CARTESIAN_POINT('Ctrl Pts',(-19.3753053524647,-7.6396257482276,0.));
#12210=CARTESIAN_POINT('Ctrl Pts',(-19.3753053524647,-7.6396257482276,21.));
#12211=CARTESIAN_POINT('Ctrl Pts',(-19.3250297839295,-7.64300812875338,
0.));
#12212=CARTESIAN_POINT('Ctrl Pts',(-19.3250297839295,-7.64300812875338,
21.));
#12213=CARTESIAN_POINT('Ctrl Pts',(-19.2748120456486,-7.64610005549613,
0.));
#12214=CARTESIAN_POINT('Ctrl Pts',(-19.2748120456486,-7.64610005549613,
21.));
#12215=CARTESIAN_POINT('Ctrl Pts',(-19.224653915265,-7.64889882291923,0.));
#12216=CARTESIAN_POINT('Ctrl Pts',(-19.224653915265,-7.64889882291923,21.));
#12217=CARTESIAN_POINT('Ctrl Pts',(-19.1745571539291,-7.65140181220525,
0.));
#12218=CARTESIAN_POINT('Ctrl Pts',(-19.1745571539291,-7.65140181220525,
21.));
#12219=CARTESIAN_POINT('Ctrl Pts',(-19.1245234597312,-7.65360662280608,
0.));
#12220=CARTESIAN_POINT('Ctrl Pts',(-19.1245234597312,-7.65360662280608,
21.));
#12221=CARTESIAN_POINT('Ctrl Pts',(-19.0745543888799,-7.65551129907201,
0.));
#12222=CARTESIAN_POINT('Ctrl Pts',(-19.0745543888799,-7.65551129907201,
21.));
#12223=CARTESIAN_POINT('Ctrl Pts',(-19.0246514144531,-7.65711415727855,
0.));
#12224=CARTESIAN_POINT('Ctrl Pts',(-19.0246514144531,-7.65711415727855,
21.));
#12225=CARTESIAN_POINT('Ctrl Pts',(-18.974816073814,-7.65841335587266,0.));
#12226=CARTESIAN_POINT('Ctrl Pts',(-18.974816073814,-7.65841335587266,21.));
#12227=CARTESIAN_POINT('Ctrl Pts',(-18.9250501008887,-7.65940650980098,
0.));
#12228=CARTESIAN_POINT('Ctrl Pts',(-18.9250501008887,-7.65940650980098,
21.));
#12229=CARTESIAN_POINT('Ctrl Pts',(-18.8753555389435,-7.66009036321663,
0.));
#12230=CARTESIAN_POINT('Ctrl Pts',(-18.8753555389435,-7.66009036321663,
21.));
#12231=CARTESIAN_POINT('Ctrl Pts',(-18.8257349246207,-7.66046025294774,
0.));
#12232=CARTESIAN_POINT('Ctrl Pts',(-18.8257349246207,-7.66046025294774,
21.));
#12233=CARTESIAN_POINT('Ctrl Pts',(-18.7761911671591,-7.6605104692254,0.));
#12234=CARTESIAN_POINT('Ctrl Pts',(-18.7761911671591,-7.6605104692254,21.));
#12235=CARTESIAN_POINT('Ctrl Pts',(-18.7267272235231,-7.66023521705904,
0.));
#12236=CARTESIAN_POINT('Ctrl Pts',(-18.7267272235231,-7.66023521705904,
21.));
#12237=CARTESIAN_POINT('Ctrl Pts',(-18.6773458057584,-7.65962948375621,
0.));
#12238=CARTESIAN_POINT('Ctrl Pts',(-18.6773458057584,-7.65962948375621,
21.));
#12239=CARTESIAN_POINT('Ctrl Pts',(-18.6280491346907,-7.65868976978871,
0.));
#12240=CARTESIAN_POINT('Ctrl Pts',(-18.6280491346907,-7.65868976978871,
21.));
#12241=CARTESIAN_POINT('Ctrl Pts',(-18.5788385228928,-7.65741532450727,
0.));
#12242=CARTESIAN_POINT('Ctrl Pts',(-18.5788385228928,-7.65741532450727,
21.));
#12243=CARTESIAN_POINT('Ctrl Pts',(-18.5297146894905,-7.65580722110436,
0.));
#12244=CARTESIAN_POINT('Ctrl Pts',(-18.5297146894905,-7.65580722110436,
21.));
#12245=CARTESIAN_POINT('Ctrl Pts',(-18.4806785483052,-7.65386603444742,
0.));
#12246=CARTESIAN_POINT('Ctrl Pts',(-18.4806785483052,-7.65386603444742,
21.));
#12247=CARTESIAN_POINT('Ctrl Pts',(-18.4317319183719,-7.65158974829126,
0.));
#12248=CARTESIAN_POINT('Ctrl Pts',(-18.4317319183719,-7.65158974829126,
21.));
#12249=CARTESIAN_POINT('Ctrl Pts',(-18.3828781275628,-7.6489719793775,0.));
#12250=CARTESIAN_POINT('Ctrl Pts',(-18.3828781275628,-7.6489719793775,21.));
#12251=CARTESIAN_POINT('Ctrl Pts',(-18.3341230095852,-7.64599903846601,
0.));
#12252=CARTESIAN_POINT('Ctrl Pts',(-18.3341230095852,-7.64599903846601,
21.));
#12253=CARTESIAN_POINT('Ctrl Pts',(-18.2854741391282,-7.64265220270759,
0.));
#12254=CARTESIAN_POINT('Ctrl Pts',(-18.2854741391282,-7.64265220270759,
21.));
#12255=CARTESIAN_POINT('Ctrl Pts',(-18.2369390502576,-7.63891299603826,
0.));
#12256=CARTESIAN_POINT('Ctrl Pts',(-18.2369390502576,-7.63891299603826,
21.));
#12257=CARTESIAN_POINT('Ctrl Pts',(-18.1885236169197,-7.63476798969016,
0.));
#12258=CARTESIAN_POINT('Ctrl Pts',(-18.1885236169197,-7.63476798969016,
21.));
#12259=CARTESIAN_POINT('Ctrl Pts',(-18.1402306858819,-7.63021285851761,
0.));
#12260=CARTESIAN_POINT('Ctrl Pts',(-18.1402306858819,-7.63021285851761,
21.));
#12261=CARTESIAN_POINT('Ctrl Pts',(-18.0920577897363,-7.62525915358073,
0.));
#12262=CARTESIAN_POINT('Ctrl Pts',(-18.0920577897363,-7.62525915358073,
21.));
#12263=CARTESIAN_POINT('Ctrl Pts',(-18.0439992897906,-7.61992799636654,
0.));
#12264=CARTESIAN_POINT('Ctrl Pts',(-18.0439992897906,-7.61992799636654,
21.));
#12265=CARTESIAN_POINT('Ctrl Pts',(-17.9960506269561,-7.61423755067037,
0.));
#12266=CARTESIAN_POINT('Ctrl Pts',(-17.9960506269561,-7.61423755067037,
21.));
#12267=CARTESIAN_POINT('Ctrl Pts',(-17.9482122228183,-7.60819152580111,
0.));
#12268=CARTESIAN_POINT('Ctrl Pts',(-17.9482122228183,-7.60819152580111,
21.));
#12269=CARTESIAN_POINT('Ctrl Pts',(-17.900492838997,-7.60176928403058,0.));
#12270=CARTESIAN_POINT('Ctrl Pts',(-17.900492838997,-7.60176928403058,21.));
#12271=CARTESIAN_POINT('Ctrl Pts',(-17.8529149331931,-7.59491004201955,
0.));
#12272=CARTESIAN_POINT('Ctrl Pts',(-17.8529149331931,-7.59491004201955,
21.));
#12273=CARTESIAN_POINT('Ctrl Pts',(-17.8055090348024,-7.58752955799498,
0.));
#12274=CARTESIAN_POINT('Ctrl Pts',(-17.8055090348024,-7.58752955799498,
21.));
#12275=CARTESIAN_POINT('Ctrl Pts',(-17.7583042294209,-7.57954834582803,
0.));
#12276=CARTESIAN_POINT('Ctrl Pts',(-17.7583042294209,-7.57954834582803,
21.));
#12277=CARTESIAN_POINT('Ctrl Pts',(-17.7113192869136,-7.57091795530423,
0.));
#12278=CARTESIAN_POINT('Ctrl Pts',(-17.7113192869136,-7.57091795530423,
21.));
#12279=CARTESIAN_POINT('Ctrl Pts',(-17.6645549117314,-7.56164400295862,
0.));
#12280=CARTESIAN_POINT('Ctrl Pts',(-17.6645549117314,-7.56164400295862,
21.));
#12281=CARTESIAN_POINT('Ctrl Pts',(-17.6179818599248,-7.55182125346563,
0.));
#12282=CARTESIAN_POINT('Ctrl Pts',(-17.6179818599248,-7.55182125346563,
21.));
#12283=CARTESIAN_POINT('Ctrl Pts',(-17.5715579419204,-7.54158441095317,
0.));
#12284=CARTESIAN_POINT('Ctrl Pts',(-17.5715579419204,-7.54158441095317,
21.));
#12285=CARTESIAN_POINT('Ctrl Pts',(-17.5252518287336,-7.53103903007863,
0.));
#12286=CARTESIAN_POINT('Ctrl Pts',(-17.5252518287336,-7.53103903007863,
21.));
#12287=CARTESIAN_POINT('Ctrl Pts',(-17.4790653226646,-7.52019696747328,
0.));
#12288=CARTESIAN_POINT('Ctrl Pts',(-17.4790653226646,-7.52019696747328,
21.));
#12289=CARTESIAN_POINT('Ctrl Pts',(-17.4330545448126,-7.50891486634214,
0.));
#12290=CARTESIAN_POINT('Ctrl Pts',(-17.4330545448126,-7.50891486634214,
21.));
#12291=CARTESIAN_POINT('Ctrl Pts',(-17.3873563447297,-7.4968177445175,0.));
#12292=CARTESIAN_POINT('Ctrl Pts',(-17.3873563447297,-7.4968177445175,21.));
#12293=CARTESIAN_POINT('Ctrl Pts',(-17.3421522689127,-7.48340100912745,
0.));
#12294=CARTESIAN_POINT('Ctrl Pts',(-17.3421522689127,-7.48340100912745,
21.));
#12295=CARTESIAN_POINT('Ctrl Pts',(-17.3065305096784,-7.47120323460919,
0.));
#12296=CARTESIAN_POINT('Ctrl Pts',(-17.3065305096784,-7.47120323460919,
21.));
#12297=CARTESIAN_POINT('Ctrl Pts',(-17.2801832097582,-7.4610504981825,0.));
#12298=CARTESIAN_POINT('Ctrl Pts',(-17.2801832097582,-7.4610504981825,21.));
#12299=CARTESIAN_POINT('Ctrl Pts',(-17.2627905583523,-7.45381253347183,
0.));
#12300=CARTESIAN_POINT('Ctrl Pts',(-17.2627905583523,-7.45381253347183,
21.));
#12301=CARTESIAN_POINT('Ctrl Pts',(-17.2541372868972,-7.45007618140238,
0.));
#12302=CARTESIAN_POINT('Ctrl Pts',(-17.2541372868972,-7.45007618140238,
21.));
#12303=CARTESIAN_POINT('',(-20.698113262342,-7.45574324794406,0.));
#12304=CARTESIAN_POINT('Ctrl Pts',(-17.2541372868972,-7.45007618140238,
0.));
#12305=CARTESIAN_POINT('Ctrl Pts',(-17.2627905583523,-7.45381253347183,
0.));
#12306=CARTESIAN_POINT('Ctrl Pts',(-17.2801832097582,-7.4610504981825,0.));
#12307=CARTESIAN_POINT('Ctrl Pts',(-17.3065305096784,-7.47120323460919,
0.));
#12308=CARTESIAN_POINT('Ctrl Pts',(-17.3421522689127,-7.48340100912745,
0.));
#12309=CARTESIAN_POINT('Ctrl Pts',(-17.3873563447297,-7.4968177445175,0.));
#12310=CARTESIAN_POINT('Ctrl Pts',(-17.4330545448126,-7.50891486634214,
0.));
#12311=CARTESIAN_POINT('Ctrl Pts',(-17.4790653226646,-7.52019696747328,
0.));
#12312=CARTESIAN_POINT('Ctrl Pts',(-17.5252518287336,-7.53103903007863,
0.));
#12313=CARTESIAN_POINT('Ctrl Pts',(-17.5715579419204,-7.54158441095317,
0.));
#12314=CARTESIAN_POINT('Ctrl Pts',(-17.6179818599248,-7.55182125346563,
0.));
#12315=CARTESIAN_POINT('Ctrl Pts',(-17.6645549117314,-7.56164400295862,
0.));
#12316=CARTESIAN_POINT('Ctrl Pts',(-17.7113192869136,-7.57091795530423,
0.));
#12317=CARTESIAN_POINT('Ctrl Pts',(-17.7583042294209,-7.57954834582803,
0.));
#12318=CARTESIAN_POINT('Ctrl Pts',(-17.8055090348024,-7.58752955799498,
0.));
#12319=CARTESIAN_POINT('Ctrl Pts',(-17.8529149331931,-7.59491004201955,
0.));
#12320=CARTESIAN_POINT('Ctrl Pts',(-17.900492838997,-7.60176928403058,0.));
#12321=CARTESIAN_POINT('Ctrl Pts',(-17.9482122228183,-7.60819152580111,
0.));
#12322=CARTESIAN_POINT('Ctrl Pts',(-17.9960506269561,-7.61423755067037,
0.));
#12323=CARTESIAN_POINT('Ctrl Pts',(-18.0439992897906,-7.61992799636654,
0.));
#12324=CARTESIAN_POINT('Ctrl Pts',(-18.0920577897363,-7.62525915358073,
0.));
#12325=CARTESIAN_POINT('Ctrl Pts',(-18.1402306858819,-7.63021285851761,
0.));
#12326=CARTESIAN_POINT('Ctrl Pts',(-18.1885236169197,-7.63476798969016,
0.));
#12327=CARTESIAN_POINT('Ctrl Pts',(-18.2369390502576,-7.63891299603826,
0.));
#12328=CARTESIAN_POINT('Ctrl Pts',(-18.2854741391282,-7.64265220270759,
0.));
#12329=CARTESIAN_POINT('Ctrl Pts',(-18.3341230095852,-7.64599903846601,
0.));
#12330=CARTESIAN_POINT('Ctrl Pts',(-18.3828781275628,-7.6489719793775,0.));
#12331=CARTESIAN_POINT('Ctrl Pts',(-18.4317319183719,-7.65158974829126,
0.));
#12332=CARTESIAN_POINT('Ctrl Pts',(-18.4806785483052,-7.65386603444742,
0.));
#12333=CARTESIAN_POINT('Ctrl Pts',(-18.5297146894905,-7.65580722110436,
0.));
#12334=CARTESIAN_POINT('Ctrl Pts',(-18.5788385228928,-7.65741532450727,
0.));
#12335=CARTESIAN_POINT('Ctrl Pts',(-18.6280491346907,-7.65868976978871,
0.));
#12336=CARTESIAN_POINT('Ctrl Pts',(-18.6773458057584,-7.65962948375621,
0.));
#12337=CARTESIAN_POINT('Ctrl Pts',(-18.7267272235231,-7.66023521705904,
0.));
#12338=CARTESIAN_POINT('Ctrl Pts',(-18.7761911671591,-7.6605104692254,0.));
#12339=CARTESIAN_POINT('Ctrl Pts',(-18.8257349246207,-7.66046025294774,
0.));
#12340=CARTESIAN_POINT('Ctrl Pts',(-18.8753555389435,-7.66009036321663,
0.));
#12341=CARTESIAN_POINT('Ctrl Pts',(-18.9250501008887,-7.65940650980098,
0.));
#12342=CARTESIAN_POINT('Ctrl Pts',(-18.974816073814,-7.65841335587266,0.));
#12343=CARTESIAN_POINT('Ctrl Pts',(-19.0246514144531,-7.65711415727855,
0.));
#12344=CARTESIAN_POINT('Ctrl Pts',(-19.0745543888799,-7.65551129907201,
0.));
#12345=CARTESIAN_POINT('Ctrl Pts',(-19.1245234597312,-7.65360662280608,
0.));
#12346=CARTESIAN_POINT('Ctrl Pts',(-19.1745571539291,-7.65140181220525,
0.));
#12347=CARTESIAN_POINT('Ctrl Pts',(-19.224653915265,-7.64889882291923,0.));
#12348=CARTESIAN_POINT('Ctrl Pts',(-19.2748120456486,-7.64610005549613,
0.));
#12349=CARTESIAN_POINT('Ctrl Pts',(-19.3250297839295,-7.64300812875338,
0.));
#12350=CARTESIAN_POINT('Ctrl Pts',(-19.3753053524647,-7.6396257482276,0.));
#12351=CARTESIAN_POINT('Ctrl Pts',(-19.4256370121006,-7.63595554930653,
0.));
#12352=CARTESIAN_POINT('Ctrl Pts',(-19.4760231231881,-7.63199992715365,
0.));
#12353=CARTESIAN_POINT('Ctrl Pts',(-19.5264621687521,-7.62776096538882,
0.));
#12354=CARTESIAN_POINT('Ctrl Pts',(-19.5769527121826,-7.62324053735219,
0.));
#12355=CARTESIAN_POINT('Ctrl Pts',(-19.6274933688524,-7.6184403707059,0.));
#12356=CARTESIAN_POINT('Ctrl Pts',(-19.6780827744426,-7.61336212350879,
0.));
#12357=CARTESIAN_POINT('Ctrl Pts',(-19.7287195480601,-7.60800746969261,
0.));
#12358=CARTESIAN_POINT('Ctrl Pts',(-19.7794022782484,-7.60237814110186,
0.));
#12359=CARTESIAN_POINT('Ctrl Pts',(-19.830129556152,-7.59647587605448,0.));
#12360=CARTESIAN_POINT('Ctrl Pts',(-19.8808999994024,-7.59030238888852,
0.));
#12361=CARTESIAN_POINT('Ctrl Pts',(-19.931712276832,-7.58385933533351,0.));
#12362=CARTESIAN_POINT('Ctrl Pts',(-19.9825651387294,-7.57714827622806,
0.));
#12363=CARTESIAN_POINT('Ctrl Pts',(-20.0334574248557,-7.57017066105972,
0.));
#12364=CARTESIAN_POINT('Ctrl Pts',(-20.0843880130978,-7.5629278654946,0.));
#12365=CARTESIAN_POINT('Ctrl Pts',(-20.1353557774357,-7.55542122125494,
0.));
#12366=CARTESIAN_POINT('Ctrl Pts',(-20.1863595454674,-7.54765204869254,
0.));
#12367=CARTESIAN_POINT('Ctrl Pts',(-20.2373980474879,-7.53962169534166,
0.));
#12368=CARTESIAN_POINT('Ctrl Pts',(-20.2884698940944,-7.53133155804007,
0.));
#12369=CARTESIAN_POINT('Ctrl Pts',(-20.3395736743243,-7.52278303006887,
0.));
#12370=CARTESIAN_POINT('Ctrl Pts',(-20.3907080367098,-7.51397746081993,
0.));
#12371=CARTESIAN_POINT('Ctrl Pts',(-20.4418717748497,-7.50491611266253,
0.));
#12372=CARTESIAN_POINT('Ctrl Pts',(-20.4930639156161,-7.49560012018405,
0.));
#12373=CARTESIAN_POINT('Ctrl Pts',(-20.5545277683621,-7.48411651832412,
0.));
#12374=CARTESIAN_POINT('Ctrl Pts',(-20.6057817877246,-7.47423073598681,
0.));
#12375=CARTESIAN_POINT('Ctrl Pts',(-20.6468066077586,-7.46612041736313,
0.));
#12376=CARTESIAN_POINT('Ctrl Pts',(-20.6775873630604,-7.45992433946823,
0.));
#12377=CARTESIAN_POINT('Ctrl Pts',(-20.698113262342,-7.455743247944,0.));
#12378=CARTESIAN_POINT('',(-20.698113262342,-7.45574324794406,13.));
#12379=CARTESIAN_POINT('Ctrl Pts',(-20.698113262342,-7.455743247944,13.));
#12380=CARTESIAN_POINT('Ctrl Pts',(-20.5970733933809,-7.47632490106067,
13.));
#12381=CARTESIAN_POINT('Ctrl Pts',(-20.496187784905,-7.49544541955086,13.));
#12382=CARTESIAN_POINT('Ctrl Pts',(-20.3954689842507,-7.51308219823823,
13.));
#12383=CARTESIAN_POINT('Ctrl Pts',(-20.2285735577406,-7.54230710641993,
13.));
#12384=CARTESIAN_POINT('Ctrl Pts',(-20.0621477325708,-7.5674509566436,13.));
#12385=CARTESIAN_POINT('Ctrl Pts',(-19.8963869140364,-7.58830059883611,
13.));
#12386=CARTESIAN_POINT('Ctrl Pts',(-19.7689734275332,-7.60432685659461,
13.));
#12387=CARTESIAN_POINT('Ctrl Pts',(-19.6419503956054,-7.61781485408936,
13.));
#12388=CARTESIAN_POINT('Ctrl Pts',(-19.5154161657059,-7.6286436791923,13.));
#12389=CARTESIAN_POINT('Ctrl Pts',(-19.3792051127088,-7.64030064878198,
13.));
#12390=CARTESIAN_POINT('Ctrl Pts',(-19.2435576448926,-7.64888186434619,
13.));
#12391=CARTESIAN_POINT('Ctrl Pts',(-19.1086228836126,-7.65417053742023,
13.));
#12392=CARTESIAN_POINT('Ctrl Pts',(-19.0339193365638,-7.65709849041074,
13.));
#12393=CARTESIAN_POINT('Ctrl Pts',(-18.9594327323946,-7.65902218171137,
13.));
#12394=CARTESIAN_POINT('Ctrl Pts',(-18.8851905417994,-7.65990167998082,
13.));
#12395=CARTESIAN_POINT('Ctrl Pts',(-18.813647852512,-7.6607491990386,13.));
#12396=CARTESIAN_POINT('Ctrl Pts',(-18.7423342827731,-7.66062065572261,
13.));
#12397=CARTESIAN_POINT('Ctrl Pts',(-18.6712863088345,-7.65944821269773,
13.));
#12398=CARTESIAN_POINT('Ctrl Pts',(-18.6098790720615,-7.65843486238751,
13.));
#12399=CARTESIAN_POINT('Ctrl Pts',(-18.5486691990401,-7.65664478981881,
13.));
#12400=CARTESIAN_POINT('Ctrl Pts',(-18.487665984844,-7.65407864069299,13.));
#12401=CARTESIAN_POINT('Ctrl Pts',(-18.4438867380777,-7.65223703156962,
13.));
#12402=CARTESIAN_POINT('Ctrl Pts',(-18.4002130326034,-7.64999840196622,
13.));
#12403=CARTESIAN_POINT('Ctrl Pts',(-18.3566609382467,-7.64732656561704,
13.));
#12404=CARTESIAN_POINT('Ctrl Pts',(-18.3138180356583,-7.6446982368046,13.));
#12405=CARTESIAN_POINT('Ctrl Pts',(-18.2710948572002,-7.64164464439117,
13.));
#12406=CARTESIAN_POINT('Ctrl Pts',(-18.2285117407113,-7.63811742043515,
13.));
#12407=CARTESIAN_POINT('Ctrl Pts',(-18.1915896769364,-7.63505911003915,
13.));
#12408=CARTESIAN_POINT('Ctrl Pts',(-18.1547737063835,-7.63164238135661,
13.));
#12409=CARTESIAN_POINT('Ctrl Pts',(-18.1180614603993,-7.62788266165657,
13.));
#12410=CARTESIAN_POINT('Ctrl Pts',(-18.0848085885333,-7.62447721821159,
13.));
#12411=CARTESIAN_POINT('Ctrl Pts',(-18.0516390295742,-7.62079564899676,
13.));
#12412=CARTESIAN_POINT('Ctrl Pts',(-18.0185473583857,-7.61686093606607,
13.));
#12413=CARTESIAN_POINT('Ctrl Pts',(-17.9906726825976,-7.61354654173896,
13.));
#12414=CARTESIAN_POINT('Ctrl Pts',(-17.9628527173259,-7.61005417561197,
13.));
#12415=CARTESIAN_POINT('Ctrl Pts',(-17.935095231232,-7.60636550499839,13.));
#12416=CARTESIAN_POINT('Ctrl Pts',(-17.8949271288068,-7.60102759728881,
13.));
#12417=CARTESIAN_POINT('Ctrl Pts',(-17.8548900767542,-7.5952778259702,13.));
#12418=CARTESIAN_POINT('Ctrl Pts',(-17.8150590780368,-7.58891067826985,
13.));
#12419=CARTESIAN_POINT('Ctrl Pts',(-17.7909916433023,-7.58506340060529,
13.));
#12420=CARTESIAN_POINT('Ctrl Pts',(-17.7670005718664,-7.58098742040678,
13.));
#12421=CARTESIAN_POINT('Ctrl Pts',(-17.743095591428,-7.57665817622453,13.));
#12422=CARTESIAN_POINT('Ctrl Pts',(-17.7210484745798,-7.57266539519733,
13.));
#12423=CARTESIAN_POINT('Ctrl Pts',(-17.6990750119521,-7.5684559326956,13.));
#12424=CARTESIAN_POINT('Ctrl Pts',(-17.6771683095201,-7.56405390355785,
13.));
#12425=CARTESIAN_POINT('Ctrl Pts',(-17.6470334201915,-7.55799846635553,
13.));
#12426=CARTESIAN_POINT('Ctrl Pts',(-17.6170224066021,-7.55158552707305,
13.));
#12427=CARTESIAN_POINT('Ctrl Pts',(-17.5870909089238,-7.54495919885366,
13.));
#12428=CARTESIAN_POINT('Ctrl Pts',(-17.5681018329048,-7.54075533803665,
13.));
#12429=CARTESIAN_POINT('Ctrl Pts',(-17.5491442490796,-7.53646718585433,
13.));
#12430=CARTESIAN_POINT('Ctrl Pts',(-17.5302169633081,-7.53210330802969,
13.));
#12431=CARTESIAN_POINT('Ctrl Pts',(-17.5132306053115,-7.52818693080173,
13.));
#12432=CARTESIAN_POINT('Ctrl Pts',(-17.4962684160869,-7.52421025221118,
13.));
#12433=CARTESIAN_POINT('Ctrl Pts',(-17.4793429835075,-7.52014106530203,
13.));
#12434=CARTESIAN_POINT('Ctrl Pts',(-17.4615509829577,-7.51586353943172,
13.));
#12435=CARTESIAN_POINT('Ctrl Pts',(-17.4437995539221,-7.51148394209351,
13.));
#12436=CARTESIAN_POINT('Ctrl Pts',(-17.4261238143002,-7.50690601560406,
13.));
#12437=CARTESIAN_POINT('Ctrl Pts',(-17.3967644499127,-7.49930208983814,
13.));
#12438=CARTESIAN_POINT('Ctrl Pts',(-17.367616818873,-7.49114308213498,13.));
#12439=CARTESIAN_POINT('Ctrl Pts',(-17.3388922514848,-7.48183975621699,
13.));
#12440=CARTESIAN_POINT('Ctrl Pts',(-17.3230525027431,-7.47670957120807,
13.));
#12441=CARTESIAN_POINT('Ctrl Pts',(-17.3073418194459,-7.47123011544593,
13.));
#12442=CARTESIAN_POINT('Ctrl Pts',(-17.2917860605524,-7.46532888197223,
13.));
#12443=CARTESIAN_POINT('Ctrl Pts',(-17.2791322530001,-7.46052853290484,
13.));
#12444=CARTESIAN_POINT('Ctrl Pts',(-17.2665809316714,-7.45544915948875,
13.));
#12445=CARTESIAN_POINT('Ctrl Pts',(-17.2541372868972,-7.45007618140238,
13.));
#12446=CARTESIAN_POINT('',(-20.698113262342,-7.45574324794406,0.));
#12447=CARTESIAN_POINT('Origin',(-5.38923623413286E-12,-1.75106900012182E-12,
0.));
#12448=CARTESIAN_POINT('',(-21.1275013067528,-6.1342227326009,0.));
#12449=CARTESIAN_POINT('Origin',(-5.38923623413286E-12,-1.75106900012182E-12,
0.));
#12450=CARTESIAN_POINT('',(-21.1275013067528,-6.1342227326009,13.));
#12451=CARTESIAN_POINT('Origin',(-5.38923623413286E-12,-1.75106900012182E-12,
13.));
#12452=CARTESIAN_POINT('',(-21.1275013067528,-6.1342227326009,0.));
#12453=CARTESIAN_POINT('Ctrl Pts',(-18.337935196262,-4.1144891981253,0.));
#12454=CARTESIAN_POINT('Ctrl Pts',(-18.337935196262,-4.1144891981253,21.));
#12455=CARTESIAN_POINT('Ctrl Pts',(-18.3471320125699,-4.11655269114951,
0.));
#12456=CARTESIAN_POINT('Ctrl Pts',(-18.3471320125699,-4.11655269114951,
21.));
#12457=CARTESIAN_POINT('Ctrl Pts',(-18.3654573320481,-4.12092019868859,
0.));
#12458=CARTESIAN_POINT('Ctrl Pts',(-18.3654573320481,-4.12092019868859,
21.));
#12459=CARTESIAN_POINT('Ctrl Pts',(-18.3927403741815,-4.12819301671078,
0.));
#12460=CARTESIAN_POINT('Ctrl Pts',(-18.3927403741815,-4.12819301671078,
21.));
#12461=CARTESIAN_POINT('Ctrl Pts',(-18.4287286547442,-4.13926275457062,
0.));
#12462=CARTESIAN_POINT('Ctrl Pts',(-18.4287286547442,-4.13926275457062,
21.));
#12463=CARTESIAN_POINT('Ctrl Pts',(-18.4731856794913,-4.15497867673974,
0.));
#12464=CARTESIAN_POINT('Ctrl Pts',(-18.4731856794913,-4.15497867673974,
21.));
#12465=CARTESIAN_POINT('Ctrl Pts',(-18.5172668097744,-4.17205262766561,
0.));
#12466=CARTESIAN_POINT('Ctrl Pts',(-18.5172668097744,-4.17205262766561,
21.));
#12467=CARTESIAN_POINT('Ctrl Pts',(-18.5611217636409,-4.1899696727862,0.));
#12468=CARTESIAN_POINT('Ctrl Pts',(-18.5611217636409,-4.1899696727862,21.));
#12469=CARTESIAN_POINT('Ctrl Pts',(-18.6048602364653,-4.20834600700664,
0.));
#12470=CARTESIAN_POINT('Ctrl Pts',(-18.6048602364653,-4.20834600700664,
21.));
#12471=CARTESIAN_POINT('Ctrl Pts',(-18.6485210883348,-4.22703266508918,
0.));
#12472=CARTESIAN_POINT('Ctrl Pts',(-18.6485210883348,-4.22703266508918,
21.));
#12473=CARTESIAN_POINT('Ctrl Pts',(-18.6920958920047,-4.24603817988452,
0.));
#12474=CARTESIAN_POINT('Ctrl Pts',(-18.6920958920047,-4.24603817988452,
21.));
#12475=CARTESIAN_POINT('Ctrl Pts',(-18.735547949685,-4.26546636161932,0.));
#12476=CARTESIAN_POINT('Ctrl Pts',(-18.735547949685,-4.26546636161932,21.));
#12477=CARTESIAN_POINT('Ctrl Pts',(-18.778832216358,-4.28545098663153,0.));
#12478=CARTESIAN_POINT('Ctrl Pts',(-18.778832216358,-4.28545098663153,21.));
#12479=CARTESIAN_POINT('Ctrl Pts',(-18.8219166495975,-4.30608591031525,
0.));
#12480=CARTESIAN_POINT('Ctrl Pts',(-18.8219166495975,-4.30608591031525,
21.));
#12481=CARTESIAN_POINT('Ctrl Pts',(-18.8647973781745,-4.32737526247704,
0.));
#12482=CARTESIAN_POINT('Ctrl Pts',(-18.8647973781745,-4.32737526247704,
21.));
#12483=CARTESIAN_POINT('Ctrl Pts',(-18.9074876952706,-4.34926881342021,
0.));
#12484=CARTESIAN_POINT('Ctrl Pts',(-18.9074876952706,-4.34926881342021,
21.));
#12485=CARTESIAN_POINT('Ctrl Pts',(-18.9500107909187,-4.37168516143122,
0.));
#12486=CARTESIAN_POINT('Ctrl Pts',(-18.9500107909187,-4.37168516143122,
21.));
#12487=CARTESIAN_POINT('Ctrl Pts',(-18.9923914823906,-4.39453820875554,
0.));
#12488=CARTESIAN_POINT('Ctrl Pts',(-18.9923914823906,-4.39453820875554,
21.));
#12489=CARTESIAN_POINT('Ctrl Pts',(-19.034647328575,-4.41776558033331,0.));
#12490=CARTESIAN_POINT('Ctrl Pts',(-19.034647328575,-4.41776558033331,21.));
#12491=CARTESIAN_POINT('Ctrl Pts',(-19.0767833717249,-4.44134542994081,
0.));
#12492=CARTESIAN_POINT('Ctrl Pts',(-19.0767833717249,-4.44134542994081,
21.));
#12493=CARTESIAN_POINT('Ctrl Pts',(-19.1187970904933,-4.46528051067021,
0.));
#12494=CARTESIAN_POINT('Ctrl Pts',(-19.1187970904933,-4.46528051067021,
21.));
#12495=CARTESIAN_POINT('Ctrl Pts',(-19.1606814968494,-4.48958819710576,
0.));
#12496=CARTESIAN_POINT('Ctrl Pts',(-19.1606814968494,-4.48958819710576,
21.));
#12497=CARTESIAN_POINT('Ctrl Pts',(-19.2024287376926,-4.51428889122954,
0.));
#12498=CARTESIAN_POINT('Ctrl Pts',(-19.2024287376926,-4.51428889122954,
21.));
#12499=CARTESIAN_POINT('Ctrl Pts',(-19.2440340196551,-4.53939338835151,
0.));
#12500=CARTESIAN_POINT('Ctrl Pts',(-19.2440340196551,-4.53939338835151,
21.));
#12501=CARTESIAN_POINT('Ctrl Pts',(-19.2854975819105,-4.5648965160674,0.));
#12502=CARTESIAN_POINT('Ctrl Pts',(-19.2854975819105,-4.5648965160674,21.));
#12503=CARTESIAN_POINT('Ctrl Pts',(-19.3268225655679,-4.59078395765677,
0.));
#12504=CARTESIAN_POINT('Ctrl Pts',(-19.3268225655679,-4.59078395765677,
21.));
#12505=CARTESIAN_POINT('Ctrl Pts',(-19.3680137353983,-4.61703633725711,
0.));
#12506=CARTESIAN_POINT('Ctrl Pts',(-19.3680137353983,-4.61703633725711,
21.));
#12507=CARTESIAN_POINT('Ctrl Pts',(-19.4090759683639,-4.64363405547472,
0.));
#12508=CARTESIAN_POINT('Ctrl Pts',(-19.4090759683639,-4.64363405547472,
21.));
#12509=CARTESIAN_POINT('Ctrl Pts',(-19.4500125912299,-4.67056260851453,
0.));
#12510=CARTESIAN_POINT('Ctrl Pts',(-19.4500125912299,-4.67056260851453,
21.));
#12511=CARTESIAN_POINT('Ctrl Pts',(-19.4908246636763,-4.69781487613784,
0.));
#12512=CARTESIAN_POINT('Ctrl Pts',(-19.4908246636763,-4.69781487613784,
21.));
#12513=CARTESIAN_POINT('Ctrl Pts',(-19.531511899192,-4.72538815796615,0.));
#12514=CARTESIAN_POINT('Ctrl Pts',(-19.531511899192,-4.72538815796615,21.));
#12515=CARTESIAN_POINT('Ctrl Pts',(-19.5720732205813,-4.7532823819461,0.));
#12516=CARTESIAN_POINT('Ctrl Pts',(-19.5720732205813,-4.7532823819461,21.));
#12517=CARTESIAN_POINT('Ctrl Pts',(-19.6125074152527,-4.7814979936173,0.));
#12518=CARTESIAN_POINT('Ctrl Pts',(-19.6125074152527,-4.7814979936173,21.));
#12519=CARTESIAN_POINT('Ctrl Pts',(-19.6528138625329,-4.8100336141806,0.));
#12520=CARTESIAN_POINT('Ctrl Pts',(-19.6528138625329,-4.8100336141806,21.));
#12521=CARTESIAN_POINT('Ctrl Pts',(-19.6929928227072,-4.83888510708974,
0.));
#12522=CARTESIAN_POINT('Ctrl Pts',(-19.6929928227072,-4.83888510708974,
21.));
#12523=CARTESIAN_POINT('Ctrl Pts',(-19.7330450480715,-4.86804682289086,
0.));
#12524=CARTESIAN_POINT('Ctrl Pts',(-19.7330450480715,-4.86804682289086,
21.));
#12525=CARTESIAN_POINT('Ctrl Pts',(-19.772971552601,-4.89751233527804,0.));
#12526=CARTESIAN_POINT('Ctrl Pts',(-19.772971552601,-4.89751233527804,21.));
#12527=CARTESIAN_POINT('Ctrl Pts',(-19.8127733387903,-4.92727531494346,
0.));
#12528=CARTESIAN_POINT('Ctrl Pts',(-19.8127733387903,-4.92727531494346,
21.));
#12529=CARTESIAN_POINT('Ctrl Pts',(-19.8524510953961,-4.95733049830095,
0.));
#12530=CARTESIAN_POINT('Ctrl Pts',(-19.8524510953961,-4.95733049830095,
21.));
#12531=CARTESIAN_POINT('Ctrl Pts',(-19.8920050831202,-4.98767405031333,
0.));
#12532=CARTESIAN_POINT('Ctrl Pts',(-19.8920050831202,-4.98767405031333,
21.));
#12533=CARTESIAN_POINT('Ctrl Pts',(-19.931435301086,-5.01830302225557,0.));
#12534=CARTESIAN_POINT('Ctrl Pts',(-19.931435301086,-5.01830302225557,21.));
#12535=CARTESIAN_POINT('Ctrl Pts',(-19.9707415879783,-5.04921502064063,
0.));
#12536=CARTESIAN_POINT('Ctrl Pts',(-19.9707415879783,-5.04921502064063,
21.));
#12537=CARTESIAN_POINT('Ctrl Pts',(-20.0099237417205,-5.08040781745336,
0.));
#12538=CARTESIAN_POINT('Ctrl Pts',(-20.0099237417205,-5.08040781745336,
21.));
#12539=CARTESIAN_POINT('Ctrl Pts',(-20.0489816528155,-5.11187891582334,
0.));
#12540=CARTESIAN_POINT('Ctrl Pts',(-20.0489816528155,-5.11187891582334,
21.));
#12541=CARTESIAN_POINT('Ctrl Pts',(-20.087915358486,-5.14362537555397,0.));
#12542=CARTESIAN_POINT('Ctrl Pts',(-20.087915358486,-5.14362537555397,21.));
#12543=CARTESIAN_POINT('Ctrl Pts',(-20.1267249732337,-5.17564404279921,
0.));
#12544=CARTESIAN_POINT('Ctrl Pts',(-20.1267249732337,-5.17564404279921,
21.));
#12545=CARTESIAN_POINT('Ctrl Pts',(-20.1654106491899,-5.20793168386163,
0.));
#12546=CARTESIAN_POINT('Ctrl Pts',(-20.1654106491899,-5.20793168386163,
21.));
#12547=CARTESIAN_POINT('Ctrl Pts',(-20.2039725283917,-5.2404851444189,0.));
#12548=CARTESIAN_POINT('Ctrl Pts',(-20.2039725283917,-5.2404851444189,21.));
#12549=CARTESIAN_POINT('Ctrl Pts',(-20.2424106921768,-5.2733015229815,0.));
#12550=CARTESIAN_POINT('Ctrl Pts',(-20.2424106921768,-5.2733015229815,21.));
#12551=CARTESIAN_POINT('Ctrl Pts',(-20.2807251380077,-5.30637824220997,
0.));
#12552=CARTESIAN_POINT('Ctrl Pts',(-20.2807251380077,-5.30637824220997,
21.));
#12553=CARTESIAN_POINT('Ctrl Pts',(-20.3189158047642,-5.33971294212213,
0.));
#12554=CARTESIAN_POINT('Ctrl Pts',(-20.3189158047642,-5.33971294212213,
21.));
#12555=CARTESIAN_POINT('Ctrl Pts',(-20.3569825877537,-5.37330341114649,
0.));
#12556=CARTESIAN_POINT('Ctrl Pts',(-20.3569825877537,-5.37330341114649,
21.));
#12557=CARTESIAN_POINT('Ctrl Pts',(-20.3949253578015,-5.40714750595874,
0.));
#12558=CARTESIAN_POINT('Ctrl Pts',(-20.3949253578015,-5.40714750595874,
21.));
#12559=CARTESIAN_POINT('Ctrl Pts',(-20.4327439816542,-5.44124306065111,
0.));
#12560=CARTESIAN_POINT('Ctrl Pts',(-20.4327439816542,-5.44124306065111,
21.));
#12561=CARTESIAN_POINT('Ctrl Pts',(-20.4704383353718,-5.4755878444985,0.));
#12562=CARTESIAN_POINT('Ctrl Pts',(-20.4704383353718,-5.4755878444985,21.));
#12563=CARTESIAN_POINT('Ctrl Pts',(-20.5080083009242,-5.51017962306782,
0.));
#12564=CARTESIAN_POINT('Ctrl Pts',(-20.5080083009242,-5.51017962306782,
21.));
#12565=CARTESIAN_POINT('Ctrl Pts',(-20.5454537676144,-5.5450161968946,0.));
#12566=CARTESIAN_POINT('Ctrl Pts',(-20.5454537676144,-5.5450161968946,21.));
#12567=CARTESIAN_POINT('Ctrl Pts',(-20.5827746317185,-5.58009544402474,
0.));
#12568=CARTESIAN_POINT('Ctrl Pts',(-20.5827746317185,-5.58009544402474,
21.));
#12569=CARTESIAN_POINT('Ctrl Pts',(-20.6199707996366,-5.61541536715149,
0.));
#12570=CARTESIAN_POINT('Ctrl Pts',(-20.6199707996366,-5.61541536715149,
21.));
#12571=CARTESIAN_POINT('Ctrl Pts',(-20.6570421847033,-5.65097411164334,
0.));
#12572=CARTESIAN_POINT('Ctrl Pts',(-20.6570421847033,-5.65097411164334,
21.));
#12573=CARTESIAN_POINT('Ctrl Pts',(-20.6939886877061,-5.68676990500163,
0.));
#12574=CARTESIAN_POINT('Ctrl Pts',(-20.6939886877061,-5.68676990500163,
21.));
#12575=CARTESIAN_POINT('Ctrl Pts',(-20.7308101804425,-5.72280100798241,
0.));
#12576=CARTESIAN_POINT('Ctrl Pts',(-20.7308101804425,-5.72280100798241,
21.));
#12577=CARTESIAN_POINT('Ctrl Pts',(-20.7675064905026,-5.75906566327795,
0.));
#12578=CARTESIAN_POINT('Ctrl Pts',(-20.7675064905026,-5.75906566327795,
21.));
#12579=CARTESIAN_POINT('Ctrl Pts',(-20.8040773827343,-5.79556203439644,
0.));
#12580=CARTESIAN_POINT('Ctrl Pts',(-20.8040773827343,-5.79556203439644,
21.));
#12581=CARTESIAN_POINT('Ctrl Pts',(-20.8405225541277,-5.83228817460177,
0.));
#12582=CARTESIAN_POINT('Ctrl Pts',(-20.8405225541277,-5.83228817460177,
21.));
#12583=CARTESIAN_POINT('Ctrl Pts',(-20.8768416821402,-5.86924212736287,
0.));
#12584=CARTESIAN_POINT('Ctrl Pts',(-20.8768416821402,-5.86924212736287,
21.));
#12585=CARTESIAN_POINT('Ctrl Pts',(-20.9130344665641,-5.90642200662599,
0.));
#12586=CARTESIAN_POINT('Ctrl Pts',(-20.9130344665641,-5.90642200662599,
21.));
#12587=CARTESIAN_POINT('Ctrl Pts',(-20.9491006734021,-5.94382608200804,
0.));
#12588=CARTESIAN_POINT('Ctrl Pts',(-20.9491006734021,-5.94382608200804,
21.));
#12589=CARTESIAN_POINT('Ctrl Pts',(-20.9850401822713,-5.98145286361836,
0.));
#12590=CARTESIAN_POINT('Ctrl Pts',(-20.9850401822713,-5.98145286361836,
21.));
#12591=CARTESIAN_POINT('Ctrl Pts',(-21.0208530236003,-6.01930117633044,
0.));
#12592=CARTESIAN_POINT('Ctrl Pts',(-21.0208530236003,-6.01930117633044,
21.));
#12593=CARTESIAN_POINT('Ctrl Pts',(-21.0565393163693,-6.05737013696532,
0.));
#12594=CARTESIAN_POINT('Ctrl Pts',(-21.0565393163693,-6.05737013696532,
21.));
#12595=CARTESIAN_POINT('Ctrl Pts',(-21.0849872356853,-6.08800133883114,
0.));
#12596=CARTESIAN_POINT('Ctrl Pts',(-21.0849872356853,-6.08800133883114,
21.));
#12597=CARTESIAN_POINT('Ctrl Pts',(-21.1062663590356,-6.11107360216957,
0.));
#12598=CARTESIAN_POINT('Ctrl Pts',(-21.1062663590356,-6.11107360216957,
21.));
#12599=CARTESIAN_POINT('Ctrl Pts',(-21.1204271980506,-6.12649903511517,
0.));
#12600=CARTESIAN_POINT('Ctrl Pts',(-21.1204271980506,-6.12649903511517,
21.));
#12601=CARTESIAN_POINT('Ctrl Pts',(-21.1275013067528,-6.1342227326009,0.));
#12602=CARTESIAN_POINT('Ctrl Pts',(-21.1275013067528,-6.1342227326009,21.));
#12603=CARTESIAN_POINT('Ctrl Pts',(-18.337935196262,-4.1144891981253,0.));
#12604=CARTESIAN_POINT('Ctrl Pts',(-18.3471320125699,-4.11655269114951,
0.));
#12605=CARTESIAN_POINT('Ctrl Pts',(-18.3654573320481,-4.12092019868859,
0.));
#12606=CARTESIAN_POINT('Ctrl Pts',(-18.3927403741815,-4.12819301671078,
0.));
#12607=CARTESIAN_POINT('Ctrl Pts',(-18.4287286547442,-4.13926275457062,
0.));
#12608=CARTESIAN_POINT('Ctrl Pts',(-18.4731856794913,-4.15497867673974,
0.));
#12609=CARTESIAN_POINT('Ctrl Pts',(-18.5172668097744,-4.17205262766561,
0.));
#12610=CARTESIAN_POINT('Ctrl Pts',(-18.5611217636409,-4.1899696727862,0.));
#12611=CARTESIAN_POINT('Ctrl Pts',(-18.6048602364653,-4.20834600700664,
0.));
#12612=CARTESIAN_POINT('Ctrl Pts',(-18.6485210883348,-4.22703266508918,
0.));
#12613=CARTESIAN_POINT('Ctrl Pts',(-18.6920958920047,-4.24603817988452,
0.));
#12614=CARTESIAN_POINT('Ctrl Pts',(-18.735547949685,-4.26546636161932,0.));
#12615=CARTESIAN_POINT('Ctrl Pts',(-18.778832216358,-4.28545098663153,0.));
#12616=CARTESIAN_POINT('Ctrl Pts',(-18.8219166495975,-4.30608591031525,
0.));
#12617=CARTESIAN_POINT('Ctrl Pts',(-18.8647973781745,-4.32737526247704,
0.));
#12618=CARTESIAN_POINT('Ctrl Pts',(-18.9074876952706,-4.34926881342021,
0.));
#12619=CARTESIAN_POINT('Ctrl Pts',(-18.9500107909187,-4.37168516143122,
0.));
#12620=CARTESIAN_POINT('Ctrl Pts',(-18.9923914823906,-4.39453820875554,
0.));
#12621=CARTESIAN_POINT('Ctrl Pts',(-19.034647328575,-4.41776558033331,0.));
#12622=CARTESIAN_POINT('Ctrl Pts',(-19.0767833717249,-4.44134542994081,
0.));
#12623=CARTESIAN_POINT('Ctrl Pts',(-19.1187970904933,-4.46528051067021,
0.));
#12624=CARTESIAN_POINT('Ctrl Pts',(-19.1606814968494,-4.48958819710576,
0.));
#12625=CARTESIAN_POINT('Ctrl Pts',(-19.2024287376926,-4.51428889122954,
0.));
#12626=CARTESIAN_POINT('Ctrl Pts',(-19.2440340196551,-4.53939338835151,
0.));
#12627=CARTESIAN_POINT('Ctrl Pts',(-19.2854975819105,-4.5648965160674,0.));
#12628=CARTESIAN_POINT('Ctrl Pts',(-19.3268225655679,-4.59078395765677,
0.));
#12629=CARTESIAN_POINT('Ctrl Pts',(-19.3680137353983,-4.61703633725711,
0.));
#12630=CARTESIAN_POINT('Ctrl Pts',(-19.4090759683639,-4.64363405547472,
0.));
#12631=CARTESIAN_POINT('Ctrl Pts',(-19.4500125912299,-4.67056260851453,
0.));
#12632=CARTESIAN_POINT('Ctrl Pts',(-19.4908246636763,-4.69781487613784,
0.));
#12633=CARTESIAN_POINT('Ctrl Pts',(-19.531511899192,-4.72538815796615,0.));
#12634=CARTESIAN_POINT('Ctrl Pts',(-19.5720732205813,-4.7532823819461,0.));
#12635=CARTESIAN_POINT('Ctrl Pts',(-19.6125074152527,-4.7814979936173,0.));
#12636=CARTESIAN_POINT('Ctrl Pts',(-19.6528138625329,-4.8100336141806,0.));
#12637=CARTESIAN_POINT('Ctrl Pts',(-19.6929928227072,-4.83888510708974,
0.));
#12638=CARTESIAN_POINT('Ctrl Pts',(-19.7330450480715,-4.86804682289086,
0.));
#12639=CARTESIAN_POINT('Ctrl Pts',(-19.772971552601,-4.89751233527804,0.));
#12640=CARTESIAN_POINT('Ctrl Pts',(-19.8127733387903,-4.92727531494346,
0.));
#12641=CARTESIAN_POINT('Ctrl Pts',(-19.8524510953961,-4.95733049830095,
0.));
#12642=CARTESIAN_POINT('Ctrl Pts',(-19.8920050831202,-4.98767405031333,
0.));
#12643=CARTESIAN_POINT('Ctrl Pts',(-19.931435301086,-5.01830302225557,0.));
#12644=CARTESIAN_POINT('Ctrl Pts',(-19.9707415879783,-5.04921502064063,
0.));
#12645=CARTESIAN_POINT('Ctrl Pts',(-20.0099237417205,-5.08040781745336,
0.));
#12646=CARTESIAN_POINT('Ctrl Pts',(-20.0489816528155,-5.11187891582334,
0.));
#12647=CARTESIAN_POINT('Ctrl Pts',(-20.087915358486,-5.14362537555397,0.));
#12648=CARTESIAN_POINT('Ctrl Pts',(-20.1267249732337,-5.17564404279921,
0.));
#12649=CARTESIAN_POINT('Ctrl Pts',(-20.1654106491899,-5.20793168386163,
0.));
#12650=CARTESIAN_POINT('Ctrl Pts',(-20.2039725283917,-5.2404851444189,0.));
#12651=CARTESIAN_POINT('Ctrl Pts',(-20.2424106921768,-5.2733015229815,0.));
#12652=CARTESIAN_POINT('Ctrl Pts',(-20.2807251380077,-5.30637824220997,
0.));
#12653=CARTESIAN_POINT('Ctrl Pts',(-20.3189158047642,-5.33971294212213,
0.));
#12654=CARTESIAN_POINT('Ctrl Pts',(-20.3569825877537,-5.37330341114649,
0.));
#12655=CARTESIAN_POINT('Ctrl Pts',(-20.3949253578015,-5.40714750595874,
0.));
#12656=CARTESIAN_POINT('Ctrl Pts',(-20.4327439816542,-5.44124306065111,
0.));
#12657=CARTESIAN_POINT('Ctrl Pts',(-20.4704383353718,-5.4755878444985,0.));
#12658=CARTESIAN_POINT('Ctrl Pts',(-20.5080083009242,-5.51017962306782,
0.));
#12659=CARTESIAN_POINT('Ctrl Pts',(-20.5454537676144,-5.5450161968946,0.));
#12660=CARTESIAN_POINT('Ctrl Pts',(-20.5827746317185,-5.58009544402474,
0.));
#12661=CARTESIAN_POINT('Ctrl Pts',(-20.6199707996366,-5.61541536715149,
0.));
#12662=CARTESIAN_POINT('Ctrl Pts',(-20.6570421847033,-5.65097411164334,
0.));
#12663=CARTESIAN_POINT('Ctrl Pts',(-20.6939886877061,-5.68676990500163,
0.));
#12664=CARTESIAN_POINT('Ctrl Pts',(-20.7308101804425,-5.72280100798241,
0.));
#12665=CARTESIAN_POINT('Ctrl Pts',(-20.7675064905026,-5.75906566327795,
0.));
#12666=CARTESIAN_POINT('Ctrl Pts',(-20.8040773827343,-5.79556203439644,
0.));
#12667=CARTESIAN_POINT('Ctrl Pts',(-20.8405225541277,-5.83228817460177,
0.));
#12668=CARTESIAN_POINT('Ctrl Pts',(-20.8768416821402,-5.86924212736287,
0.));
#12669=CARTESIAN_POINT('Ctrl Pts',(-20.9130344665641,-5.90642200662599,
0.));
#12670=CARTESIAN_POINT('Ctrl Pts',(-20.9491006734021,-5.94382608200804,
0.));
#12671=CARTESIAN_POINT('Ctrl Pts',(-20.9850401822713,-5.98145286361836,
0.));
#12672=CARTESIAN_POINT('Ctrl Pts',(-21.0280155918661,-6.02687083887286,
0.));
#12673=CARTESIAN_POINT('Ctrl Pts',(-21.0636702474951,-6.06499496148844,
0.));
#12674=CARTESIAN_POINT('Ctrl Pts',(-21.0920928984154,-6.09567013127871,
0.));
#12675=CARTESIAN_POINT('Ctrl Pts',(-21.1133530893457,-6.118775337615,0.));
#12676=CARTESIAN_POINT('Ctrl Pts',(-21.1275013067528,-6.1342227326009,0.));
#12677=CARTESIAN_POINT('Ctrl Pts',(-18.337935196262,-4.1144891981253,13.));
#12678=CARTESIAN_POINT('Ctrl Pts',(-18.3534360435645,-4.11796712887951,
13.));
#12679=CARTESIAN_POINT('Ctrl Pts',(-18.3688191548995,-4.12185943358937,
13.));
#12680=CARTESIAN_POINT('Ctrl Pts',(-18.3840926404824,-4.12613856044267,
13.));
#12681=CARTESIAN_POINT('Ctrl Pts',(-18.4019943079477,-4.13115401716693,
13.));
#12682=CARTESIAN_POINT('Ctrl Pts',(-18.4197456248295,-4.13670006307401,
13.));
#12683=CARTESIAN_POINT('Ctrl Pts',(-18.4373797424196,-4.1426637807957,13.));
#12684=CARTESIAN_POINT('Ctrl Pts',(-18.4621917897769,-4.15105501703309,
13.));
#12685=CARTESIAN_POINT('Ctrl Pts',(-18.4867739015683,-4.16026629328987,
13.));
#12686=CARTESIAN_POINT('Ctrl Pts',(-18.5112408492934,-4.16990400115282,
13.));
#12687=CARTESIAN_POINT('Ctrl Pts',(-18.5275152282609,-4.17631459686346,
13.));
#12688=CARTESIAN_POINT('Ctrl Pts',(-18.5437392096496,-4.18291190640786,
13.));
#12689=CARTESIAN_POINT('Ctrl Pts',(-18.5599376581358,-4.18960898617043,
13.));
#12690=CARTESIAN_POINT('Ctrl Pts',(-18.5769891804703,-4.19665876042785,
13.));
#12691=CARTESIAN_POINT('Ctrl Pts',(-18.5940126577989,-4.20381824254442,
13.));
#12692=CARTESIAN_POINT('Ctrl Pts',(-18.6110185062838,-4.21104759333806,
13.));
#12693=CARTESIAN_POINT('Ctrl Pts',(-18.6299044319376,-4.21907618313382,
13.));
#12694=CARTESIAN_POINT('Ctrl Pts',(-18.6487682283615,-4.22719219297435,
13.));
#12695=CARTESIAN_POINT('Ctrl Pts',(-18.6676042988365,-4.23540730606872,
13.));
#12696=CARTESIAN_POINT('Ctrl Pts',(-18.6960005893047,-4.24779198778706,
13.));
#12697=CARTESIAN_POINT('Ctrl Pts',(-18.7243319351566,-4.26040793123127,
13.));
#12698=CARTESIAN_POINT('Ctrl Pts',(-18.7525479285623,-4.27340283281641,
13.));
#12699=CARTESIAN_POINT('Ctrl Pts',(-18.7730462309054,-4.28284334471974,
13.));
#12700=CARTESIAN_POINT('Ctrl Pts',(-18.7934827312586,-4.29248702330122,
13.));
#12701=CARTESIAN_POINT('Ctrl Pts',(-18.8138501272238,-4.30235320731447,
13.));
#12702=CARTESIAN_POINT('Ctrl Pts',(-18.8387475247628,-4.31441377244467,
13.));
#12703=CARTESIAN_POINT('Ctrl Pts',(-18.8635420328974,-4.32680560862846,
13.));
#12704=CARTESIAN_POINT('Ctrl Pts',(-18.8882460103721,-4.33948253068856,
13.));
#12705=CARTESIAN_POINT('Ctrl Pts',(-18.9149304060727,-4.35317571045545,
13.));
#12706=CARTESIAN_POINT('Ctrl Pts',(-18.9415109549191,-4.36719580768733,
13.));
#12707=CARTESIAN_POINT('Ctrl Pts',(-18.9680129070824,-4.38145466528704,
13.));
#12708=CARTESIAN_POINT('Ctrl Pts',(-18.9924793848252,-4.39461837564137,
13.));
#12709=CARTESIAN_POINT('Ctrl Pts',(-19.0168796293529,-4.40798318219363,
13.));
#12710=CARTESIAN_POINT('Ctrl Pts',(-19.0412206988293,-4.42152146524019,
13.));
#12711=CARTESIAN_POINT('Ctrl Pts',(-19.0742892915424,-4.43991391790276,
13.));
#12712=CARTESIAN_POINT('Ctrl Pts',(-19.1072480696,-4.45862842583326,13.));
#12713=CARTESIAN_POINT('Ctrl Pts',(-19.1400849917464,-4.47769255669731,
13.));
#12714=CARTESIAN_POINT('Ctrl Pts',(-19.1717719124003,-4.49608903123077,
13.));
#12715=CARTESIAN_POINT('Ctrl Pts',(-19.2033430485145,-4.51481852753576,
13.));
#12716=CARTESIAN_POINT('Ctrl Pts',(-19.234791092488,-4.53389559694226,13.));
#12717=CARTESIAN_POINT('Ctrl Pts',(-19.2775141413934,-4.55981233026633,
13.));
#12718=CARTESIAN_POINT('Ctrl Pts',(-19.3200109594547,-4.58636743991277,
13.));
#12719=CARTESIAN_POINT('Ctrl Pts',(-19.3623013146402,-4.61347737193446,
13.));
#12720=CARTESIAN_POINT('Ctrl Pts',(-19.399473617434,-4.63730641279748,13.));
#12721=CARTESIAN_POINT('Ctrl Pts',(-19.4364884576265,-4.66155758403617,
13.));
#12722=CARTESIAN_POINT('Ctrl Pts',(-19.4733518508893,-4.68619912965976,
13.));
#12723=CARTESIAN_POINT('Ctrl Pts',(-19.5276974421966,-4.72252675034556,
13.));
#12724=CARTESIAN_POINT('Ctrl Pts',(-19.5817111528826,-4.7597114391696,13.));
#12725=CARTESIAN_POINT('Ctrl Pts',(-19.6353839065147,-4.79774570303518,
13.));
#12726=CARTESIAN_POINT('Ctrl Pts',(-19.7031194454445,-4.84574531524799,
13.));
#12727=CARTESIAN_POINT('Ctrl Pts',(-19.7703134647831,-4.8950930427256,13.));
#12728=CARTESIAN_POINT('Ctrl Pts',(-19.8369838018469,-4.94566457621167,
13.));
#12729=CARTESIAN_POINT('Ctrl Pts',(-19.9272939135678,-5.01416761729656,
13.));
#12730=CARTESIAN_POINT('Ctrl Pts',(-20.0166413602828,-5.08492180312729,
13.));
#12731=CARTESIAN_POINT('Ctrl Pts',(-20.1050225704216,-5.15778644838132,
13.));
#12732=CARTESIAN_POINT('Ctrl Pts',(-20.1838167338246,-5.22274718783514,
13.));
#12733=CARTESIAN_POINT('Ctrl Pts',(-20.2618454267474,-5.28937724234836,
13.));
#12734=CARTESIAN_POINT('Ctrl Pts',(-20.3391090332473,-5.35757729646381,
13.));
#12735=CARTESIAN_POINT('Ctrl Pts',(-20.4486128105791,-5.45423552765683,
13.));
#12736=CARTESIAN_POINT('Ctrl Pts',(-20.5565772409505,-5.55405241054101,
13.));
#12737=CARTESIAN_POINT('Ctrl Pts',(-20.6629906947268,-5.65680258421402,
13.));
#12738=CARTESIAN_POINT('Ctrl Pts',(-20.745650141592,-5.73661648198461,13.));
#12739=CARTESIAN_POINT('Ctrl Pts',(-20.8273750331781,-5.81820510936894,
13.));
#12740=CARTESIAN_POINT('Ctrl Pts',(-20.9081522158766,-5.90147459332601,
13.));
#12741=CARTESIAN_POINT('Ctrl Pts',(-20.9780305852213,-5.9735089916636,13.));
#12742=CARTESIAN_POINT('Ctrl Pts',(-21.0471984394024,-6.04679718721607,
13.));
#12743=CARTESIAN_POINT('Ctrl Pts',(-21.1156584437795,-6.12131239523347,
13.));
#12744=CARTESIAN_POINT('Ctrl Pts',(-21.11960842029,-6.12561174233439,13.));
#12745=CARTESIAN_POINT('Ctrl Pts',(-21.1235560412392,-6.12991518820048,
13.));
#12746=CARTESIAN_POINT('Ctrl Pts',(-21.1275013067528,-6.1342227326009,13.));
#12747=CARTESIAN_POINT('Ctrl Pts',(-21.9890268624765,-0.694764450219579,
0.));
#12748=CARTESIAN_POINT('Ctrl Pts',(-21.9890268624765,-0.694764450219579,
21.));
#12749=CARTESIAN_POINT('Ctrl Pts',(-21.9799122315157,-0.699924103234221,
0.));
#12750=CARTESIAN_POINT('Ctrl Pts',(-21.9799122315157,-0.699924103234221,
21.));
#12751=CARTESIAN_POINT('Ctrl Pts',(-21.9616777523685,-0.710218621843554,
0.));
#12752=CARTESIAN_POINT('Ctrl Pts',(-21.9616777523685,-0.710218621843554,
21.));
#12753=CARTESIAN_POINT('Ctrl Pts',(-21.9343103819749,-0.725586037496633,
0.));
#12754=CARTESIAN_POINT('Ctrl Pts',(-21.9343103819749,-0.725586037496633,
21.));
#12755=CARTESIAN_POINT('Ctrl Pts',(-21.8977892409997,-0.74592715110982,
0.));
#12756=CARTESIAN_POINT('Ctrl Pts',(-21.8977892409997,-0.74592715110982,
21.));
#12757=CARTESIAN_POINT('Ctrl Pts',(-21.8520856039249,-0.771105213258328,
0.));
#12758=CARTESIAN_POINT('Ctrl Pts',(-21.8520856039249,-0.771105213258328,
21.));
#12759=CARTESIAN_POINT('Ctrl Pts',(-21.8063297959755,-0.796034321106411,
0.));
#12760=CARTESIAN_POINT('Ctrl Pts',(-21.8063297959755,-0.796034321106411,
21.));
#12761=CARTESIAN_POINT('Ctrl Pts',(-21.7605219769118,-0.820713597934076,
0.));
#12762=CARTESIAN_POINT('Ctrl Pts',(-21.7605219769118,-0.820713597934076,
21.));
#12763=CARTESIAN_POINT('Ctrl Pts',(-21.7146624809285,-0.845141916726556,
0.));
#12764=CARTESIAN_POINT('Ctrl Pts',(-21.7146624809285,-0.845141916726556,
21.));
#12765=CARTESIAN_POINT('Ctrl Pts',(-21.6687518829182,-0.869317897714098,
0.));
#12766=CARTESIAN_POINT('Ctrl Pts',(-21.6687518829182,-0.869317897714098,
21.));
#12767=CARTESIAN_POINT('Ctrl Pts',(-21.6227909401433,-0.89323996751367,
0.));
#12768=CARTESIAN_POINT('Ctrl Pts',(-21.6227909401433,-0.89323996751367,
21.));
#12769=CARTESIAN_POINT('Ctrl Pts',(-21.5767805209408,-0.916906425150852,
0.));
#12770=CARTESIAN_POINT('Ctrl Pts',(-21.5767805209408,-0.916906425150852,
21.));
#12771=CARTESIAN_POINT('Ctrl Pts',(-21.5307215366685,-0.940315509525148,
0.));
#12772=CARTESIAN_POINT('Ctrl Pts',(-21.5307215366685,-0.940315509525148,
21.));
#12773=CARTESIAN_POINT('Ctrl Pts',(-21.4846148770804,-0.96346546281577,
0.));
#12774=CARTESIAN_POINT('Ctrl Pts',(-21.4846148770804,-0.96346546281577,
21.));
#12775=CARTESIAN_POINT('Ctrl Pts',(-21.4384613333266,-0.986354611081132,
0.));
#12776=CARTESIAN_POINT('Ctrl Pts',(-21.4384613333266,-0.986354611081132,
21.));
#12777=CARTESIAN_POINT('Ctrl Pts',(-21.3922616124166,-1.00898133629988,
0.));
#12778=CARTESIAN_POINT('Ctrl Pts',(-21.3922616124166,-1.00898133629988,
21.));
#12779=CARTESIAN_POINT('Ctrl Pts',(-21.3460163737343,-1.03134402396953,
0.));
#12780=CARTESIAN_POINT('Ctrl Pts',(-21.3460163737343,-1.03134402396953,
21.));
#12781=CARTESIAN_POINT('Ctrl Pts',(-21.2997262593683,-1.05344101900192,
0.));
#12782=CARTESIAN_POINT('Ctrl Pts',(-21.2997262593683,-1.05344101900192,
21.));
#12783=CARTESIAN_POINT('Ctrl Pts',(-21.2533919248553,-1.07527058431887,
0.));
#12784=CARTESIAN_POINT('Ctrl Pts',(-21.2533919248553,-1.07527058431887,
21.));
#12785=CARTESIAN_POINT('Ctrl Pts',(-21.2070140764156,-1.09683084929266,
0.));
#12786=CARTESIAN_POINT('Ctrl Pts',(-21.2070140764156,-1.09683084929266,
21.));
#12787=CARTESIAN_POINT('Ctrl Pts',(-21.1605934684164,-1.11811982787746,
0.));
#12788=CARTESIAN_POINT('Ctrl Pts',(-21.1605934684164,-1.11811982787746,
21.));
#12789=CARTESIAN_POINT('Ctrl Pts',(-21.1141308858087,-1.13913546246555,
0.));
#12790=CARTESIAN_POINT('Ctrl Pts',(-21.1141308858087,-1.13913546246555,
21.));
#12791=CARTESIAN_POINT('Ctrl Pts',(-21.0676271313238,-1.15987566445807,
0.));
#12792=CARTESIAN_POINT('Ctrl Pts',(-21.0676271313238,-1.15987566445807,
21.));
#12793=CARTESIAN_POINT('Ctrl Pts',(-21.0210830121673,-1.18033835060894,
0.));
#12794=CARTESIAN_POINT('Ctrl Pts',(-21.0210830121673,-1.18033835060894,
21.));
#12795=CARTESIAN_POINT('Ctrl Pts',(-20.9744993243732,-1.20052150219503,
0.));
#12796=CARTESIAN_POINT('Ctrl Pts',(-20.9744993243732,-1.20052150219503,
21.));
#12797=CARTESIAN_POINT('Ctrl Pts',(-20.9278768531175,-1.22042312071096,
0.));
#12798=CARTESIAN_POINT('Ctrl Pts',(-20.9278768531175,-1.22042312071096,
21.));
#12799=CARTESIAN_POINT('Ctrl Pts',(-20.881216381382,-1.24004113517905,0.));
#12800=CARTESIAN_POINT('Ctrl Pts',(-20.881216381382,-1.24004113517905,21.));
#12801=CARTESIAN_POINT('Ctrl Pts',(-20.83451869657,-1.25937332001005,0.));
#12802=CARTESIAN_POINT('Ctrl Pts',(-20.83451869657,-1.25937332001005,21.));
#12803=CARTESIAN_POINT('Ctrl Pts',(-20.7877845975367,-1.27841722479262,
0.));
#12804=CARTESIAN_POINT('Ctrl Pts',(-20.7877845975367,-1.27841722479262,
21.));
#12805=CARTESIAN_POINT('Ctrl Pts',(-20.7410149035348,-1.29717006491149,
0.));
#12806=CARTESIAN_POINT('Ctrl Pts',(-20.7410149035348,-1.29717006491149,
21.));
#12807=CARTESIAN_POINT('Ctrl Pts',(-20.694210454218,-1.31562879653596,0.));
#12808=CARTESIAN_POINT('Ctrl Pts',(-20.694210454218,-1.31562879653596,21.));
#12809=CARTESIAN_POINT('Ctrl Pts',(-20.6473721041685,-1.3337902972259,0.));
#12810=CARTESIAN_POINT('Ctrl Pts',(-20.6473721041685,-1.3337902972259,21.));
#12811=CARTESIAN_POINT('Ctrl Pts',(-20.6005007190809,-1.35165153211252,
0.));
#12812=CARTESIAN_POINT('Ctrl Pts',(-20.6005007190809,-1.35165153211252,
21.));
#12813=CARTESIAN_POINT('Ctrl Pts',(-20.5535971721246,-1.36920969340018,
0.));
#12814=CARTESIAN_POINT('Ctrl Pts',(-20.5535971721246,-1.36920969340018,
21.));
#12815=CARTESIAN_POINT('Ctrl Pts',(-20.5066623390132,-1.38646244026049,
0.));
#12816=CARTESIAN_POINT('Ctrl Pts',(-20.5066623390132,-1.38646244026049,
21.));
#12817=CARTESIAN_POINT('Ctrl Pts',(-20.4596971004275,-1.40340771617024,
0.));
#12818=CARTESIAN_POINT('Ctrl Pts',(-20.4596971004275,-1.40340771617024,
21.));
#12819=CARTESIAN_POINT('Ctrl Pts',(-20.4127023494155,-1.4200432946371,0.));
#12820=CARTESIAN_POINT('Ctrl Pts',(-20.4127023494155,-1.4200432946371,21.));
#12821=CARTESIAN_POINT('Ctrl Pts',(-20.3656789980171,-1.43636637152782,
0.));
#12822=CARTESIAN_POINT('Ctrl Pts',(-20.3656789980171,-1.43636637152782,
21.));
#12823=CARTESIAN_POINT('Ctrl Pts',(-20.3186279833818,-1.45237321894403,
0.));
#12824=CARTESIAN_POINT('Ctrl Pts',(-20.3186279833818,-1.45237321894403,
21.));
#12825=CARTESIAN_POINT('Ctrl Pts',(-20.2715502770004,-1.46805861808021,
0.));
#12826=CARTESIAN_POINT('Ctrl Pts',(-20.2715502770004,-1.46805861808021,
21.));
#12827=CARTESIAN_POINT('Ctrl Pts',(-20.224446881308,-1.48341623961913,0.));
#12828=CARTESIAN_POINT('Ctrl Pts',(-20.224446881308,-1.48341623961913,21.));
#12829=CARTESIAN_POINT('Ctrl Pts',(-20.1773188177942,-1.49843965844502,
0.));
#12830=CARTESIAN_POINT('Ctrl Pts',(-20.1773188177942,-1.49843965844502,
21.));
#12831=CARTESIAN_POINT('Ctrl Pts',(-20.1301671167606,-1.51312326913583,
0.));
#12832=CARTESIAN_POINT('Ctrl Pts',(-20.1301671167606,-1.51312326913583,
21.));
#12833=CARTESIAN_POINT('Ctrl Pts',(-20.0829928089241,-1.52746305716964,
0.));
#12834=CARTESIAN_POINT('Ctrl Pts',(-20.0829928089241,-1.52746305716964,
21.));
#12835=CARTESIAN_POINT('Ctrl Pts',(-20.0357969106526,-1.54145790302917,
0.));
#12836=CARTESIAN_POINT('Ctrl Pts',(-20.0357969106526,-1.54145790302917,
21.));
#12837=CARTESIAN_POINT('Ctrl Pts',(-19.9885804375097,-1.55510860515913,
0.));
#12838=CARTESIAN_POINT('Ctrl Pts',(-19.9885804375097,-1.55510860515913,
21.));
#12839=CARTESIAN_POINT('Ctrl Pts',(-19.9413444362352,-1.56841542790452,
0.));
#12840=CARTESIAN_POINT('Ctrl Pts',(-19.9413444362352,-1.56841542790452,
21.));
#12841=CARTESIAN_POINT('Ctrl Pts',(-19.8940900137801,-1.58137589158952,
0.));
#12842=CARTESIAN_POINT('Ctrl Pts',(-19.8940900137801,-1.58137589158952,
21.));
#12843=CARTESIAN_POINT('Ctrl Pts',(-19.8468183626037,-1.59398289700559,
0.));
#12844=CARTESIAN_POINT('Ctrl Pts',(-19.8468183626037,-1.59398289700559,
21.));
#12845=CARTESIAN_POINT('Ctrl Pts',(-19.7995308006834,-1.60622162219699,
0.));
#12846=CARTESIAN_POINT('Ctrl Pts',(-19.7995308006834,-1.60622162219699,
21.));
#12847=CARTESIAN_POINT('Ctrl Pts',(-19.7522287462982,-1.61807191996833,
0.));
#12848=CARTESIAN_POINT('Ctrl Pts',(-19.7522287462982,-1.61807191996833,
21.));
#12849=CARTESIAN_POINT('Ctrl Pts',(-19.7049136553525,-1.62951389038421,
0.));
#12850=CARTESIAN_POINT('Ctrl Pts',(-19.7049136553525,-1.62951389038421,
21.));
#12851=CARTESIAN_POINT('Ctrl Pts',(-19.6575869645839,-1.64053294677821,
0.));
#12852=CARTESIAN_POINT('Ctrl Pts',(-19.6575869645839,-1.64053294677821,
21.));
#12853=CARTESIAN_POINT('Ctrl Pts',(-19.6102500448855,-1.65112409599282,
0.));
#12854=CARTESIAN_POINT('Ctrl Pts',(-19.6102500448855,-1.65112409599282,
21.));
#12855=CARTESIAN_POINT('Ctrl Pts',(-19.5629041190868,-1.66129908621006,
0.));
#12856=CARTESIAN_POINT('Ctrl Pts',(-19.5629041190868,-1.66129908621006,
21.));
#12857=CARTESIAN_POINT('Ctrl Pts',(-19.5155503513712,-1.67107974760948,
0.));
#12858=CARTESIAN_POINT('Ctrl Pts',(-19.5155503513712,-1.67107974760948,
21.));
#12859=CARTESIAN_POINT('Ctrl Pts',(-19.4681900187091,-1.68048476382294,
0.));
#12860=CARTESIAN_POINT('Ctrl Pts',(-19.4681900187091,-1.68048476382294,
21.));
#12861=CARTESIAN_POINT('Ctrl Pts',(-19.4208246682917,-1.6895175323357,0.));
#12862=CARTESIAN_POINT('Ctrl Pts',(-19.4208246682917,-1.6895175323357,21.));
#12863=CARTESIAN_POINT('Ctrl Pts',(-19.3734562555057,-1.69815571801252,
0.));
#12864=CARTESIAN_POINT('Ctrl Pts',(-19.3734562555057,-1.69815571801252,
21.));
#12865=CARTESIAN_POINT('Ctrl Pts',(-19.3260873558094,-1.70633457265124,
0.));
#12866=CARTESIAN_POINT('Ctrl Pts',(-19.3260873558094,-1.70633457265124,
21.));
#12867=CARTESIAN_POINT('Ctrl Pts',(-19.2787209722437,-1.71396454346262,
0.));
#12868=CARTESIAN_POINT('Ctrl Pts',(-19.2787209722437,-1.71396454346262,
21.));
#12869=CARTESIAN_POINT('Ctrl Pts',(-19.2313602042899,-1.72096104670234,
0.));
#12870=CARTESIAN_POINT('Ctrl Pts',(-19.2313602042899,-1.72096104670234,
21.));
#12871=CARTESIAN_POINT('Ctrl Pts',(-19.1840079312107,-1.72727220327098,
0.));
#12872=CARTESIAN_POINT('Ctrl Pts',(-19.1840079312107,-1.72727220327098,
21.));
#12873=CARTESIAN_POINT('Ctrl Pts',(-19.1366665585833,-1.73290313712353,
0.));
#12874=CARTESIAN_POINT('Ctrl Pts',(-19.1366665585833,-1.73290313712353,
21.));
#12875=CARTESIAN_POINT('Ctrl Pts',(-19.0893375576541,-1.7379530116984,0.));
#12876=CARTESIAN_POINT('Ctrl Pts',(-19.0893375576541,-1.7379530116984,21.));
#12877=CARTESIAN_POINT('Ctrl Pts',(-19.0420224296189,-1.74256297552949,
0.));
#12878=CARTESIAN_POINT('Ctrl Pts',(-19.0420224296189,-1.74256297552949,
21.));
#12879=CARTESIAN_POINT('Ctrl Pts',(-18.9947239970259,-1.74684309825012,
0.));
#12880=CARTESIAN_POINT('Ctrl Pts',(-18.9947239970259,-1.74684309825012,
21.));
#12881=CARTESIAN_POINT('Ctrl Pts',(-18.947447637865,-1.75080409924533,0.));
#12882=CARTESIAN_POINT('Ctrl Pts',(-18.947447637865,-1.75080409924533,21.));
#12883=CARTESIAN_POINT('Ctrl Pts',(-18.9002024267872,-1.75429229572775,
0.));
#12884=CARTESIAN_POINT('Ctrl Pts',(-18.9002024267872,-1.75429229572775,
21.));
#12885=CARTESIAN_POINT('Ctrl Pts',(-18.8530026395886,-1.75690876962597,
0.));
#12886=CARTESIAN_POINT('Ctrl Pts',(-18.8530026395886,-1.75690876962597,
21.));
#12887=CARTESIAN_POINT('Ctrl Pts',(-18.8058650094753,-1.7581175236483,0.));
#12888=CARTESIAN_POINT('Ctrl Pts',(-18.8058650094753,-1.7581175236483,21.));
#12889=CARTESIAN_POINT('Ctrl Pts',(-18.7682173836138,-1.75752447968136,
0.));
#12890=CARTESIAN_POINT('Ctrl Pts',(-18.7682173836138,-1.75752447968136,
21.));
#12891=CARTESIAN_POINT('Ctrl Pts',(-18.7400222442427,-1.75601041697575,
0.));
#12892=CARTESIAN_POINT('Ctrl Pts',(-18.7400222442427,-1.75601041697575,
21.));
#12893=CARTESIAN_POINT('Ctrl Pts',(-18.7212441956871,-1.75450132833463,
0.));
#12894=CARTESIAN_POINT('Ctrl Pts',(-18.7212441956871,-1.75450132833463,
21.));
#12895=CARTESIAN_POINT('Ctrl Pts',(-18.7118598491961,-1.75362185428836,
0.));
#12896=CARTESIAN_POINT('Ctrl Pts',(-18.7118598491961,-1.75362185428836,
21.));
#12897=CARTESIAN_POINT('',(-21.9890268624765,-0.694764450219644,0.));
#12898=CARTESIAN_POINT('Ctrl Pts',(-18.7118598491961,-1.75362185428836,
0.));
#12899=CARTESIAN_POINT('Ctrl Pts',(-18.7212441956871,-1.75450132833463,
0.));
#12900=CARTESIAN_POINT('Ctrl Pts',(-18.7400222442427,-1.75601041697575,
0.));
#12901=CARTESIAN_POINT('Ctrl Pts',(-18.7682173836138,-1.75752447968136,
0.));
#12902=CARTESIAN_POINT('Ctrl Pts',(-18.8058650094753,-1.7581175236483,0.));
#12903=CARTESIAN_POINT('Ctrl Pts',(-18.8530026395886,-1.75690876962597,
0.));
#12904=CARTESIAN_POINT('Ctrl Pts',(-18.9002024267872,-1.75429229572775,
0.));
#12905=CARTESIAN_POINT('Ctrl Pts',(-18.947447637865,-1.75080409924533,0.));
#12906=CARTESIAN_POINT('Ctrl Pts',(-18.9947239970259,-1.74684309825012,
0.));
#12907=CARTESIAN_POINT('Ctrl Pts',(-19.0420224296189,-1.74256297552949,
0.));
#12908=CARTESIAN_POINT('Ctrl Pts',(-19.0893375576541,-1.7379530116984,0.));
#12909=CARTESIAN_POINT('Ctrl Pts',(-19.1366665585833,-1.73290313712353,
0.));
#12910=CARTESIAN_POINT('Ctrl Pts',(-19.1840079312107,-1.72727220327098,
0.));
#12911=CARTESIAN_POINT('Ctrl Pts',(-19.2313602042899,-1.72096104670234,
0.));
#12912=CARTESIAN_POINT('Ctrl Pts',(-19.2787209722437,-1.71396454346262,
0.));
#12913=CARTESIAN_POINT('Ctrl Pts',(-19.3260873558094,-1.70633457265124,
0.));
#12914=CARTESIAN_POINT('Ctrl Pts',(-19.3734562555057,-1.69815571801252,
0.));
#12915=CARTESIAN_POINT('Ctrl Pts',(-19.4208246682917,-1.6895175323357,0.));
#12916=CARTESIAN_POINT('Ctrl Pts',(-19.4681900187091,-1.68048476382294,
0.));
#12917=CARTESIAN_POINT('Ctrl Pts',(-19.5155503513712,-1.67107974760948,
0.));
#12918=CARTESIAN_POINT('Ctrl Pts',(-19.5629041190868,-1.66129908621006,
0.));
#12919=CARTESIAN_POINT('Ctrl Pts',(-19.6102500448855,-1.65112409599282,
0.));
#12920=CARTESIAN_POINT('Ctrl Pts',(-19.6575869645839,-1.64053294677821,
0.));
#12921=CARTESIAN_POINT('Ctrl Pts',(-19.7049136553525,-1.62951389038421,
0.));
#12922=CARTESIAN_POINT('Ctrl Pts',(-19.7522287462982,-1.61807191996833,
0.));
#12923=CARTESIAN_POINT('Ctrl Pts',(-19.7995308006834,-1.60622162219699,
0.));
#12924=CARTESIAN_POINT('Ctrl Pts',(-19.8468183626037,-1.59398289700559,
0.));
#12925=CARTESIAN_POINT('Ctrl Pts',(-19.8940900137801,-1.58137589158952,
0.));
#12926=CARTESIAN_POINT('Ctrl Pts',(-19.9413444362352,-1.56841542790452,
0.));
#12927=CARTESIAN_POINT('Ctrl Pts',(-19.9885804375097,-1.55510860515913,
0.));
#12928=CARTESIAN_POINT('Ctrl Pts',(-20.0357969106526,-1.54145790302917,
0.));
#12929=CARTESIAN_POINT('Ctrl Pts',(-20.0829928089241,-1.52746305716964,
0.));
#12930=CARTESIAN_POINT('Ctrl Pts',(-20.1301671167606,-1.51312326913583,
0.));
#12931=CARTESIAN_POINT('Ctrl Pts',(-20.1773188177942,-1.49843965844502,
0.));
#12932=CARTESIAN_POINT('Ctrl Pts',(-20.224446881308,-1.48341623961913,0.));
#12933=CARTESIAN_POINT('Ctrl Pts',(-20.2715502770004,-1.46805861808021,
0.));
#12934=CARTESIAN_POINT('Ctrl Pts',(-20.3186279833818,-1.45237321894403,
0.));
#12935=CARTESIAN_POINT('Ctrl Pts',(-20.3656789980171,-1.43636637152782,
0.));
#12936=CARTESIAN_POINT('Ctrl Pts',(-20.4127023494155,-1.4200432946371,0.));
#12937=CARTESIAN_POINT('Ctrl Pts',(-20.4596971004275,-1.40340771617024,
0.));
#12938=CARTESIAN_POINT('Ctrl Pts',(-20.5066623390132,-1.38646244026049,
0.));
#12939=CARTESIAN_POINT('Ctrl Pts',(-20.5535971721246,-1.36920969340018,
0.));
#12940=CARTESIAN_POINT('Ctrl Pts',(-20.6005007190809,-1.35165153211252,
0.));
#12941=CARTESIAN_POINT('Ctrl Pts',(-20.6473721041685,-1.3337902972259,0.));
#12942=CARTESIAN_POINT('Ctrl Pts',(-20.694210454218,-1.31562879653596,0.));
#12943=CARTESIAN_POINT('Ctrl Pts',(-20.7410149035348,-1.29717006491149,
0.));
#12944=CARTESIAN_POINT('Ctrl Pts',(-20.7877845975367,-1.27841722479262,
0.));
#12945=CARTESIAN_POINT('Ctrl Pts',(-20.83451869657,-1.25937332001005,0.));
#12946=CARTESIAN_POINT('Ctrl Pts',(-20.881216381382,-1.24004113517905,0.));
#12947=CARTESIAN_POINT('Ctrl Pts',(-20.9278768531175,-1.22042312071096,
0.));
#12948=CARTESIAN_POINT('Ctrl Pts',(-20.9744993243732,-1.20052150219503,
0.));
#12949=CARTESIAN_POINT('Ctrl Pts',(-21.0210830121673,-1.18033835060894,
0.));
#12950=CARTESIAN_POINT('Ctrl Pts',(-21.0676271313238,-1.15987566445807,
0.));
#12951=CARTESIAN_POINT('Ctrl Pts',(-21.1141308858087,-1.13913546246555,
0.));
#12952=CARTESIAN_POINT('Ctrl Pts',(-21.1605934684164,-1.11811982787746,
0.));
#12953=CARTESIAN_POINT('Ctrl Pts',(-21.2070140764156,-1.09683084929266,
0.));
#12954=CARTESIAN_POINT('Ctrl Pts',(-21.2533919248553,-1.07527058431887,
0.));
#12955=CARTESIAN_POINT('Ctrl Pts',(-21.2997262593683,-1.05344101900192,
0.));
#12956=CARTESIAN_POINT('Ctrl Pts',(-21.3460163737343,-1.03134402396953,
0.));
#12957=CARTESIAN_POINT('Ctrl Pts',(-21.3922616124166,-1.00898133629988,
0.));
#12958=CARTESIAN_POINT('Ctrl Pts',(-21.4384613333266,-0.986354611081132,
0.));
#12959=CARTESIAN_POINT('Ctrl Pts',(-21.4846148770804,-0.96346546281577,
0.));
#12960=CARTESIAN_POINT('Ctrl Pts',(-21.5307215366685,-0.940315509525148,
0.));
#12961=CARTESIAN_POINT('Ctrl Pts',(-21.5767805209408,-0.916906425150852,
0.));
#12962=CARTESIAN_POINT('Ctrl Pts',(-21.6227909401433,-0.89323996751367,
0.));
#12963=CARTESIAN_POINT('Ctrl Pts',(-21.6687518829182,-0.869317897714098,
0.));
#12964=CARTESIAN_POINT('Ctrl Pts',(-21.7146624809285,-0.845141916726556,
0.));
#12965=CARTESIAN_POINT('Ctrl Pts',(-21.7605219769118,-0.820713597934076,
0.));
#12966=CARTESIAN_POINT('Ctrl Pts',(-21.8063297959755,-0.796034321106411,
0.));
#12967=CARTESIAN_POINT('Ctrl Pts',(-21.8612367655148,-0.766119391688711,
0.));
#12968=CARTESIAN_POINT('Ctrl Pts',(-21.9069273598709,-0.740879090965097,
0.));
#12969=CARTESIAN_POINT('Ctrl Pts',(-21.9434380560096,-0.720488353007145,
0.));
#12970=CARTESIAN_POINT('Ctrl Pts',(-21.970797600548,-0.705083756261758,
0.));
#12971=CARTESIAN_POINT('Ctrl Pts',(-21.9890268624765,-0.694764450219579,
0.));
#12972=CARTESIAN_POINT('',(-21.9890268624765,-0.694764450219644,13.));
#12973=CARTESIAN_POINT('Ctrl Pts',(-21.9890268624765,-0.694764450219579,
13.));
#12974=CARTESIAN_POINT('Ctrl Pts',(-21.8992923153509,-0.745561803243044,
13.));
#12975=CARTESIAN_POINT('Ctrl Pts',(-21.8092529632209,-0.794921865486053,
13.));
#12976=CARTESIAN_POINT('Ctrl Pts',(-21.71891375393,-0.84281926080538,13.));
#12977=CARTESIAN_POINT('Ctrl Pts',(-21.5692177628774,-0.92218732388059,
13.));
#12978=CARTESIAN_POINT('Ctrl Pts',(-21.418707272962,-0.997528955318343,
13.));
#12979=CARTESIAN_POINT('Ctrl Pts',(-21.267502258671,-1.06858105378788,13.));
#12980=CARTESIAN_POINT('Ctrl Pts',(-21.1512772179881,-1.12319586318391,
13.));
#12981=CARTESIAN_POINT('Ctrl Pts',(-21.034639156117,-1.17527598651002,13.));
#12982=CARTESIAN_POINT('Ctrl Pts',(-20.9176442431412,-1.22467603846418,
13.));
#12983=CARTESIAN_POINT('Ctrl Pts',(-20.7917020383065,-1.27785400410231,
13.));
#12984=CARTESIAN_POINT('Ctrl Pts',(-20.6653453745879,-1.32793259657608,
13.));
#12985=CARTESIAN_POINT('Ctrl Pts',(-20.5386490834973,-1.37465955678759,
13.));
#12986=CARTESIAN_POINT('Ctrl Pts',(-20.468506575479,-1.40052887113839,13.));
#12987=CARTESIAN_POINT('Ctrl Pts',(-20.3982600584712,-1.42537603682711,
13.));
#12988=CARTESIAN_POINT('Ctrl Pts',(-20.3279233191933,-1.44915458797959,
13.));
#12989=CARTESIAN_POINT('Ctrl Pts',(-20.2601440769455,-1.4720685330304,13.));
#12990=CARTESIAN_POINT('Ctrl Pts',(-20.1922811204785,-1.49398338578919,
13.));
#12991=CARTESIAN_POINT('Ctrl Pts',(-20.1243481778791,-1.51482335733726,
13.));
#12992=CARTESIAN_POINT('Ctrl Pts',(-20.0656332826906,-1.53283548368357,
13.));
#12993=CARTESIAN_POINT('Ctrl Pts',(-20.0068660712063,-1.55004791451012,
13.));
#12994=CARTESIAN_POINT('Ctrl Pts',(-19.9480555830993,-1.56645839157978,
13.));
#12995=CARTESIAN_POINT('Ctrl Pts',(-19.9058499566848,-1.5782354484752,13.));
#12996=CARTESIAN_POINT('Ctrl Pts',(-19.8636220199286,-1.58960230240354,
13.));
#12997=CARTESIAN_POINT('Ctrl Pts',(-19.8213758739716,-1.60051957233219,
13.));
#12998=CARTESIAN_POINT('Ctrl Pts',(-19.7798176538137,-1.61125906813568,
13.));
#12999=CARTESIAN_POINT('Ctrl Pts',(-19.7382418843902,-1.62155711742552,
13.));
#13000=CARTESIAN_POINT('Ctrl Pts',(-19.6966529616191,-1.63136143481693,
13.));
#13001=CARTESIAN_POINT('Ctrl Pts',(-19.6605929223136,-1.63986235397861,
13.));
#13002=CARTESIAN_POINT('Ctrl Pts',(-19.6245230263165,-1.6479896124833,13.));
#13003=CARTESIAN_POINT('Ctrl Pts',(-19.588445788193,-1.65575861448984,13.));
#13004=CARTESIAN_POINT('Ctrl Pts',(-19.5557680878316,-1.66279554782735,
13.));
#13005=CARTESIAN_POINT('Ctrl Pts',(-19.5230842951978,-1.66954412484817,
13.));
#13006=CARTESIAN_POINT('Ctrl Pts',(-19.4903963525255,-1.67602787924388,
13.));
#13007=CARTESIAN_POINT('Ctrl Pts',(-19.4628617563019,-1.68148945145379,
13.));
#13008=CARTESIAN_POINT('Ctrl Pts',(-19.4353241965609,-1.68676485594434,
13.));
#13009=CARTESIAN_POINT('Ctrl Pts',(-19.4077853966265,-1.69183425664604,
13.));
#13010=CARTESIAN_POINT('Ctrl Pts',(-19.3679337568149,-1.69917023102786,
13.));
#13011=CARTESIAN_POINT('Ctrl Pts',(-19.3280794804597,-1.70607400304717,
13.));
#13012=CARTESIAN_POINT('Ctrl Pts',(-19.2882303926777,-1.71232694125142,
13.));
#13013=CARTESIAN_POINT('Ctrl Pts',(-19.2641520278646,-1.71610520910184,
13.));
#13014=CARTESIAN_POINT('Ctrl Pts',(-19.2400756158948,-1.71964237036002,
13.));
#13015=CARTESIAN_POINT('Ctrl Pts',(-19.2160028184539,-1.72291205967493,
13.));
#13016=CARTESIAN_POINT('Ctrl Pts',(-19.1938009271133,-1.72592763304422,
13.));
#13017=CARTESIAN_POINT('Ctrl Pts',(-19.1716021268411,-1.72871436967926,
13.));
#13018=CARTESIAN_POINT('Ctrl Pts',(-19.1494073129248,-1.73129733452527,
13.));
#13019=CARTESIAN_POINT('Ctrl Pts',(-19.1188760970926,-1.73485046443652,
13.));
#13020=CARTESIAN_POINT('Ctrl Pts',(-19.088352219871,-1.73802530995722,13.));
#13021=CARTESIAN_POINT('Ctrl Pts',(-19.0578380259668,-1.74097263877159,
13.));
#13022=CARTESIAN_POINT('Ctrl Pts',(-19.0384792770416,-1.7428424767459,13.));
#13023=CARTESIAN_POINT('Ctrl Pts',(-19.0191244315082,-1.74462241724484,
13.));
#13024=CARTESIAN_POINT('Ctrl Pts',(-18.9997750006257,-1.74632097576469,
13.));
#13025=CARTESIAN_POINT('Ctrl Pts',(-18.9824097870453,-1.74784535297533,
13.));
#13026=CARTESIAN_POINT('Ctrl Pts',(-18.9650489251871,-1.74930491162087,
13.));
#13027=CARTESIAN_POINT('Ctrl Pts',(-18.9476944343333,-1.75066513119922,
13.));
#13028=CARTESIAN_POINT('Ctrl Pts',(-18.9294514080863,-1.75209499288047,
13.));
#13029=CARTESIAN_POINT('Ctrl Pts',(-18.911215425824,-1.75341524153972,13.));
#13030=CARTESIAN_POINT('Ctrl Pts',(-18.8929901413936,-1.75452347865236,
13.));
#13031=CARTESIAN_POINT('Ctrl Pts',(-18.8627179842862,-1.75636425804397,
13.));
#13032=CARTESIAN_POINT('Ctrl Pts',(-18.8324756678072,-1.75761169393937,
13.));
#13033=CARTESIAN_POINT('Ctrl Pts',(-18.8022820949953,-1.75764008468141,
13.));
#13034=CARTESIAN_POINT('Ctrl Pts',(-18.7856322843766,-1.75765574034698,
13.));
#13035=CARTESIAN_POINT('Ctrl Pts',(-18.7689972916915,-1.75729933637064,
13.));
#13036=CARTESIAN_POINT('Ctrl Pts',(-18.7523793043893,-1.75649392367919,
13.));
#13037=CARTESIAN_POINT('Ctrl Pts',(-18.7388614288228,-1.75583876199536,
13.));
#13038=CARTESIAN_POINT('Ctrl Pts',(-18.7253548001813,-1.75488656240187,
13.));
#13039=CARTESIAN_POINT('Ctrl Pts',(-18.7118598491961,-1.75362185428836,
13.));
#13040=CARTESIAN_POINT('',(-21.9890268624765,-0.694764450219644,0.));
#13041=CARTESIAN_POINT('Origin',(-5.6665783176868E-12,2.52435489670724E-28,
0.));
#13042=CARTESIAN_POINT('',(-21.9890268624765,0.694764450219584,0.));
#13043=CARTESIAN_POINT('Origin',(-5.6665783176868E-12,2.52435489670724E-28,
0.));
#13044=CARTESIAN_POINT('',(-21.9890268624765,0.694764450219584,13.));
#13045=CARTESIAN_POINT('Origin',(-5.6665783176868E-12,2.52435489670724E-28,
13.));
#13046=CARTESIAN_POINT('',(-21.9890268624765,0.694764450219584,0.));
#13047=CARTESIAN_POINT('Ctrl Pts',(-18.7118598491961,1.75362185428837,0.));
#13048=CARTESIAN_POINT('Ctrl Pts',(-18.7118598491961,1.75362185428837,21.));
#13049=CARTESIAN_POINT('Ctrl Pts',(-18.7212441956871,1.75450132833464,0.));
#13050=CARTESIAN_POINT('Ctrl Pts',(-18.7212441956871,1.75450132833464,21.));
#13051=CARTESIAN_POINT('Ctrl Pts',(-18.7400222442427,1.75601041697575,0.));
#13052=CARTESIAN_POINT('Ctrl Pts',(-18.7400222442427,1.75601041697575,21.));
#13053=CARTESIAN_POINT('Ctrl Pts',(-18.7682173836138,1.75752447968136,0.));
#13054=CARTESIAN_POINT('Ctrl Pts',(-18.7682173836138,1.75752447968136,21.));
#13055=CARTESIAN_POINT('Ctrl Pts',(-18.8058650094753,1.7581175236483,0.));
#13056=CARTESIAN_POINT('Ctrl Pts',(-18.8058650094753,1.7581175236483,21.));
#13057=CARTESIAN_POINT('Ctrl Pts',(-18.8530026395886,1.75690876962598,0.));
#13058=CARTESIAN_POINT('Ctrl Pts',(-18.8530026395886,1.75690876962598,21.));
#13059=CARTESIAN_POINT('Ctrl Pts',(-18.9002024267872,1.75429229572775,0.));
#13060=CARTESIAN_POINT('Ctrl Pts',(-18.9002024267872,1.75429229572775,21.));
#13061=CARTESIAN_POINT('Ctrl Pts',(-18.947447637865,1.75080409924533,0.));
#13062=CARTESIAN_POINT('Ctrl Pts',(-18.947447637865,1.75080409924533,21.));
#13063=CARTESIAN_POINT('Ctrl Pts',(-18.9947239970259,1.74684309825012,0.));
#13064=CARTESIAN_POINT('Ctrl Pts',(-18.9947239970259,1.74684309825012,21.));
#13065=CARTESIAN_POINT('Ctrl Pts',(-19.0420224296189,1.74256297552949,0.));
#13066=CARTESIAN_POINT('Ctrl Pts',(-19.0420224296189,1.74256297552949,21.));
#13067=CARTESIAN_POINT('Ctrl Pts',(-19.0893375576541,1.73795301169841,0.));
#13068=CARTESIAN_POINT('Ctrl Pts',(-19.0893375576541,1.73795301169841,21.));
#13069=CARTESIAN_POINT('Ctrl Pts',(-19.1366665585833,1.73290313712354,0.));
#13070=CARTESIAN_POINT('Ctrl Pts',(-19.1366665585833,1.73290313712354,21.));
#13071=CARTESIAN_POINT('Ctrl Pts',(-19.1840079312107,1.72727220327098,0.));
#13072=CARTESIAN_POINT('Ctrl Pts',(-19.1840079312107,1.72727220327098,21.));
#13073=CARTESIAN_POINT('Ctrl Pts',(-19.2313602042899,1.72096104670234,0.));
#13074=CARTESIAN_POINT('Ctrl Pts',(-19.2313602042899,1.72096104670234,21.));
#13075=CARTESIAN_POINT('Ctrl Pts',(-19.2787209722437,1.71396454346262,0.));
#13076=CARTESIAN_POINT('Ctrl Pts',(-19.2787209722437,1.71396454346262,21.));
#13077=CARTESIAN_POINT('Ctrl Pts',(-19.3260873558094,1.70633457265124,0.));
#13078=CARTESIAN_POINT('Ctrl Pts',(-19.3260873558094,1.70633457265124,21.));
#13079=CARTESIAN_POINT('Ctrl Pts',(-19.3734562555057,1.69815571801252,0.));
#13080=CARTESIAN_POINT('Ctrl Pts',(-19.3734562555057,1.69815571801252,21.));
#13081=CARTESIAN_POINT('Ctrl Pts',(-19.4208246682917,1.68951753233571,0.));
#13082=CARTESIAN_POINT('Ctrl Pts',(-19.4208246682917,1.68951753233571,21.));
#13083=CARTESIAN_POINT('Ctrl Pts',(-19.4681900187091,1.68048476382294,0.));
#13084=CARTESIAN_POINT('Ctrl Pts',(-19.4681900187091,1.68048476382294,21.));
#13085=CARTESIAN_POINT('Ctrl Pts',(-19.5155503513712,1.67107974760949,0.));
#13086=CARTESIAN_POINT('Ctrl Pts',(-19.5155503513712,1.67107974760949,21.));
#13087=CARTESIAN_POINT('Ctrl Pts',(-19.5629041190868,1.66129908621006,0.));
#13088=CARTESIAN_POINT('Ctrl Pts',(-19.5629041190868,1.66129908621006,21.));
#13089=CARTESIAN_POINT('Ctrl Pts',(-19.6102500448855,1.65112409599283,0.));
#13090=CARTESIAN_POINT('Ctrl Pts',(-19.6102500448855,1.65112409599283,21.));
#13091=CARTESIAN_POINT('Ctrl Pts',(-19.6575869645839,1.64053294677822,0.));
#13092=CARTESIAN_POINT('Ctrl Pts',(-19.6575869645839,1.64053294677822,21.));
#13093=CARTESIAN_POINT('Ctrl Pts',(-19.7049136553525,1.62951389038422,0.));
#13094=CARTESIAN_POINT('Ctrl Pts',(-19.7049136553525,1.62951389038422,21.));
#13095=CARTESIAN_POINT('Ctrl Pts',(-19.7522287462982,1.61807191996834,0.));
#13096=CARTESIAN_POINT('Ctrl Pts',(-19.7522287462982,1.61807191996834,21.));
#13097=CARTESIAN_POINT('Ctrl Pts',(-19.7995308006834,1.60622162219699,0.));
#13098=CARTESIAN_POINT('Ctrl Pts',(-19.7995308006834,1.60622162219699,21.));
#13099=CARTESIAN_POINT('Ctrl Pts',(-19.8468183626037,1.59398289700559,0.));
#13100=CARTESIAN_POINT('Ctrl Pts',(-19.8468183626037,1.59398289700559,21.));
#13101=CARTESIAN_POINT('Ctrl Pts',(-19.8940900137801,1.58137589158952,0.));
#13102=CARTESIAN_POINT('Ctrl Pts',(-19.8940900137801,1.58137589158952,21.));
#13103=CARTESIAN_POINT('Ctrl Pts',(-19.9413444362352,1.56841542790453,0.));
#13104=CARTESIAN_POINT('Ctrl Pts',(-19.9413444362352,1.56841542790453,21.));
#13105=CARTESIAN_POINT('Ctrl Pts',(-19.9885804375097,1.55510860515914,0.));
#13106=CARTESIAN_POINT('Ctrl Pts',(-19.9885804375097,1.55510860515914,21.));
#13107=CARTESIAN_POINT('Ctrl Pts',(-20.0357969106526,1.54145790302918,0.));
#13108=CARTESIAN_POINT('Ctrl Pts',(-20.0357969106526,1.54145790302918,21.));
#13109=CARTESIAN_POINT('Ctrl Pts',(-20.0829928089241,1.52746305716964,0.));
#13110=CARTESIAN_POINT('Ctrl Pts',(-20.0829928089241,1.52746305716964,21.));
#13111=CARTESIAN_POINT('Ctrl Pts',(-20.1301671167606,1.51312326913583,0.));
#13112=CARTESIAN_POINT('Ctrl Pts',(-20.1301671167606,1.51312326913583,21.));
#13113=CARTESIAN_POINT('Ctrl Pts',(-20.1773188177942,1.49843965844502,0.));
#13114=CARTESIAN_POINT('Ctrl Pts',(-20.1773188177942,1.49843965844502,21.));
#13115=CARTESIAN_POINT('Ctrl Pts',(-20.224446881308,1.48341623961914,0.));
#13116=CARTESIAN_POINT('Ctrl Pts',(-20.224446881308,1.48341623961914,21.));
#13117=CARTESIAN_POINT('Ctrl Pts',(-20.2715502770004,1.46805861808021,0.));
#13118=CARTESIAN_POINT('Ctrl Pts',(-20.2715502770004,1.46805861808021,21.));
#13119=CARTESIAN_POINT('Ctrl Pts',(-20.3186279833818,1.45237321894404,0.));
#13120=CARTESIAN_POINT('Ctrl Pts',(-20.3186279833818,1.45237321894404,21.));
#13121=CARTESIAN_POINT('Ctrl Pts',(-20.3656789980171,1.43636637152782,0.));
#13122=CARTESIAN_POINT('Ctrl Pts',(-20.3656789980171,1.43636637152782,21.));
#13123=CARTESIAN_POINT('Ctrl Pts',(-20.4127023494155,1.4200432946371,0.));
#13124=CARTESIAN_POINT('Ctrl Pts',(-20.4127023494155,1.4200432946371,21.));
#13125=CARTESIAN_POINT('Ctrl Pts',(-20.4596971004275,1.40340771617025,0.));
#13126=CARTESIAN_POINT('Ctrl Pts',(-20.4596971004275,1.40340771617025,21.));
#13127=CARTESIAN_POINT('Ctrl Pts',(-20.5066623390132,1.38646244026049,0.));
#13128=CARTESIAN_POINT('Ctrl Pts',(-20.5066623390132,1.38646244026049,21.));
#13129=CARTESIAN_POINT('Ctrl Pts',(-20.5535971721246,1.36920969340018,0.));
#13130=CARTESIAN_POINT('Ctrl Pts',(-20.5535971721246,1.36920969340018,21.));
#13131=CARTESIAN_POINT('Ctrl Pts',(-20.6005007190809,1.35165153211253,0.));
#13132=CARTESIAN_POINT('Ctrl Pts',(-20.6005007190809,1.35165153211253,21.));
#13133=CARTESIAN_POINT('Ctrl Pts',(-20.6473721041685,1.33379029722591,0.));
#13134=CARTESIAN_POINT('Ctrl Pts',(-20.6473721041685,1.33379029722591,21.));
#13135=CARTESIAN_POINT('Ctrl Pts',(-20.694210454218,1.31562879653596,0.));
#13136=CARTESIAN_POINT('Ctrl Pts',(-20.694210454218,1.31562879653596,21.));
#13137=CARTESIAN_POINT('Ctrl Pts',(-20.7410149035348,1.2971700649115,0.));
#13138=CARTESIAN_POINT('Ctrl Pts',(-20.7410149035348,1.2971700649115,21.));
#13139=CARTESIAN_POINT('Ctrl Pts',(-20.7877845975367,1.27841722479262,0.));
#13140=CARTESIAN_POINT('Ctrl Pts',(-20.7877845975367,1.27841722479262,21.));
#13141=CARTESIAN_POINT('Ctrl Pts',(-20.83451869657,1.25937332001005,0.));
#13142=CARTESIAN_POINT('Ctrl Pts',(-20.83451869657,1.25937332001005,21.));
#13143=CARTESIAN_POINT('Ctrl Pts',(-20.881216381382,1.24004113517905,0.));
#13144=CARTESIAN_POINT('Ctrl Pts',(-20.881216381382,1.24004113517905,21.));
#13145=CARTESIAN_POINT('Ctrl Pts',(-20.9278768531175,1.22042312071096,0.));
#13146=CARTESIAN_POINT('Ctrl Pts',(-20.9278768531175,1.22042312071096,21.));
#13147=CARTESIAN_POINT('Ctrl Pts',(-20.9744993243732,1.20052150219503,0.));
#13148=CARTESIAN_POINT('Ctrl Pts',(-20.9744993243732,1.20052150219503,21.));
#13149=CARTESIAN_POINT('Ctrl Pts',(-21.0210830121673,1.18033835060894,0.));
#13150=CARTESIAN_POINT('Ctrl Pts',(-21.0210830121673,1.18033835060894,21.));
#13151=CARTESIAN_POINT('Ctrl Pts',(-21.0676271313238,1.15987566445807,0.));
#13152=CARTESIAN_POINT('Ctrl Pts',(-21.0676271313238,1.15987566445807,21.));
#13153=CARTESIAN_POINT('Ctrl Pts',(-21.1141308858087,1.13913546246555,0.));
#13154=CARTESIAN_POINT('Ctrl Pts',(-21.1141308858087,1.13913546246555,21.));
#13155=CARTESIAN_POINT('Ctrl Pts',(-21.1605934684164,1.11811982787747,0.));
#13156=CARTESIAN_POINT('Ctrl Pts',(-21.1605934684164,1.11811982787747,21.));
#13157=CARTESIAN_POINT('Ctrl Pts',(-21.2070140764156,1.09683084929266,0.));
#13158=CARTESIAN_POINT('Ctrl Pts',(-21.2070140764156,1.09683084929266,21.));
#13159=CARTESIAN_POINT('Ctrl Pts',(-21.2533919248553,1.07527058431887,0.));
#13160=CARTESIAN_POINT('Ctrl Pts',(-21.2533919248553,1.07527058431887,21.));
#13161=CARTESIAN_POINT('Ctrl Pts',(-21.2997262593683,1.05344101900192,0.));
#13162=CARTESIAN_POINT('Ctrl Pts',(-21.2997262593683,1.05344101900192,21.));
#13163=CARTESIAN_POINT('Ctrl Pts',(-21.3460163737343,1.03134402396953,0.));
#13164=CARTESIAN_POINT('Ctrl Pts',(-21.3460163737343,1.03134402396953,21.));
#13165=CARTESIAN_POINT('Ctrl Pts',(-21.3922616124166,1.00898133629988,0.));
#13166=CARTESIAN_POINT('Ctrl Pts',(-21.3922616124166,1.00898133629988,21.));
#13167=CARTESIAN_POINT('Ctrl Pts',(-21.4384613333266,0.986354611081137,
0.));
#13168=CARTESIAN_POINT('Ctrl Pts',(-21.4384613333266,0.986354611081137,
21.));
#13169=CARTESIAN_POINT('Ctrl Pts',(-21.4846148770804,0.963465462815773,
0.));
#13170=CARTESIAN_POINT('Ctrl Pts',(-21.4846148770804,0.963465462815773,
21.));
#13171=CARTESIAN_POINT('Ctrl Pts',(-21.5307215366685,0.940315509525154,
0.));
#13172=CARTESIAN_POINT('Ctrl Pts',(-21.5307215366685,0.940315509525154,
21.));
#13173=CARTESIAN_POINT('Ctrl Pts',(-21.5767805209408,0.916906425150856,
0.));
#13174=CARTESIAN_POINT('Ctrl Pts',(-21.5767805209408,0.916906425150856,
21.));
#13175=CARTESIAN_POINT('Ctrl Pts',(-21.6227909401433,0.893239967513676,
0.));
#13176=CARTESIAN_POINT('Ctrl Pts',(-21.6227909401433,0.893239967513676,
21.));
#13177=CARTESIAN_POINT('Ctrl Pts',(-21.6687518829182,0.869317897714101,
0.));
#13178=CARTESIAN_POINT('Ctrl Pts',(-21.6687518829182,0.869317897714101,
21.));
#13179=CARTESIAN_POINT('Ctrl Pts',(-21.7146624809285,0.845141916726562,
0.));
#13180=CARTESIAN_POINT('Ctrl Pts',(-21.7146624809285,0.845141916726562,
21.));
#13181=CARTESIAN_POINT('Ctrl Pts',(-21.7605219769118,0.82071359793408,0.));
#13182=CARTESIAN_POINT('Ctrl Pts',(-21.7605219769118,0.82071359793408,21.));
#13183=CARTESIAN_POINT('Ctrl Pts',(-21.8063297959755,0.796034321106415,
0.));
#13184=CARTESIAN_POINT('Ctrl Pts',(-21.8063297959755,0.796034321106415,
21.));
#13185=CARTESIAN_POINT('Ctrl Pts',(-21.8520856039249,0.771105213258334,
0.));
#13186=CARTESIAN_POINT('Ctrl Pts',(-21.8520856039249,0.771105213258334,
21.));
#13187=CARTESIAN_POINT('Ctrl Pts',(-21.8977892409997,0.745927151109823,
0.));
#13188=CARTESIAN_POINT('Ctrl Pts',(-21.8977892409997,0.745927151109823,
21.));
#13189=CARTESIAN_POINT('Ctrl Pts',(-21.9343103819749,0.725586037496639,
0.));
#13190=CARTESIAN_POINT('Ctrl Pts',(-21.9343103819749,0.725586037496639,
21.));
#13191=CARTESIAN_POINT('Ctrl Pts',(-21.9616777523685,0.71021862184356,0.));
#13192=CARTESIAN_POINT('Ctrl Pts',(-21.9616777523685,0.71021862184356,21.));
#13193=CARTESIAN_POINT('Ctrl Pts',(-21.9799122315157,0.699924103234225,
0.));
#13194=CARTESIAN_POINT('Ctrl Pts',(-21.9799122315157,0.699924103234225,
21.));
#13195=CARTESIAN_POINT('Ctrl Pts',(-21.9890268624765,0.694764450219583,
0.));
#13196=CARTESIAN_POINT('Ctrl Pts',(-21.9890268624765,0.694764450219583,
21.));
#13197=CARTESIAN_POINT('Ctrl Pts',(-18.7118598491961,1.75362185428837,0.));
#13198=CARTESIAN_POINT('Ctrl Pts',(-18.7212441956871,1.75450132833464,0.));
#13199=CARTESIAN_POINT('Ctrl Pts',(-18.7400222442427,1.75601041697575,0.));
#13200=CARTESIAN_POINT('Ctrl Pts',(-18.7682173836138,1.75752447968136,0.));
#13201=CARTESIAN_POINT('Ctrl Pts',(-18.8058650094753,1.7581175236483,0.));
#13202=CARTESIAN_POINT('Ctrl Pts',(-18.8530026395886,1.75690876962598,0.));
#13203=CARTESIAN_POINT('Ctrl Pts',(-18.9002024267872,1.75429229572775,0.));
#13204=CARTESIAN_POINT('Ctrl Pts',(-18.947447637865,1.75080409924533,0.));
#13205=CARTESIAN_POINT('Ctrl Pts',(-18.9947239970259,1.74684309825012,0.));
#13206=CARTESIAN_POINT('Ctrl Pts',(-19.0420224296189,1.74256297552949,0.));
#13207=CARTESIAN_POINT('Ctrl Pts',(-19.0893375576541,1.73795301169841,0.));
#13208=CARTESIAN_POINT('Ctrl Pts',(-19.1366665585833,1.73290313712354,0.));
#13209=CARTESIAN_POINT('Ctrl Pts',(-19.1840079312107,1.72727220327098,0.));
#13210=CARTESIAN_POINT('Ctrl Pts',(-19.2313602042899,1.72096104670234,0.));
#13211=CARTESIAN_POINT('Ctrl Pts',(-19.2787209722437,1.71396454346262,0.));
#13212=CARTESIAN_POINT('Ctrl Pts',(-19.3260873558094,1.70633457265124,0.));
#13213=CARTESIAN_POINT('Ctrl Pts',(-19.3734562555057,1.69815571801252,0.));
#13214=CARTESIAN_POINT('Ctrl Pts',(-19.4208246682917,1.68951753233571,0.));
#13215=CARTESIAN_POINT('Ctrl Pts',(-19.4681900187091,1.68048476382294,0.));
#13216=CARTESIAN_POINT('Ctrl Pts',(-19.5155503513712,1.67107974760949,0.));
#13217=CARTESIAN_POINT('Ctrl Pts',(-19.5629041190868,1.66129908621006,0.));
#13218=CARTESIAN_POINT('Ctrl Pts',(-19.6102500448855,1.65112409599283,0.));
#13219=CARTESIAN_POINT('Ctrl Pts',(-19.6575869645839,1.64053294677822,0.));
#13220=CARTESIAN_POINT('Ctrl Pts',(-19.7049136553525,1.62951389038422,0.));
#13221=CARTESIAN_POINT('Ctrl Pts',(-19.7522287462982,1.61807191996834,0.));
#13222=CARTESIAN_POINT('Ctrl Pts',(-19.7995308006834,1.60622162219699,0.));
#13223=CARTESIAN_POINT('Ctrl Pts',(-19.8468183626037,1.59398289700559,0.));
#13224=CARTESIAN_POINT('Ctrl Pts',(-19.8940900137801,1.58137589158952,0.));
#13225=CARTESIAN_POINT('Ctrl Pts',(-19.9413444362352,1.56841542790453,0.));
#13226=CARTESIAN_POINT('Ctrl Pts',(-19.9885804375097,1.55510860515914,0.));
#13227=CARTESIAN_POINT('Ctrl Pts',(-20.0357969106526,1.54145790302918,0.));
#13228=CARTESIAN_POINT('Ctrl Pts',(-20.0829928089241,1.52746305716964,0.));
#13229=CARTESIAN_POINT('Ctrl Pts',(-20.1301671167606,1.51312326913583,0.));
#13230=CARTESIAN_POINT('Ctrl Pts',(-20.1773188177942,1.49843965844502,0.));
#13231=CARTESIAN_POINT('Ctrl Pts',(-20.224446881308,1.48341623961914,0.));
#13232=CARTESIAN_POINT('Ctrl Pts',(-20.2715502770004,1.46805861808021,0.));
#13233=CARTESIAN_POINT('Ctrl Pts',(-20.3186279833818,1.45237321894404,0.));
#13234=CARTESIAN_POINT('Ctrl Pts',(-20.3656789980171,1.43636637152782,0.));
#13235=CARTESIAN_POINT('Ctrl Pts',(-20.4127023494155,1.4200432946371,0.));
#13236=CARTESIAN_POINT('Ctrl Pts',(-20.4596971004275,1.40340771617025,0.));
#13237=CARTESIAN_POINT('Ctrl Pts',(-20.5066623390132,1.38646244026049,0.));
#13238=CARTESIAN_POINT('Ctrl Pts',(-20.5535971721246,1.36920969340018,0.));
#13239=CARTESIAN_POINT('Ctrl Pts',(-20.6005007190809,1.35165153211253,0.));
#13240=CARTESIAN_POINT('Ctrl Pts',(-20.6473721041685,1.33379029722591,0.));
#13241=CARTESIAN_POINT('Ctrl Pts',(-20.694210454218,1.31562879653596,0.));
#13242=CARTESIAN_POINT('Ctrl Pts',(-20.7410149035348,1.2971700649115,0.));
#13243=CARTESIAN_POINT('Ctrl Pts',(-20.7877845975367,1.27841722479262,0.));
#13244=CARTESIAN_POINT('Ctrl Pts',(-20.83451869657,1.25937332001005,0.));
#13245=CARTESIAN_POINT('Ctrl Pts',(-20.881216381382,1.24004113517905,0.));
#13246=CARTESIAN_POINT('Ctrl Pts',(-20.9278768531175,1.22042312071096,0.));
#13247=CARTESIAN_POINT('Ctrl Pts',(-20.9744993243732,1.20052150219503,0.));
#13248=CARTESIAN_POINT('Ctrl Pts',(-21.0210830121673,1.18033835060894,0.));
#13249=CARTESIAN_POINT('Ctrl Pts',(-21.0676271313238,1.15987566445807,0.));
#13250=CARTESIAN_POINT('Ctrl Pts',(-21.1141308858087,1.13913546246555,0.));
#13251=CARTESIAN_POINT('Ctrl Pts',(-21.1605934684164,1.11811982787747,0.));
#13252=CARTESIAN_POINT('Ctrl Pts',(-21.2070140764156,1.09683084929266,0.));
#13253=CARTESIAN_POINT('Ctrl Pts',(-21.2533919248553,1.07527058431887,0.));
#13254=CARTESIAN_POINT('Ctrl Pts',(-21.2997262593683,1.05344101900192,0.));
#13255=CARTESIAN_POINT('Ctrl Pts',(-21.3460163737343,1.03134402396953,0.));
#13256=CARTESIAN_POINT('Ctrl Pts',(-21.3922616124166,1.00898133629988,0.));
#13257=CARTESIAN_POINT('Ctrl Pts',(-21.4384613333266,0.986354611081137,
0.));
#13258=CARTESIAN_POINT('Ctrl Pts',(-21.4846148770804,0.963465462815773,
0.));
#13259=CARTESIAN_POINT('Ctrl Pts',(-21.5307215366685,0.940315509525154,
0.));
#13260=CARTESIAN_POINT('Ctrl Pts',(-21.5767805209408,0.916906425150856,
0.));
#13261=CARTESIAN_POINT('Ctrl Pts',(-21.6227909401433,0.893239967513676,
0.));
#13262=CARTESIAN_POINT('Ctrl Pts',(-21.6687518829182,0.869317897714101,
0.));
#13263=CARTESIAN_POINT('Ctrl Pts',(-21.7146624809285,0.845141916726562,
0.));
#13264=CARTESIAN_POINT('Ctrl Pts',(-21.7605219769118,0.82071359793408,0.));
#13265=CARTESIAN_POINT('Ctrl Pts',(-21.8063297959755,0.796034321106415,
0.));
#13266=CARTESIAN_POINT('Ctrl Pts',(-21.8612367655148,0.766119391688717,
0.));
#13267=CARTESIAN_POINT('Ctrl Pts',(-21.9069273598709,0.740879090965099,
0.));
#13268=CARTESIAN_POINT('Ctrl Pts',(-21.9434380560096,0.720488353007152,
0.));
#13269=CARTESIAN_POINT('Ctrl Pts',(-21.970797600548,0.705083756261763,0.));
#13270=CARTESIAN_POINT('Ctrl Pts',(-21.9890268624765,0.694764450219583,
0.));
#13271=CARTESIAN_POINT('Ctrl Pts',(-18.7118598491961,1.75362185428837,13.));
#13272=CARTESIAN_POINT('Ctrl Pts',(-18.7276767707249,1.75510417082366,13.));
#13273=CARTESIAN_POINT('Ctrl Pts',(-18.743509767289,1.75615601189424,13.));
#13274=CARTESIAN_POINT('Ctrl Pts',(-18.7593580381833,1.75680608702495,13.));
#13275=CARTESIAN_POINT('Ctrl Pts',(-18.77793339704,1.7575680237004,13.));
#13276=CARTESIAN_POINT('Ctrl Pts',(-18.796529725069,1.7577788791906,13.));
#13277=CARTESIAN_POINT('Ctrl Pts',(-18.8151436576367,1.75755628860693,13.));
#13278=CARTESIAN_POINT('Ctrl Pts',(-18.841334351583,1.75724309300298,13.));
#13279=CARTESIAN_POINT('Ctrl Pts',(-18.867559770113,1.75607893899574,13.));
#13280=CARTESIAN_POINT('Ctrl Pts',(-18.8938074357206,1.75447363677639,13.));
#13281=CARTESIAN_POINT('Ctrl Pts',(-18.9112662729044,1.75340585762614,13.));
#13282=CARTESIAN_POINT('Ctrl Pts',(-18.9287348768902,1.7521449293594,13.));
#13283=CARTESIAN_POINT('Ctrl Pts',(-18.9462100283356,1.75078122387574,13.));
#13284=CARTESIAN_POINT('Ctrl Pts',(-18.9646054898197,1.74934570031083,13.));
#13285=CARTESIAN_POINT('Ctrl Pts',(-18.9830081805109,1.74779717198811,13.));
#13286=CARTESIAN_POINT('Ctrl Pts',(-19.0014156957841,1.74617674699249,13.));
#13287=CARTESIAN_POINT('Ctrl Pts',(-19.0218582491316,1.74437717633198,13.));
#13288=CARTESIAN_POINT('Ctrl Pts',(-19.0423067706102,1.7424876259601,13.));
#13289=CARTESIAN_POINT('Ctrl Pts',(-19.0627595477341,1.74049525500348,13.));
#13290=CARTESIAN_POINT('Ctrl Pts',(-19.0935931019431,1.73749165908478,13.));
#13291=CARTESIAN_POINT('Ctrl Pts',(-19.124436353955,1.73424805120453,13.));
#13292=CARTESIAN_POINT('Ctrl Pts',(-19.155287003777,1.73060838684868,13.));
#13293=CARTESIAN_POINT('Ctrl Pts',(-19.1776993264081,1.72796425026539,13.));
#13294=CARTESIAN_POINT('Ctrl Pts',(-19.2001156538104,1.72510779282378,13.));
#13295=CARTESIAN_POINT('Ctrl Pts',(-19.2225350169938,1.72201836571105,13.));
#13296=CARTESIAN_POINT('Ctrl Pts',(-19.2499407687534,1.71824180560815,13.));
#13297=CARTESIAN_POINT('Ctrl Pts',(-19.2773510352597,1.71411839343645,13.));
#13298=CARTESIAN_POINT('Ctrl Pts',(-19.3047632983727,1.70969587297193,13.));
#13299=CARTESIAN_POINT('Ctrl Pts',(-19.3343730920364,1.70491881688253,13.));
#13300=CARTESIAN_POINT('Ctrl Pts',(-19.3639851445252,1.69979875336516,13.));
#13301=CARTESIAN_POINT('Ctrl Pts',(-19.3935962281375,1.69442732753347,13.));
#13302=CARTESIAN_POINT('Ctrl Pts',(-19.4209330414363,1.68946845243685,13.));
#13303=CARTESIAN_POINT('Ctrl Pts',(-19.448269005347,1.68429785630172,13.));
#13304=CARTESIAN_POINT('Ctrl Pts',(-19.4756022976243,1.67894398811971,13.));
#13305=CARTESIAN_POINT('Ctrl Pts',(-19.5127359786207,1.67167048329817,13.));
#13306=CARTESIAN_POINT('Ctrl Pts',(-19.5498647402244,1.66405675112121,13.));
#13307=CARTESIAN_POINT('Ctrl Pts',(-19.5869856493979,1.65607285222827,13.));
#13308=CARTESIAN_POINT('Ctrl Pts',(-19.6228065250069,1.64836856223413,13.));
#13309=CARTESIAN_POINT('Ctrl Pts',(-19.6586201923617,1.64031177032422,13.));
#13310=CARTESIAN_POINT('Ctrl Pts',(-19.6944241981293,1.63188637918844,13.));
#13311=CARTESIAN_POINT('Ctrl Pts',(-19.7430649431878,1.62044024925217,13.));
#13312=CARTESIAN_POINT('Ctrl Pts',(-19.7916877990604,1.60831707818014,13.));
#13313=CARTESIAN_POINT('Ctrl Pts',(-19.8402857466125,1.59560243913608,13.));
#13314=CARTESIAN_POINT('Ctrl Pts',(-19.8830022860036,1.58442654782939,13.));
#13315=CARTESIAN_POINT('Ctrl Pts',(-19.9256995150218,1.5728005280582,13.));
#13316=CARTESIAN_POINT('Ctrl Pts',(-19.9683733417696,1.56075644050925,13.));
#13317=CARTESIAN_POINT('Ctrl Pts',(-20.0312849226892,1.54300053141499,13.));
#13318=CARTESIAN_POINT('Ctrl Pts',(-20.0941457150012,1.52432694533036,13.));
#13319=CARTESIAN_POINT('Ctrl Pts',(-20.1569447710111,1.50474000384183,13.));
#13320=CARTESIAN_POINT('Ctrl Pts',(-20.236197792604,1.48002109251801,13.));
#13321=CARTESIAN_POINT('Ctrl Pts',(-20.3153523889882,1.45385270862993,13.));
#13322=CARTESIAN_POINT('Ctrl Pts',(-20.3943871107868,1.42635858933979,13.));
#13323=CARTESIAN_POINT('Ctrl Pts',(-20.501445734804,1.3891156850468,13.));
#13324=CARTESIAN_POINT('Ctrl Pts',(-20.6082844519781,1.34943433503116,13.));
#13325=CARTESIAN_POINT('Ctrl Pts',(-20.7148563913884,1.30744723530953,13.));
#13326=CARTESIAN_POINT('Ctrl Pts',(-20.8098680661395,1.27001463640438,13.));
#13327=CARTESIAN_POINT('Ctrl Pts',(-20.9046675819257,1.23075788115688,13.));
#13328=CARTESIAN_POINT('Ctrl Pts',(-20.9992246138437,1.18977154285938,13.));
#13329=CARTESIAN_POINT('Ctrl Pts',(-21.1332379309096,1.13168263039858,13.));
#13330=CARTESIAN_POINT('Ctrl Pts',(-21.2667633190703,1.07011397729315,13.));
#13331=CARTESIAN_POINT('Ctrl Pts',(-21.399720077537,1.00527632074311,13.));
#13332=CARTESIAN_POINT('Ctrl Pts',(-21.5029977299653,0.954911968944342,
13.));
#13333=CARTESIAN_POINT('Ctrl Pts',(-21.6059349891428,0.902570955669054,
13.));
#13334=CARTESIAN_POINT('Ctrl Pts',(-21.7084903368843,0.848338494786424,
13.));
#13335=CARTESIAN_POINT('Ctrl Pts',(-21.7972084624612,0.801423317948843,
13.));
#13336=CARTESIAN_POINT('Ctrl Pts',(-21.8856382926503,0.753096148034919,
13.));
#13337=CARTESIAN_POINT('Ctrl Pts',(-21.9737740854159,0.703383282495547,
13.));
#13338=CARTESIAN_POINT('Ctrl Pts',(-21.9788593181079,0.700514964402279,
13.));
#13339=CARTESIAN_POINT('Ctrl Pts',(-21.983943577112,0.697642020224148,13.));
#13340=CARTESIAN_POINT('Ctrl Pts',(-21.9890268624765,0.694764450219584,
13.));
#13341=CARTESIAN_POINT('Ctrl Pts',(-21.1275013067528,6.1342227326009,0.));
#13342=CARTESIAN_POINT('Ctrl Pts',(-21.1275013067528,6.1342227326009,21.));
#13343=CARTESIAN_POINT('Ctrl Pts',(-21.1204271980506,6.12649903511517,0.));
#13344=CARTESIAN_POINT('Ctrl Pts',(-21.1204271980506,6.12649903511517,21.));
#13345=CARTESIAN_POINT('Ctrl Pts',(-21.1062663590356,6.11107360216958,0.));
#13346=CARTESIAN_POINT('Ctrl Pts',(-21.1062663590356,6.11107360216958,21.));
#13347=CARTESIAN_POINT('Ctrl Pts',(-21.0849872356853,6.08800133883114,0.));
#13348=CARTESIAN_POINT('Ctrl Pts',(-21.0849872356853,6.08800133883114,21.));
#13349=CARTESIAN_POINT('Ctrl Pts',(-21.0565393163693,6.05737013696533,0.));
#13350=CARTESIAN_POINT('Ctrl Pts',(-21.0565393163693,6.05737013696533,21.));
#13351=CARTESIAN_POINT('Ctrl Pts',(-21.0208530236003,6.01930117633045,0.));
#13352=CARTESIAN_POINT('Ctrl Pts',(-21.0208530236003,6.01930117633045,21.));
#13353=CARTESIAN_POINT('Ctrl Pts',(-20.9850401822713,5.98145286361837,0.));
#13354=CARTESIAN_POINT('Ctrl Pts',(-20.9850401822713,5.98145286361837,21.));
#13355=CARTESIAN_POINT('Ctrl Pts',(-20.9491006734021,5.94382608200804,0.));
#13356=CARTESIAN_POINT('Ctrl Pts',(-20.9491006734021,5.94382608200804,21.));
#13357=CARTESIAN_POINT('Ctrl Pts',(-20.9130344665641,5.906422006626,0.));
#13358=CARTESIAN_POINT('Ctrl Pts',(-20.9130344665641,5.906422006626,21.));
#13359=CARTESIAN_POINT('Ctrl Pts',(-20.8768416821402,5.86924212736288,0.));
#13360=CARTESIAN_POINT('Ctrl Pts',(-20.8768416821402,5.86924212736288,21.));
#13361=CARTESIAN_POINT('Ctrl Pts',(-20.8405225541277,5.83228817460178,0.));
#13362=CARTESIAN_POINT('Ctrl Pts',(-20.8405225541277,5.83228817460178,21.));
#13363=CARTESIAN_POINT('Ctrl Pts',(-20.8040773827343,5.79556203439644,0.));
#13364=CARTESIAN_POINT('Ctrl Pts',(-20.8040773827343,5.79556203439644,21.));
#13365=CARTESIAN_POINT('Ctrl Pts',(-20.7675064905026,5.75906566327796,0.));
#13366=CARTESIAN_POINT('Ctrl Pts',(-20.7675064905026,5.75906566327796,21.));
#13367=CARTESIAN_POINT('Ctrl Pts',(-20.7308101804425,5.72280100798241,0.));
#13368=CARTESIAN_POINT('Ctrl Pts',(-20.7308101804425,5.72280100798241,21.));
#13369=CARTESIAN_POINT('Ctrl Pts',(-20.6939886877061,5.68676990500163,0.));
#13370=CARTESIAN_POINT('Ctrl Pts',(-20.6939886877061,5.68676990500163,21.));
#13371=CARTESIAN_POINT('Ctrl Pts',(-20.6570421847033,5.65097411164335,0.));
#13372=CARTESIAN_POINT('Ctrl Pts',(-20.6570421847033,5.65097411164335,21.));
#13373=CARTESIAN_POINT('Ctrl Pts',(-20.6199707996366,5.61541536715149,0.));
#13374=CARTESIAN_POINT('Ctrl Pts',(-20.6199707996366,5.61541536715149,21.));
#13375=CARTESIAN_POINT('Ctrl Pts',(-20.5827746317185,5.58009544402475,0.));
#13376=CARTESIAN_POINT('Ctrl Pts',(-20.5827746317185,5.58009544402475,21.));
#13377=CARTESIAN_POINT('Ctrl Pts',(-20.5454537676144,5.5450161968946,0.));
#13378=CARTESIAN_POINT('Ctrl Pts',(-20.5454537676144,5.5450161968946,21.));
#13379=CARTESIAN_POINT('Ctrl Pts',(-20.5080083009242,5.51017962306782,0.));
#13380=CARTESIAN_POINT('Ctrl Pts',(-20.5080083009242,5.51017962306782,21.));
#13381=CARTESIAN_POINT('Ctrl Pts',(-20.4704383353718,5.47558784449851,0.));
#13382=CARTESIAN_POINT('Ctrl Pts',(-20.4704383353718,5.47558784449851,21.));
#13383=CARTESIAN_POINT('Ctrl Pts',(-20.4327439816542,5.44124306065111,0.));
#13384=CARTESIAN_POINT('Ctrl Pts',(-20.4327439816542,5.44124306065111,21.));
#13385=CARTESIAN_POINT('Ctrl Pts',(-20.3949253578015,5.40714750595875,0.));
#13386=CARTESIAN_POINT('Ctrl Pts',(-20.3949253578015,5.40714750595875,21.));
#13387=CARTESIAN_POINT('Ctrl Pts',(-20.3569825877537,5.37330341114649,0.));
#13388=CARTESIAN_POINT('Ctrl Pts',(-20.3569825877537,5.37330341114649,21.));
#13389=CARTESIAN_POINT('Ctrl Pts',(-20.3189158047642,5.33971294212214,0.));
#13390=CARTESIAN_POINT('Ctrl Pts',(-20.3189158047642,5.33971294212214,21.));
#13391=CARTESIAN_POINT('Ctrl Pts',(-20.2807251380077,5.30637824220997,0.));
#13392=CARTESIAN_POINT('Ctrl Pts',(-20.2807251380077,5.30637824220997,21.));
#13393=CARTESIAN_POINT('Ctrl Pts',(-20.2424106921768,5.2733015229815,0.));
#13394=CARTESIAN_POINT('Ctrl Pts',(-20.2424106921768,5.2733015229815,21.));
#13395=CARTESIAN_POINT('Ctrl Pts',(-20.2039725283917,5.2404851444189,0.));
#13396=CARTESIAN_POINT('Ctrl Pts',(-20.2039725283917,5.2404851444189,21.));
#13397=CARTESIAN_POINT('Ctrl Pts',(-20.1654106491899,5.20793168386163,0.));
#13398=CARTESIAN_POINT('Ctrl Pts',(-20.1654106491899,5.20793168386163,21.));
#13399=CARTESIAN_POINT('Ctrl Pts',(-20.1267249732337,5.17564404279922,0.));
#13400=CARTESIAN_POINT('Ctrl Pts',(-20.1267249732337,5.17564404279922,21.));
#13401=CARTESIAN_POINT('Ctrl Pts',(-20.087915358486,5.14362537555398,0.));
#13402=CARTESIAN_POINT('Ctrl Pts',(-20.087915358486,5.14362537555398,21.));
#13403=CARTESIAN_POINT('Ctrl Pts',(-20.0489816528155,5.11187891582335,0.));
#13404=CARTESIAN_POINT('Ctrl Pts',(-20.0489816528155,5.11187891582335,21.));
#13405=CARTESIAN_POINT('Ctrl Pts',(-20.0099237417205,5.08040781745336,0.));
#13406=CARTESIAN_POINT('Ctrl Pts',(-20.0099237417205,5.08040781745336,21.));
#13407=CARTESIAN_POINT('Ctrl Pts',(-19.9707415879783,5.04921502064063,0.));
#13408=CARTESIAN_POINT('Ctrl Pts',(-19.9707415879783,5.04921502064063,21.));
#13409=CARTESIAN_POINT('Ctrl Pts',(-19.931435301086,5.01830302225557,0.));
#13410=CARTESIAN_POINT('Ctrl Pts',(-19.931435301086,5.01830302225557,21.));
#13411=CARTESIAN_POINT('Ctrl Pts',(-19.8920050831202,4.98767405031333,0.));
#13412=CARTESIAN_POINT('Ctrl Pts',(-19.8920050831202,4.98767405031333,21.));
#13413=CARTESIAN_POINT('Ctrl Pts',(-19.8524510953961,4.95733049830096,0.));
#13414=CARTESIAN_POINT('Ctrl Pts',(-19.8524510953961,4.95733049830096,21.));
#13415=CARTESIAN_POINT('Ctrl Pts',(-19.8127733387903,4.92727531494347,0.));
#13416=CARTESIAN_POINT('Ctrl Pts',(-19.8127733387903,4.92727531494347,21.));
#13417=CARTESIAN_POINT('Ctrl Pts',(-19.772971552601,4.89751233527804,0.));
#13418=CARTESIAN_POINT('Ctrl Pts',(-19.772971552601,4.89751233527804,21.));
#13419=CARTESIAN_POINT('Ctrl Pts',(-19.7330450480715,4.86804682289087,0.));
#13420=CARTESIAN_POINT('Ctrl Pts',(-19.7330450480715,4.86804682289087,21.));
#13421=CARTESIAN_POINT('Ctrl Pts',(-19.6929928227072,4.83888510708974,0.));
#13422=CARTESIAN_POINT('Ctrl Pts',(-19.6929928227072,4.83888510708974,21.));
#13423=CARTESIAN_POINT('Ctrl Pts',(-19.6528138625329,4.81003361418061,0.));
#13424=CARTESIAN_POINT('Ctrl Pts',(-19.6528138625329,4.81003361418061,21.));
#13425=CARTESIAN_POINT('Ctrl Pts',(-19.6125074152527,4.7814979936173,0.));
#13426=CARTESIAN_POINT('Ctrl Pts',(-19.6125074152527,4.7814979936173,21.));
#13427=CARTESIAN_POINT('Ctrl Pts',(-19.5720732205813,4.75328238194611,0.));
#13428=CARTESIAN_POINT('Ctrl Pts',(-19.5720732205813,4.75328238194611,21.));
#13429=CARTESIAN_POINT('Ctrl Pts',(-19.531511899192,4.72538815796615,0.));
#13430=CARTESIAN_POINT('Ctrl Pts',(-19.531511899192,4.72538815796615,21.));
#13431=CARTESIAN_POINT('Ctrl Pts',(-19.4908246636763,4.69781487613784,0.));
#13432=CARTESIAN_POINT('Ctrl Pts',(-19.4908246636763,4.69781487613784,21.));
#13433=CARTESIAN_POINT('Ctrl Pts',(-19.4500125912299,4.67056260851453,0.));
#13434=CARTESIAN_POINT('Ctrl Pts',(-19.4500125912299,4.67056260851453,21.));
#13435=CARTESIAN_POINT('Ctrl Pts',(-19.4090759683639,4.64363405547472,0.));
#13436=CARTESIAN_POINT('Ctrl Pts',(-19.4090759683639,4.64363405547472,21.));
#13437=CARTESIAN_POINT('Ctrl Pts',(-19.3680137353983,4.61703633725712,0.));
#13438=CARTESIAN_POINT('Ctrl Pts',(-19.3680137353983,4.61703633725712,21.));
#13439=CARTESIAN_POINT('Ctrl Pts',(-19.3268225655679,4.59078395765677,0.));
#13440=CARTESIAN_POINT('Ctrl Pts',(-19.3268225655679,4.59078395765677,21.));
#13441=CARTESIAN_POINT('Ctrl Pts',(-19.2854975819105,4.56489651606741,0.));
#13442=CARTESIAN_POINT('Ctrl Pts',(-19.2854975819105,4.56489651606741,21.));
#13443=CARTESIAN_POINT('Ctrl Pts',(-19.2440340196551,4.53939338835152,0.));
#13444=CARTESIAN_POINT('Ctrl Pts',(-19.2440340196551,4.53939338835152,21.));
#13445=CARTESIAN_POINT('Ctrl Pts',(-19.2024287376926,4.51428889122955,0.));
#13446=CARTESIAN_POINT('Ctrl Pts',(-19.2024287376926,4.51428889122955,21.));
#13447=CARTESIAN_POINT('Ctrl Pts',(-19.1606814968494,4.48958819710577,0.));
#13448=CARTESIAN_POINT('Ctrl Pts',(-19.1606814968494,4.48958819710577,21.));
#13449=CARTESIAN_POINT('Ctrl Pts',(-19.1187970904933,4.46528051067021,0.));
#13450=CARTESIAN_POINT('Ctrl Pts',(-19.1187970904933,4.46528051067021,21.));
#13451=CARTESIAN_POINT('Ctrl Pts',(-19.0767833717249,4.44134542994082,0.));
#13452=CARTESIAN_POINT('Ctrl Pts',(-19.0767833717249,4.44134542994082,21.));
#13453=CARTESIAN_POINT('Ctrl Pts',(-19.034647328575,4.41776558033332,0.));
#13454=CARTESIAN_POINT('Ctrl Pts',(-19.034647328575,4.41776558033332,21.));
#13455=CARTESIAN_POINT('Ctrl Pts',(-18.9923914823906,4.39453820875555,0.));
#13456=CARTESIAN_POINT('Ctrl Pts',(-18.9923914823906,4.39453820875555,21.));
#13457=CARTESIAN_POINT('Ctrl Pts',(-18.9500107909187,4.37168516143122,0.));
#13458=CARTESIAN_POINT('Ctrl Pts',(-18.9500107909187,4.37168516143122,21.));
#13459=CARTESIAN_POINT('Ctrl Pts',(-18.9074876952706,4.34926881342022,0.));
#13460=CARTESIAN_POINT('Ctrl Pts',(-18.9074876952706,4.34926881342022,21.));
#13461=CARTESIAN_POINT('Ctrl Pts',(-18.8647973781745,4.32737526247704,0.));
#13462=CARTESIAN_POINT('Ctrl Pts',(-18.8647973781745,4.32737526247704,21.));
#13463=CARTESIAN_POINT('Ctrl Pts',(-18.8219166495975,4.30608591031526,0.));
#13464=CARTESIAN_POINT('Ctrl Pts',(-18.8219166495975,4.30608591031526,21.));
#13465=CARTESIAN_POINT('Ctrl Pts',(-18.778832216358,4.28545098663153,0.));
#13466=CARTESIAN_POINT('Ctrl Pts',(-18.778832216358,4.28545098663153,21.));
#13467=CARTESIAN_POINT('Ctrl Pts',(-18.735547949685,4.26546636161933,0.));
#13468=CARTESIAN_POINT('Ctrl Pts',(-18.735547949685,4.26546636161933,21.));
#13469=CARTESIAN_POINT('Ctrl Pts',(-18.6920958920047,4.24603817988452,0.));
#13470=CARTESIAN_POINT('Ctrl Pts',(-18.6920958920047,4.24603817988452,21.));
#13471=CARTESIAN_POINT('Ctrl Pts',(-18.6485210883348,4.22703266508919,0.));
#13472=CARTESIAN_POINT('Ctrl Pts',(-18.6485210883348,4.22703266508919,21.));
#13473=CARTESIAN_POINT('Ctrl Pts',(-18.6048602364653,4.20834600700665,0.));
#13474=CARTESIAN_POINT('Ctrl Pts',(-18.6048602364653,4.20834600700665,21.));
#13475=CARTESIAN_POINT('Ctrl Pts',(-18.5611217636409,4.18996967278621,0.));
#13476=CARTESIAN_POINT('Ctrl Pts',(-18.5611217636409,4.18996967278621,21.));
#13477=CARTESIAN_POINT('Ctrl Pts',(-18.5172668097744,4.17205262766562,0.));
#13478=CARTESIAN_POINT('Ctrl Pts',(-18.5172668097744,4.17205262766562,21.));
#13479=CARTESIAN_POINT('Ctrl Pts',(-18.4731856794913,4.15497867673974,0.));
#13480=CARTESIAN_POINT('Ctrl Pts',(-18.4731856794913,4.15497867673974,21.));
#13481=CARTESIAN_POINT('Ctrl Pts',(-18.4287286547442,4.13926275457062,0.));
#13482=CARTESIAN_POINT('Ctrl Pts',(-18.4287286547442,4.13926275457062,21.));
#13483=CARTESIAN_POINT('Ctrl Pts',(-18.3927403741815,4.12819301671079,0.));
#13484=CARTESIAN_POINT('Ctrl Pts',(-18.3927403741815,4.12819301671079,21.));
#13485=CARTESIAN_POINT('Ctrl Pts',(-18.3654573320481,4.1209201986886,0.));
#13486=CARTESIAN_POINT('Ctrl Pts',(-18.3654573320481,4.1209201986886,21.));
#13487=CARTESIAN_POINT('Ctrl Pts',(-18.3471320125699,4.11655269114951,0.));
#13488=CARTESIAN_POINT('Ctrl Pts',(-18.3471320125699,4.11655269114951,21.));
#13489=CARTESIAN_POINT('Ctrl Pts',(-18.337935196262,4.11448919812531,0.));
#13490=CARTESIAN_POINT('Ctrl Pts',(-18.337935196262,4.11448919812531,21.));
#13491=CARTESIAN_POINT('',(-21.1275013067528,6.13422273260085,0.));
#13492=CARTESIAN_POINT('Ctrl Pts',(-18.337935196262,4.11448919812531,0.));
#13493=CARTESIAN_POINT('Ctrl Pts',(-18.3471320125699,4.11655269114951,0.));
#13494=CARTESIAN_POINT('Ctrl Pts',(-18.3654573320481,4.1209201986886,0.));
#13495=CARTESIAN_POINT('Ctrl Pts',(-18.3927403741815,4.12819301671079,0.));
#13496=CARTESIAN_POINT('Ctrl Pts',(-18.4287286547442,4.13926275457062,0.));
#13497=CARTESIAN_POINT('Ctrl Pts',(-18.4731856794913,4.15497867673974,0.));
#13498=CARTESIAN_POINT('Ctrl Pts',(-18.5172668097744,4.17205262766562,0.));
#13499=CARTESIAN_POINT('Ctrl Pts',(-18.5611217636409,4.18996967278621,0.));
#13500=CARTESIAN_POINT('Ctrl Pts',(-18.6048602364653,4.20834600700665,0.));
#13501=CARTESIAN_POINT('Ctrl Pts',(-18.6485210883348,4.22703266508919,0.));
#13502=CARTESIAN_POINT('Ctrl Pts',(-18.6920958920047,4.24603817988452,0.));
#13503=CARTESIAN_POINT('Ctrl Pts',(-18.735547949685,4.26546636161933,0.));
#13504=CARTESIAN_POINT('Ctrl Pts',(-18.778832216358,4.28545098663153,0.));
#13505=CARTESIAN_POINT('Ctrl Pts',(-18.8219166495975,4.30608591031526,0.));
#13506=CARTESIAN_POINT('Ctrl Pts',(-18.8647973781745,4.32737526247704,0.));
#13507=CARTESIAN_POINT('Ctrl Pts',(-18.9074876952706,4.34926881342022,0.));
#13508=CARTESIAN_POINT('Ctrl Pts',(-18.9500107909187,4.37168516143122,0.));
#13509=CARTESIAN_POINT('Ctrl Pts',(-18.9923914823906,4.39453820875555,0.));
#13510=CARTESIAN_POINT('Ctrl Pts',(-19.034647328575,4.41776558033332,0.));
#13511=CARTESIAN_POINT('Ctrl Pts',(-19.0767833717249,4.44134542994082,0.));
#13512=CARTESIAN_POINT('Ctrl Pts',(-19.1187970904933,4.46528051067021,0.));
#13513=CARTESIAN_POINT('Ctrl Pts',(-19.1606814968494,4.48958819710577,0.));
#13514=CARTESIAN_POINT('Ctrl Pts',(-19.2024287376926,4.51428889122955,0.));
#13515=CARTESIAN_POINT('Ctrl Pts',(-19.2440340196551,4.53939338835152,0.));
#13516=CARTESIAN_POINT('Ctrl Pts',(-19.2854975819105,4.56489651606741,0.));
#13517=CARTESIAN_POINT('Ctrl Pts',(-19.3268225655679,4.59078395765677,0.));
#13518=CARTESIAN_POINT('Ctrl Pts',(-19.3680137353983,4.61703633725712,0.));
#13519=CARTESIAN_POINT('Ctrl Pts',(-19.4090759683639,4.64363405547472,0.));
#13520=CARTESIAN_POINT('Ctrl Pts',(-19.4500125912299,4.67056260851453,0.));
#13521=CARTESIAN_POINT('Ctrl Pts',(-19.4908246636763,4.69781487613784,0.));
#13522=CARTESIAN_POINT('Ctrl Pts',(-19.531511899192,4.72538815796615,0.));
#13523=CARTESIAN_POINT('Ctrl Pts',(-19.5720732205813,4.75328238194611,0.));
#13524=CARTESIAN_POINT('Ctrl Pts',(-19.6125074152527,4.7814979936173,0.));
#13525=CARTESIAN_POINT('Ctrl Pts',(-19.6528138625329,4.81003361418061,0.));
#13526=CARTESIAN_POINT('Ctrl Pts',(-19.6929928227072,4.83888510708974,0.));
#13527=CARTESIAN_POINT('Ctrl Pts',(-19.7330450480715,4.86804682289087,0.));
#13528=CARTESIAN_POINT('Ctrl Pts',(-19.772971552601,4.89751233527804,0.));
#13529=CARTESIAN_POINT('Ctrl Pts',(-19.8127733387903,4.92727531494347,0.));
#13530=CARTESIAN_POINT('Ctrl Pts',(-19.8524510953961,4.95733049830096,0.));
#13531=CARTESIAN_POINT('Ctrl Pts',(-19.8920050831202,4.98767405031333,0.));
#13532=CARTESIAN_POINT('Ctrl Pts',(-19.931435301086,5.01830302225557,0.));
#13533=CARTESIAN_POINT('Ctrl Pts',(-19.9707415879783,5.04921502064063,0.));
#13534=CARTESIAN_POINT('Ctrl Pts',(-20.0099237417205,5.08040781745336,0.));
#13535=CARTESIAN_POINT('Ctrl Pts',(-20.0489816528155,5.11187891582335,0.));
#13536=CARTESIAN_POINT('Ctrl Pts',(-20.087915358486,5.14362537555398,0.));
#13537=CARTESIAN_POINT('Ctrl Pts',(-20.1267249732337,5.17564404279922,0.));
#13538=CARTESIAN_POINT('Ctrl Pts',(-20.1654106491899,5.20793168386163,0.));
#13539=CARTESIAN_POINT('Ctrl Pts',(-20.2039725283917,5.2404851444189,0.));
#13540=CARTESIAN_POINT('Ctrl Pts',(-20.2424106921768,5.2733015229815,0.));
#13541=CARTESIAN_POINT('Ctrl Pts',(-20.2807251380077,5.30637824220997,0.));
#13542=CARTESIAN_POINT('Ctrl Pts',(-20.3189158047642,5.33971294212214,0.));
#13543=CARTESIAN_POINT('Ctrl Pts',(-20.3569825877537,5.37330341114649,0.));
#13544=CARTESIAN_POINT('Ctrl Pts',(-20.3949253578015,5.40714750595875,0.));
#13545=CARTESIAN_POINT('Ctrl Pts',(-20.4327439816542,5.44124306065111,0.));
#13546=CARTESIAN_POINT('Ctrl Pts',(-20.4704383353718,5.47558784449851,0.));
#13547=CARTESIAN_POINT('Ctrl Pts',(-20.5080083009242,5.51017962306782,0.));
#13548=CARTESIAN_POINT('Ctrl Pts',(-20.5454537676144,5.5450161968946,0.));
#13549=CARTESIAN_POINT('Ctrl Pts',(-20.5827746317185,5.58009544402475,0.));
#13550=CARTESIAN_POINT('Ctrl Pts',(-20.6199707996366,5.61541536715149,0.));
#13551=CARTESIAN_POINT('Ctrl Pts',(-20.6570421847033,5.65097411164335,0.));
#13552=CARTESIAN_POINT('Ctrl Pts',(-20.6939886877061,5.68676990500163,0.));
#13553=CARTESIAN_POINT('Ctrl Pts',(-20.7308101804425,5.72280100798241,0.));
#13554=CARTESIAN_POINT('Ctrl Pts',(-20.7675064905026,5.75906566327796,0.));
#13555=CARTESIAN_POINT('Ctrl Pts',(-20.8040773827343,5.79556203439644,0.));
#13556=CARTESIAN_POINT('Ctrl Pts',(-20.8405225541277,5.83228817460178,0.));
#13557=CARTESIAN_POINT('Ctrl Pts',(-20.8768416821402,5.86924212736288,0.));
#13558=CARTESIAN_POINT('Ctrl Pts',(-20.9130344665641,5.906422006626,0.));
#13559=CARTESIAN_POINT('Ctrl Pts',(-20.9491006734021,5.94382608200804,0.));
#13560=CARTESIAN_POINT('Ctrl Pts',(-20.9850401822713,5.98145286361837,0.));
#13561=CARTESIAN_POINT('Ctrl Pts',(-21.0280155918661,6.02687083887287,0.));
#13562=CARTESIAN_POINT('Ctrl Pts',(-21.0636702474951,6.06499496148845,0.));
#13563=CARTESIAN_POINT('Ctrl Pts',(-21.0920928984154,6.09567013127871,0.));
#13564=CARTESIAN_POINT('Ctrl Pts',(-21.1133530893457,6.11877533761502,0.));
#13565=CARTESIAN_POINT('Ctrl Pts',(-21.1275013067528,6.1342227326009,0.));
#13566=CARTESIAN_POINT('',(-21.1275013067528,6.13422273260085,13.));
#13567=CARTESIAN_POINT('Ctrl Pts',(-21.1275013067528,6.1342227326009,13.));
#13568=CARTESIAN_POINT('Ctrl Pts',(-21.0578559230999,6.05818207543008,13.));
#13569=CARTESIAN_POINT('Ctrl Pts',(-20.9874765053145,5.98341417321284,13.));
#13570=CARTESIAN_POINT('Ctrl Pts',(-20.9163599174182,5.90994468906837,13.));
#13571=CARTESIAN_POINT('Ctrl Pts',(-20.7985166493983,5.78820257000103,13.));
#13572=CARTESIAN_POINT('Ctrl Pts',(-20.6786545111106,5.6700381210249,13.));
#13573=CARTESIAN_POINT('Ctrl Pts',(-20.5568063022896,5.55573864053401,13.));
#13574=CARTESIAN_POINT('Ctrl Pts',(-20.4631466243016,5.46788135776747,13.));
#13575=CARTESIAN_POINT('Ctrl Pts',(-20.3683108787545,5.38230707413678,13.));
#13576=CARTESIAN_POINT('Ctrl Pts',(-20.2723075600433,5.29917141679073,13.));
#13577=CARTESIAN_POINT('Ctrl Pts',(-20.1689623028903,5.20967788675077,13.));
#13578=CARTESIAN_POINT('Ctrl Pts',(-20.0642651129984,5.12300396079329,13.));
#13579=CARTESIAN_POINT('Ctrl Pts',(-19.9582092070171,5.03941267576854,13.));
#13580=CARTESIAN_POINT('Ctrl Pts',(-19.8994937738184,4.99313426754168,13.));
#13581=CARTESIAN_POINT('Ctrl Pts',(-19.8403635608621,4.94779583996753,13.));
#13582=CARTESIAN_POINT('Ctrl Pts',(-19.7808173213525,4.90344584505529,13.));
#13583=CARTESIAN_POINT('Ctrl Pts',(-19.7234362340388,4.86070845388874,13.));
#13584=CARTESIAN_POINT('Ctrl Pts',(-19.665666793332,4.8188953867059,13.));
#13585=CARTESIAN_POINT('Ctrl Pts',(-19.6074986353569,4.77808296524689,13.));
#13586=CARTESIAN_POINT('Ctrl Pts',(-19.5572235046905,4.74280851453208,13.));
#13587=CARTESIAN_POINT('Ctrl Pts',(-19.5066514987622,4.70827845283243,13.));
#13588=CARTESIAN_POINT('Ctrl Pts',(-19.4557905169783,4.67449772127139,13.));
#13589=CARTESIAN_POINT('Ctrl Pts',(-19.4192898917399,4.65025481876063,13.));
#13590=CARTESIAN_POINT('Ctrl Pts',(-19.382641288418,4.62639514817842,13.));
#13591=CARTESIAN_POINT('Ctrl Pts',(-19.3458364380218,4.60295743043302,13.));
#13592=CARTESIAN_POINT('Ctrl Pts',(-19.3096309080951,4.57990136629721,13.));
#13593=CARTESIAN_POINT('Ctrl Pts',(-19.2732722733459,4.55725971973435,13.));
#13594=CARTESIAN_POINT('Ctrl Pts',(-19.2367485574674,4.53508357551694,13.));
#13595=CARTESIAN_POINT('Ctrl Pts',(-19.205080350215,4.51585555574276,13.));
#13596=CARTESIAN_POINT('Ctrl Pts',(-19.1732873011956,4.49697986249447,13.));
#13597=CARTESIAN_POINT('Ctrl Pts',(-19.1413765620497,4.47844262259009,13.));
#13598=CARTESIAN_POINT('Ctrl Pts',(-19.1124727543428,4.4616521366297,13.));
#13599=CARTESIAN_POINT('Ctrl Pts',(-19.083474045539,4.44513401120468,13.));
#13600=CARTESIAN_POINT('Ctrl Pts',(-19.0543895551234,4.42886646462772,13.));
#13601=CARTESIAN_POINT('Ctrl Pts',(-19.0298903165561,4.41516354259612,13.));
#13602=CARTESIAN_POINT('Ctrl Pts',(-19.0053307305268,4.40163676081042,13.));
#13603=CARTESIAN_POINT('Ctrl Pts',(-18.9807063063319,4.38830551702962,13.));
#13604=CARTESIAN_POINT('Ctrl Pts',(-18.9450720846902,4.36901375646356,13.));
#13605=CARTESIAN_POINT('Ctrl Pts',(-18.9093017976668,4.35013223004763,13.));
#13606=CARTESIAN_POINT('Ctrl Pts',(-18.8733353265524,4.33187128675496,13.));
#13607=CARTESIAN_POINT('Ctrl Pts',(-18.8516029898089,4.32083731659903,13.));
#13608=CARTESIAN_POINT('Ctrl Pts',(-18.8297980042953,4.31003325590031,13.));
#13609=CARTESIAN_POINT('Ctrl Pts',(-18.8079138030273,4.29948469308613,13.));
#13610=CARTESIAN_POINT('Ctrl Pts',(-18.7877304129875,4.28975595064628,13.));
#13611=CARTESIAN_POINT('Ctrl Pts',(-18.7674792482884,4.28024580006689,13.));
#13612=CARTESIAN_POINT('Ctrl Pts',(-18.7471689058935,4.27093067982675,13.));
#13613=CARTESIAN_POINT('Ctrl Pts',(-18.7192299720641,4.25811678811867,13.));
#13614=CARTESIAN_POINT('Ctrl Pts',(-18.6911811213665,4.24566493398838,13.));
#13615=CARTESIAN_POINT('Ctrl Pts',(-18.663071173524,4.23343245340777,13.));
#13616=CARTESIAN_POINT('Ctrl Pts',(-18.6452377209097,4.2256719494036,13.));
#13617=CARTESIAN_POINT('Ctrl Pts',(-18.6273802007938,4.21799814919381,13.));
#13618=CARTESIAN_POINT('Ctrl Pts',(-18.6095026819025,4.21040342106478,13.));
#13619=CARTESIAN_POINT('Ctrl Pts',(-18.5934584408283,4.20358750607481,13.));
#13620=CARTESIAN_POINT('Ctrl Pts',(-18.5773983084498,4.1968345819597,13.));
#13621=CARTESIAN_POINT('Ctrl Pts',(-18.5613135377966,4.19017810366012,13.));
#13622=CARTESIAN_POINT('Ctrl Pts',(-18.5444052403814,4.18318081925649,13.));
#13623=CARTESIAN_POINT('Ctrl Pts',(-18.5274697699072,4.17628995974216,13.));
#13624=CARTESIAN_POINT('Ctrl Pts',(-18.5104789585051,4.16960404100154,13.));
#13625=CARTESIAN_POINT('Ctrl Pts',(-18.482257258292,4.1584987447398,13.));
#13626=CARTESIAN_POINT('Ctrl Pts',(-18.4538805849791,4.14796697293776,13.));
#13627=CARTESIAN_POINT('Ctrl Pts',(-18.4251735639783,4.13860964459712,13.));
#13628=CARTESIAN_POINT('Ctrl Pts',(-18.4093434909438,4.13344968073196,13.));
#13629=CARTESIAN_POINT('Ctrl Pts',(-18.3934125378492,4.1286481456075,13.));
#13630=CARTESIAN_POINT('Ctrl Pts',(-18.377359006511,4.12427889810063,13.));
#13631=CARTESIAN_POINT('Ctrl Pts',(-18.3643002867397,4.12072474060085,13.));
#13632=CARTESIAN_POINT('Ctrl Pts',(-18.3511604736674,4.117456558433,13.));
#13633=CARTESIAN_POINT('Ctrl Pts',(-18.337935196262,4.11448919812531,13.));
#13634=CARTESIAN_POINT('',(-21.1275013067528,6.13422273260085,0.));
#13635=CARTESIAN_POINT('Origin',(-5.38923623413286E-12,1.75106900012182E-12,
0.));
#13636=CARTESIAN_POINT('',(-20.698113262342,7.45574324794401,0.));
#13637=CARTESIAN_POINT('Origin',(-5.38923623413286E-12,1.75106900012182E-12,
0.));
#13638=CARTESIAN_POINT('',(-20.698113262342,7.45574324794401,13.));
#13639=CARTESIAN_POINT('Origin',(-5.38923623413286E-12,1.75106900012182E-12,
13.));
#13640=CARTESIAN_POINT('',(-20.698113262342,7.45574324794401,0.));
#13641=CARTESIAN_POINT('Ctrl Pts',(-17.2541372868972,7.45007618140238,0.));
#13642=CARTESIAN_POINT('Ctrl Pts',(-17.2541372868972,7.45007618140238,21.));
#13643=CARTESIAN_POINT('Ctrl Pts',(-17.2627905583523,7.45381253347183,0.));
#13644=CARTESIAN_POINT('Ctrl Pts',(-17.2627905583523,7.45381253347183,21.));
#13645=CARTESIAN_POINT('Ctrl Pts',(-17.2801832097582,7.46105049818251,0.));
#13646=CARTESIAN_POINT('Ctrl Pts',(-17.2801832097582,7.46105049818251,21.));
#13647=CARTESIAN_POINT('Ctrl Pts',(-17.3065305096784,7.4712032346092,0.));
#13648=CARTESIAN_POINT('Ctrl Pts',(-17.3065305096784,7.4712032346092,21.));
#13649=CARTESIAN_POINT('Ctrl Pts',(-17.3421522689127,7.48340100912745,0.));
#13650=CARTESIAN_POINT('Ctrl Pts',(-17.3421522689127,7.48340100912745,21.));
#13651=CARTESIAN_POINT('Ctrl Pts',(-17.3873563447297,7.49681774451751,0.));
#13652=CARTESIAN_POINT('Ctrl Pts',(-17.3873563447297,7.49681774451751,21.));
#13653=CARTESIAN_POINT('Ctrl Pts',(-17.4330545448126,7.50891486634214,0.));
#13654=CARTESIAN_POINT('Ctrl Pts',(-17.4330545448126,7.50891486634214,21.));
#13655=CARTESIAN_POINT('Ctrl Pts',(-17.4790653226646,7.52019696747328,0.));
#13656=CARTESIAN_POINT('Ctrl Pts',(-17.4790653226646,7.52019696747328,21.));
#13657=CARTESIAN_POINT('Ctrl Pts',(-17.5252518287336,7.53103903007863,0.));
#13658=CARTESIAN_POINT('Ctrl Pts',(-17.5252518287336,7.53103903007863,21.));
#13659=CARTESIAN_POINT('Ctrl Pts',(-17.5715579419204,7.54158441095317,0.));
#13660=CARTESIAN_POINT('Ctrl Pts',(-17.5715579419204,7.54158441095317,21.));
#13661=CARTESIAN_POINT('Ctrl Pts',(-17.6179818599248,7.55182125346564,0.));
#13662=CARTESIAN_POINT('Ctrl Pts',(-17.6179818599248,7.55182125346564,21.));
#13663=CARTESIAN_POINT('Ctrl Pts',(-17.6645549117314,7.56164400295863,0.));
#13664=CARTESIAN_POINT('Ctrl Pts',(-17.6645549117314,7.56164400295863,21.));
#13665=CARTESIAN_POINT('Ctrl Pts',(-17.7113192869136,7.57091795530423,0.));
#13666=CARTESIAN_POINT('Ctrl Pts',(-17.7113192869136,7.57091795530423,21.));
#13667=CARTESIAN_POINT('Ctrl Pts',(-17.7583042294209,7.57954834582803,0.));
#13668=CARTESIAN_POINT('Ctrl Pts',(-17.7583042294209,7.57954834582803,21.));
#13669=CARTESIAN_POINT('Ctrl Pts',(-17.8055090348024,7.58752955799499,0.));
#13670=CARTESIAN_POINT('Ctrl Pts',(-17.8055090348024,7.58752955799499,21.));
#13671=CARTESIAN_POINT('Ctrl Pts',(-17.8529149331931,7.59491004201955,0.));
#13672=CARTESIAN_POINT('Ctrl Pts',(-17.8529149331931,7.59491004201955,21.));
#13673=CARTESIAN_POINT('Ctrl Pts',(-17.900492838997,7.60176928403058,0.));
#13674=CARTESIAN_POINT('Ctrl Pts',(-17.900492838997,7.60176928403058,21.));
#13675=CARTESIAN_POINT('Ctrl Pts',(-17.9482122228183,7.60819152580111,0.));
#13676=CARTESIAN_POINT('Ctrl Pts',(-17.9482122228183,7.60819152580111,21.));
#13677=CARTESIAN_POINT('Ctrl Pts',(-17.9960506269561,7.61423755067038,0.));
#13678=CARTESIAN_POINT('Ctrl Pts',(-17.9960506269561,7.61423755067038,21.));
#13679=CARTESIAN_POINT('Ctrl Pts',(-18.0439992897906,7.61992799636654,0.));
#13680=CARTESIAN_POINT('Ctrl Pts',(-18.0439992897906,7.61992799636654,21.));
#13681=CARTESIAN_POINT('Ctrl Pts',(-18.0920577897363,7.62525915358074,0.));
#13682=CARTESIAN_POINT('Ctrl Pts',(-18.0920577897363,7.62525915358074,21.));
#13683=CARTESIAN_POINT('Ctrl Pts',(-18.1402306858819,7.63021285851761,0.));
#13684=CARTESIAN_POINT('Ctrl Pts',(-18.1402306858819,7.63021285851761,21.));
#13685=CARTESIAN_POINT('Ctrl Pts',(-18.1885236169197,7.63476798969016,0.));
#13686=CARTESIAN_POINT('Ctrl Pts',(-18.1885236169197,7.63476798969016,21.));
#13687=CARTESIAN_POINT('Ctrl Pts',(-18.2369390502576,7.63891299603826,0.));
#13688=CARTESIAN_POINT('Ctrl Pts',(-18.2369390502576,7.63891299603826,21.));
#13689=CARTESIAN_POINT('Ctrl Pts',(-18.2854741391282,7.6426522027076,0.));
#13690=CARTESIAN_POINT('Ctrl Pts',(-18.2854741391282,7.6426522027076,21.));
#13691=CARTESIAN_POINT('Ctrl Pts',(-18.3341230095852,7.64599903846601,0.));
#13692=CARTESIAN_POINT('Ctrl Pts',(-18.3341230095852,7.64599903846601,21.));
#13693=CARTESIAN_POINT('Ctrl Pts',(-18.3828781275628,7.6489719793775,0.));
#13694=CARTESIAN_POINT('Ctrl Pts',(-18.3828781275628,7.6489719793775,21.));
#13695=CARTESIAN_POINT('Ctrl Pts',(-18.4317319183719,7.65158974829126,0.));
#13696=CARTESIAN_POINT('Ctrl Pts',(-18.4317319183719,7.65158974829126,21.));
#13697=CARTESIAN_POINT('Ctrl Pts',(-18.4806785483052,7.65386603444743,0.));
#13698=CARTESIAN_POINT('Ctrl Pts',(-18.4806785483052,7.65386603444743,21.));
#13699=CARTESIAN_POINT('Ctrl Pts',(-18.5297146894905,7.65580722110437,0.));
#13700=CARTESIAN_POINT('Ctrl Pts',(-18.5297146894905,7.65580722110437,21.));
#13701=CARTESIAN_POINT('Ctrl Pts',(-18.5788385228928,7.65741532450727,0.));
#13702=CARTESIAN_POINT('Ctrl Pts',(-18.5788385228928,7.65741532450727,21.));
#13703=CARTESIAN_POINT('Ctrl Pts',(-18.6280491346907,7.65868976978872,0.));
#13704=CARTESIAN_POINT('Ctrl Pts',(-18.6280491346907,7.65868976978872,21.));
#13705=CARTESIAN_POINT('Ctrl Pts',(-18.6773458057584,7.65962948375621,0.));
#13706=CARTESIAN_POINT('Ctrl Pts',(-18.6773458057584,7.65962948375621,21.));
#13707=CARTESIAN_POINT('Ctrl Pts',(-18.7267272235231,7.66023521705905,0.));
#13708=CARTESIAN_POINT('Ctrl Pts',(-18.7267272235231,7.66023521705905,21.));
#13709=CARTESIAN_POINT('Ctrl Pts',(-18.7761911671591,7.6605104692254,0.));
#13710=CARTESIAN_POINT('Ctrl Pts',(-18.7761911671591,7.6605104692254,21.));
#13711=CARTESIAN_POINT('Ctrl Pts',(-18.8257349246207,7.66046025294775,0.));
#13712=CARTESIAN_POINT('Ctrl Pts',(-18.8257349246207,7.66046025294775,21.));
#13713=CARTESIAN_POINT('Ctrl Pts',(-18.8753555389435,7.66009036321663,0.));
#13714=CARTESIAN_POINT('Ctrl Pts',(-18.8753555389435,7.66009036321663,21.));
#13715=CARTESIAN_POINT('Ctrl Pts',(-18.9250501008887,7.65940650980099,0.));
#13716=CARTESIAN_POINT('Ctrl Pts',(-18.9250501008887,7.65940650980099,21.));
#13717=CARTESIAN_POINT('Ctrl Pts',(-18.974816073814,7.65841335587266,0.));
#13718=CARTESIAN_POINT('Ctrl Pts',(-18.974816073814,7.65841335587266,21.));
#13719=CARTESIAN_POINT('Ctrl Pts',(-19.0246514144531,7.65711415727855,0.));
#13720=CARTESIAN_POINT('Ctrl Pts',(-19.0246514144531,7.65711415727855,21.));
#13721=CARTESIAN_POINT('Ctrl Pts',(-19.0745543888799,7.65551129907201,0.));
#13722=CARTESIAN_POINT('Ctrl Pts',(-19.0745543888799,7.65551129907201,21.));
#13723=CARTESIAN_POINT('Ctrl Pts',(-19.1245234597312,7.65360662280609,0.));
#13724=CARTESIAN_POINT('Ctrl Pts',(-19.1245234597312,7.65360662280609,21.));
#13725=CARTESIAN_POINT('Ctrl Pts',(-19.1745571539291,7.65140181220526,0.));
#13726=CARTESIAN_POINT('Ctrl Pts',(-19.1745571539291,7.65140181220526,21.));
#13727=CARTESIAN_POINT('Ctrl Pts',(-19.224653915265,7.64889882291923,0.));
#13728=CARTESIAN_POINT('Ctrl Pts',(-19.224653915265,7.64889882291923,21.));
#13729=CARTESIAN_POINT('Ctrl Pts',(-19.2748120456486,7.64610005549613,0.));
#13730=CARTESIAN_POINT('Ctrl Pts',(-19.2748120456486,7.64610005549613,21.));
#13731=CARTESIAN_POINT('Ctrl Pts',(-19.3250297839295,7.64300812875339,0.));
#13732=CARTESIAN_POINT('Ctrl Pts',(-19.3250297839295,7.64300812875339,21.));
#13733=CARTESIAN_POINT('Ctrl Pts',(-19.3753053524647,7.63962574822761,0.));
#13734=CARTESIAN_POINT('Ctrl Pts',(-19.3753053524647,7.63962574822761,21.));
#13735=CARTESIAN_POINT('Ctrl Pts',(-19.4256370121006,7.63595554930654,0.));
#13736=CARTESIAN_POINT('Ctrl Pts',(-19.4256370121006,7.63595554930654,21.));
#13737=CARTESIAN_POINT('Ctrl Pts',(-19.4760231231881,7.63199992715366,0.));
#13738=CARTESIAN_POINT('Ctrl Pts',(-19.4760231231881,7.63199992715366,21.));
#13739=CARTESIAN_POINT('Ctrl Pts',(-19.5264621687521,7.62776096538883,0.));
#13740=CARTESIAN_POINT('Ctrl Pts',(-19.5264621687521,7.62776096538883,21.));
#13741=CARTESIAN_POINT('Ctrl Pts',(-19.5769527121826,7.62324053735219,0.));
#13742=CARTESIAN_POINT('Ctrl Pts',(-19.5769527121826,7.62324053735219,21.));
#13743=CARTESIAN_POINT('Ctrl Pts',(-19.6274933688524,7.61844037070591,0.));
#13744=CARTESIAN_POINT('Ctrl Pts',(-19.6274933688524,7.61844037070591,21.));
#13745=CARTESIAN_POINT('Ctrl Pts',(-19.6780827744426,7.61336212350879,0.));
#13746=CARTESIAN_POINT('Ctrl Pts',(-19.6780827744426,7.61336212350879,21.));
#13747=CARTESIAN_POINT('Ctrl Pts',(-19.7287195480601,7.60800746969262,0.));
#13748=CARTESIAN_POINT('Ctrl Pts',(-19.7287195480601,7.60800746969262,21.));
#13749=CARTESIAN_POINT('Ctrl Pts',(-19.7794022782484,7.60237814110187,0.));
#13750=CARTESIAN_POINT('Ctrl Pts',(-19.7794022782484,7.60237814110187,21.));
#13751=CARTESIAN_POINT('Ctrl Pts',(-19.830129556152,7.59647587605448,0.));
#13752=CARTESIAN_POINT('Ctrl Pts',(-19.830129556152,7.59647587605448,21.));
#13753=CARTESIAN_POINT('Ctrl Pts',(-19.8808999994024,7.59030238888852,0.));
#13754=CARTESIAN_POINT('Ctrl Pts',(-19.8808999994024,7.59030238888852,21.));
#13755=CARTESIAN_POINT('Ctrl Pts',(-19.931712276832,7.58385933533352,0.));
#13756=CARTESIAN_POINT('Ctrl Pts',(-19.931712276832,7.58385933533352,21.));
#13757=CARTESIAN_POINT('Ctrl Pts',(-19.9825651387294,7.57714827622806,0.));
#13758=CARTESIAN_POINT('Ctrl Pts',(-19.9825651387294,7.57714827622806,21.));
#13759=CARTESIAN_POINT('Ctrl Pts',(-20.0334574248556,7.57017066105973,0.));
#13760=CARTESIAN_POINT('Ctrl Pts',(-20.0334574248556,7.57017066105973,21.));
#13761=CARTESIAN_POINT('Ctrl Pts',(-20.0843880130978,7.5629278654946,0.));
#13762=CARTESIAN_POINT('Ctrl Pts',(-20.0843880130978,7.5629278654946,21.));
#13763=CARTESIAN_POINT('Ctrl Pts',(-20.1353557774357,7.55542122125494,0.));
#13764=CARTESIAN_POINT('Ctrl Pts',(-20.1353557774357,7.55542122125494,21.));
#13765=CARTESIAN_POINT('Ctrl Pts',(-20.1863595454674,7.54765204869254,0.));
#13766=CARTESIAN_POINT('Ctrl Pts',(-20.1863595454674,7.54765204869254,21.));
#13767=CARTESIAN_POINT('Ctrl Pts',(-20.2373980474879,7.53962169534167,0.));
#13768=CARTESIAN_POINT('Ctrl Pts',(-20.2373980474879,7.53962169534167,21.));
#13769=CARTESIAN_POINT('Ctrl Pts',(-20.2884698940944,7.53133155804008,0.));
#13770=CARTESIAN_POINT('Ctrl Pts',(-20.2884698940944,7.53133155804008,21.));
#13771=CARTESIAN_POINT('Ctrl Pts',(-20.3395736743243,7.52278303006887,0.));
#13772=CARTESIAN_POINT('Ctrl Pts',(-20.3395736743243,7.52278303006887,21.));
#13773=CARTESIAN_POINT('Ctrl Pts',(-20.3907080367098,7.51397746081994,0.));
#13774=CARTESIAN_POINT('Ctrl Pts',(-20.3907080367098,7.51397746081994,21.));
#13775=CARTESIAN_POINT('Ctrl Pts',(-20.4418717748497,7.50491611266253,0.));
#13776=CARTESIAN_POINT('Ctrl Pts',(-20.4418717748497,7.50491611266253,21.));
#13777=CARTESIAN_POINT('Ctrl Pts',(-20.4930639156161,7.49560012018405,0.));
#13778=CARTESIAN_POINT('Ctrl Pts',(-20.4930639156161,7.49560012018405,21.));
#13779=CARTESIAN_POINT('Ctrl Pts',(-20.5442837929044,7.48603045196745,0.));
#13780=CARTESIAN_POINT('Ctrl Pts',(-20.5442837929044,7.48603045196745,21.));
#13781=CARTESIAN_POINT('Ctrl Pts',(-20.5955309838521,7.47620789245428,0.));
#13782=CARTESIAN_POINT('Ctrl Pts',(-20.5955309838521,7.47620789245428,21.));
#13783=CARTESIAN_POINT('Ctrl Pts',(-20.6365504027501,7.46814799701905,0.));
#13784=CARTESIAN_POINT('Ctrl Pts',(-20.6365504027501,7.46814799701905,21.));
#13785=CARTESIAN_POINT('Ctrl Pts',(-20.6673271112931,7.46198969876654,0.));
#13786=CARTESIAN_POINT('Ctrl Pts',(-20.6673271112931,7.46198969876654,21.));
#13787=CARTESIAN_POINT('Ctrl Pts',(-20.6878503127065,7.45783379370107,0.));
#13788=CARTESIAN_POINT('Ctrl Pts',(-20.6878503127065,7.45783379370107,21.));
#13789=CARTESIAN_POINT('Ctrl Pts',(-20.698113262342,7.45574324794401,0.));
#13790=CARTESIAN_POINT('Ctrl Pts',(-20.698113262342,7.45574324794401,21.));
#13791=CARTESIAN_POINT('Ctrl Pts',(-17.2541372868972,7.45007618140238,0.));
#13792=CARTESIAN_POINT('Ctrl Pts',(-17.2627905583523,7.45381253347183,0.));
#13793=CARTESIAN_POINT('Ctrl Pts',(-17.2801832097582,7.46105049818251,0.));
#13794=CARTESIAN_POINT('Ctrl Pts',(-17.3065305096784,7.4712032346092,0.));
#13795=CARTESIAN_POINT('Ctrl Pts',(-17.3421522689127,7.48340100912745,0.));
#13796=CARTESIAN_POINT('Ctrl Pts',(-17.3873563447297,7.49681774451751,0.));
#13797=CARTESIAN_POINT('Ctrl Pts',(-17.4330545448126,7.50891486634214,0.));
#13798=CARTESIAN_POINT('Ctrl Pts',(-17.4790653226646,7.52019696747328,0.));
#13799=CARTESIAN_POINT('Ctrl Pts',(-17.5252518287336,7.53103903007863,0.));
#13800=CARTESIAN_POINT('Ctrl Pts',(-17.5715579419204,7.54158441095317,0.));
#13801=CARTESIAN_POINT('Ctrl Pts',(-17.6179818599248,7.55182125346564,0.));
#13802=CARTESIAN_POINT('Ctrl Pts',(-17.6645549117314,7.56164400295863,0.));
#13803=CARTESIAN_POINT('Ctrl Pts',(-17.7113192869136,7.57091795530423,0.));
#13804=CARTESIAN_POINT('Ctrl Pts',(-17.7583042294209,7.57954834582803,0.));
#13805=CARTESIAN_POINT('Ctrl Pts',(-17.8055090348024,7.58752955799499,0.));
#13806=CARTESIAN_POINT('Ctrl Pts',(-17.8529149331931,7.59491004201955,0.));
#13807=CARTESIAN_POINT('Ctrl Pts',(-17.900492838997,7.60176928403058,0.));
#13808=CARTESIAN_POINT('Ctrl Pts',(-17.9482122228183,7.60819152580111,0.));
#13809=CARTESIAN_POINT('Ctrl Pts',(-17.9960506269561,7.61423755067038,0.));
#13810=CARTESIAN_POINT('Ctrl Pts',(-18.0439992897906,7.61992799636654,0.));
#13811=CARTESIAN_POINT('Ctrl Pts',(-18.0920577897363,7.62525915358074,0.));
#13812=CARTESIAN_POINT('Ctrl Pts',(-18.1402306858819,7.63021285851761,0.));
#13813=CARTESIAN_POINT('Ctrl Pts',(-18.1885236169197,7.63476798969016,0.));
#13814=CARTESIAN_POINT('Ctrl Pts',(-18.2369390502576,7.63891299603826,0.));
#13815=CARTESIAN_POINT('Ctrl Pts',(-18.2854741391282,7.6426522027076,0.));
#13816=CARTESIAN_POINT('Ctrl Pts',(-18.3341230095852,7.64599903846601,0.));
#13817=CARTESIAN_POINT('Ctrl Pts',(-18.3828781275628,7.6489719793775,0.));
#13818=CARTESIAN_POINT('Ctrl Pts',(-18.4317319183719,7.65158974829126,0.));
#13819=CARTESIAN_POINT('Ctrl Pts',(-18.4806785483052,7.65386603444743,0.));
#13820=CARTESIAN_POINT('Ctrl Pts',(-18.5297146894905,7.65580722110437,0.));
#13821=CARTESIAN_POINT('Ctrl Pts',(-18.5788385228928,7.65741532450727,0.));
#13822=CARTESIAN_POINT('Ctrl Pts',(-18.6280491346907,7.65868976978872,0.));
#13823=CARTESIAN_POINT('Ctrl Pts',(-18.6773458057584,7.65962948375621,0.));
#13824=CARTESIAN_POINT('Ctrl Pts',(-18.7267272235231,7.66023521705905,0.));
#13825=CARTESIAN_POINT('Ctrl Pts',(-18.7761911671591,7.6605104692254,0.));
#13826=CARTESIAN_POINT('Ctrl Pts',(-18.8257349246207,7.66046025294775,0.));
#13827=CARTESIAN_POINT('Ctrl Pts',(-18.8753555389435,7.66009036321663,0.));
#13828=CARTESIAN_POINT('Ctrl Pts',(-18.9250501008887,7.65940650980099,0.));
#13829=CARTESIAN_POINT('Ctrl Pts',(-18.974816073814,7.65841335587266,0.));
#13830=CARTESIAN_POINT('Ctrl Pts',(-19.0246514144531,7.65711415727855,0.));
#13831=CARTESIAN_POINT('Ctrl Pts',(-19.0745543888799,7.65551129907201,0.));
#13832=CARTESIAN_POINT('Ctrl Pts',(-19.1245234597312,7.65360662280609,0.));
#13833=CARTESIAN_POINT('Ctrl Pts',(-19.1745571539291,7.65140181220526,0.));
#13834=CARTESIAN_POINT('Ctrl Pts',(-19.224653915265,7.64889882291923,0.));
#13835=CARTESIAN_POINT('Ctrl Pts',(-19.2748120456486,7.64610005549613,0.));
#13836=CARTESIAN_POINT('Ctrl Pts',(-19.3250297839295,7.64300812875339,0.));
#13837=CARTESIAN_POINT('Ctrl Pts',(-19.3753053524647,7.63962574822761,0.));
#13838=CARTESIAN_POINT('Ctrl Pts',(-19.4256370121006,7.63595554930654,0.));
#13839=CARTESIAN_POINT('Ctrl Pts',(-19.4760231231881,7.63199992715366,0.));
#13840=CARTESIAN_POINT('Ctrl Pts',(-19.5264621687521,7.62776096538883,0.));
#13841=CARTESIAN_POINT('Ctrl Pts',(-19.5769527121826,7.62324053735219,0.));
#13842=CARTESIAN_POINT('Ctrl Pts',(-19.6274933688524,7.61844037070591,0.));
#13843=CARTESIAN_POINT('Ctrl Pts',(-19.6780827744426,7.61336212350879,0.));
#13844=CARTESIAN_POINT('Ctrl Pts',(-19.7287195480601,7.60800746969262,0.));
#13845=CARTESIAN_POINT('Ctrl Pts',(-19.7794022782484,7.60237814110187,0.));
#13846=CARTESIAN_POINT('Ctrl Pts',(-19.830129556152,7.59647587605448,0.));
#13847=CARTESIAN_POINT('Ctrl Pts',(-19.8808999994024,7.59030238888852,0.));
#13848=CARTESIAN_POINT('Ctrl Pts',(-19.931712276832,7.58385933533352,0.));
#13849=CARTESIAN_POINT('Ctrl Pts',(-19.9825651387294,7.57714827622806,0.));
#13850=CARTESIAN_POINT('Ctrl Pts',(-20.0334574248556,7.57017066105973,0.));
#13851=CARTESIAN_POINT('Ctrl Pts',(-20.0843880130978,7.5629278654946,0.));
#13852=CARTESIAN_POINT('Ctrl Pts',(-20.1353557774357,7.55542122125494,0.));
#13853=CARTESIAN_POINT('Ctrl Pts',(-20.1863595454674,7.54765204869254,0.));
#13854=CARTESIAN_POINT('Ctrl Pts',(-20.2373980474879,7.53962169534167,0.));
#13855=CARTESIAN_POINT('Ctrl Pts',(-20.2884698940944,7.53133155804008,0.));
#13856=CARTESIAN_POINT('Ctrl Pts',(-20.3395736743243,7.52278303006887,0.));
#13857=CARTESIAN_POINT('Ctrl Pts',(-20.3907080367098,7.51397746081994,0.));
#13858=CARTESIAN_POINT('Ctrl Pts',(-20.4418717748497,7.50491611266253,0.));
#13859=CARTESIAN_POINT('Ctrl Pts',(-20.4930639156161,7.49560012018405,0.));
#13860=CARTESIAN_POINT('Ctrl Pts',(-20.5545277683621,7.48411651832413,0.));
#13861=CARTESIAN_POINT('Ctrl Pts',(-20.6057817877246,7.47423073598682,0.));
#13862=CARTESIAN_POINT('Ctrl Pts',(-20.6468066077586,7.46612041736313,0.));
#13863=CARTESIAN_POINT('Ctrl Pts',(-20.6775873630604,7.45992433946825,0.));
#13864=CARTESIAN_POINT('Ctrl Pts',(-20.698113262342,7.45574324794401,0.));
#13865=CARTESIAN_POINT('Ctrl Pts',(-17.2541372868972,7.45007618140238,13.));
#13866=CARTESIAN_POINT('Ctrl Pts',(-17.2687220121555,7.45637364574105,13.));
#13867=CARTESIAN_POINT('Ctrl Pts',(-17.2834550499143,7.46226667104457,13.));
#13868=CARTESIAN_POINT('Ctrl Pts',(-17.2983267669271,7.46778231426201,13.));
#13869=CARTESIAN_POINT('Ctrl Pts',(-17.3157575316218,7.47424706066486,13.));
#13870=CARTESIAN_POINT('Ctrl Pts',(-17.3333785326358,7.48019417754631,13.));
#13871=CARTESIAN_POINT('Ctrl Pts',(-17.3511502187641,7.48573450281641,13.));
#13872=CARTESIAN_POINT('Ctrl Pts',(-17.3761558317125,7.49353000563545,13.));
#13873=CARTESIAN_POINT('Ctrl Pts',(-17.4014574303119,7.50052692940329,13.));
#13874=CARTESIAN_POINT('Ctrl Pts',(-17.4269165094344,7.50711117101308,13.));
#13875=CARTESIAN_POINT('Ctrl Pts',(-17.4438508122093,7.51149073008615,13.));
#13876=CARTESIAN_POINT('Ctrl Pts',(-17.4608540901245,7.51568961154121,13.));
#13877=CARTESIAN_POINT('Ctrl Pts',(-17.4778953549503,7.51979276933068,13.));
#13878=CARTESIAN_POINT('Ctrl Pts',(-17.4958340796436,7.52411201550815,13.));
#13879=CARTESIAN_POINT('Ctrl Pts',(-17.5138146001121,7.5283260217222,13.));
#13880=CARTESIAN_POINT('Ctrl Pts',(-17.5318219263245,7.53247314101481,13.));
#13881=CARTESIAN_POINT('Ctrl Pts',(-17.5518200478112,7.53707874400416,13.));
#13882=CARTESIAN_POINT('Ctrl Pts',(-17.5718516505879,7.54160061545662,13.));
#13883=CARTESIAN_POINT('Ctrl Pts',(-17.5919190740318,7.54602601378866,13.));
#13884=CARTESIAN_POINT('Ctrl Pts',(-17.6221716888658,7.55269751656531,13.));
#13885=CARTESIAN_POINT('Ctrl Pts',(-17.6525076946334,7.5591437511878,13.));
#13886=CARTESIAN_POINT('Ctrl Pts',(-17.6829731243182,7.56521559976737,13.));
#13887=CARTESIAN_POINT('Ctrl Pts',(-17.7051055929372,7.56962666501534,13.));
#13888=CARTESIAN_POINT('Ctrl Pts',(-17.7273074810734,7.57383703866986,13.));
#13889=CARTESIAN_POINT('Ctrl Pts',(-17.7495842479966,7.57782678310862,13.));
#13890=CARTESIAN_POINT('Ctrl Pts',(-17.7768156880398,7.5827039040502,13.));
#13891=CARTESIAN_POINT('Ctrl Pts',(-17.804158605046,7.58725254420512,13.));
#13892=CARTESIAN_POINT('Ctrl Pts',(-17.8315958504836,7.59151733245453,13.));
#13893=CARTESIAN_POINT('Ctrl Pts',(-17.8612326292062,7.59612401157375,13.));
#13894=CARTESIAN_POINT('Ctrl Pts',(-17.8909775513234,7.60040516925881,13.));
#13895=CARTESIAN_POINT('Ctrl Pts',(-17.9207992272113,7.60444696777764,13.));
#13896=CARTESIAN_POINT('Ctrl Pts',(-17.9483304583115,7.60817833718496,13.));
#13897=CARTESIAN_POINT('Ctrl Pts',(-17.9759263069947,7.61170808544359,13.));
#13898=CARTESIAN_POINT('Ctrl Pts',(-18.0035762489806,7.61506270604767,13.));
#13899=CARTESIAN_POINT('Ctrl Pts',(-18.0411401148566,7.61962013038154,13.));
#13900=CARTESIAN_POINT('Ctrl Pts',(-18.0788044381469,7.62385245909619,13.));
#13901=CARTESIAN_POINT('Ctrl Pts',(-18.1165756811382,7.62773031180927,13.));
#13902=CARTESIAN_POINT('Ctrl Pts',(-18.153024114841,7.63147235592348,13.));
#13903=CARTESIAN_POINT('Ctrl Pts',(-18.1895746221693,7.63487692332076,13.));
#13904=CARTESIAN_POINT('Ctrl Pts',(-18.2262298442069,7.63792794642771,13.));
#13905=CARTESIAN_POINT('Ctrl Pts',(-18.2760269903147,7.64207284679906,13.));
#13906=CARTESIAN_POINT('Ctrl Pts',(-18.3260163400117,7.64556831472679,13.));
#13907=CARTESIAN_POINT('Ctrl Pts',(-18.3761647741424,7.64849356609341,13.));
#13908=CARTESIAN_POINT('Ctrl Pts',(-18.4202441575899,7.65106479845398,13.));
#13909=CARTESIAN_POINT('Ctrl Pts',(-18.4644442731264,7.65320196597232,13.));
#13910=CARTESIAN_POINT('Ctrl Pts',(-18.5087513218291,7.65493429570773,13.));
#13911=CARTESIAN_POINT('Ctrl Pts',(-18.5740706685125,7.65748817031392,13.));
#13912=CARTESIAN_POINT('Ctrl Pts',(-18.6396252901455,7.65915358769466,13.));
#13913=CARTESIAN_POINT('Ctrl Pts',(-18.705403439408,7.65993127489916,13.));
#13914=CARTESIAN_POINT('Ctrl Pts',(-18.78841610566,7.66091272374015,13.));
#13915=CARTESIAN_POINT('Ctrl Pts',(-18.8717830756308,7.66048522719313,13.));
#13916=CARTESIAN_POINT('Ctrl Pts',(-18.9554457128649,7.65875983807032,13.));
#13917=CARTESIAN_POINT('Ctrl Pts',(-19.0687732052322,7.65642266547919,13.));
#13918=CARTESIAN_POINT('Ctrl Pts',(-19.1826450749315,7.65169843824091,13.));
#13919=CARTESIAN_POINT('Ctrl Pts',(-19.2969757397446,7.64469887385594,13.));
#13920=CARTESIAN_POINT('Ctrl Pts',(-19.3989045214534,7.63845857890604,13.));
#13921=CARTESIAN_POINT('Ctrl Pts',(-19.5011952233073,7.6304178474504,13.));
#13922=CARTESIAN_POINT('Ctrl Pts',(-19.6037897798545,7.62065725312474,13.));
#13923=CARTESIAN_POINT('Ctrl Pts',(-19.7491944792891,7.60682380686804,13.));
#13924=CARTESIAN_POINT('Ctrl Pts',(-19.8952104297527,7.5895301522803,13.));
#13925=CARTESIAN_POINT('Ctrl Pts',(-20.0416957588587,7.56895177443313,13.));
#13926=CARTESIAN_POINT('Ctrl Pts',(-20.1554820830514,7.55296697931836,13.));
#13927=CARTESIAN_POINT('Ctrl Pts',(-20.2695554960095,7.53499708015271,13.));
#13928=CARTESIAN_POINT('Ctrl Pts',(-20.38385017906,7.51511029031556,13.));
#13929=CARTESIAN_POINT('Ctrl Pts',(-20.4827237158978,7.49790671447922,13.));
#13930=CARTESIAN_POINT('Ctrl Pts',(-20.5817593973802,7.4792711652965,13.));
#13931=CARTESIAN_POINT('Ctrl Pts',(-20.6809436361476,7.45922687874239,13.));
#13932=CARTESIAN_POINT('Ctrl Pts',(-20.6866663413833,7.45807036894775,13.));
#13933=CARTESIAN_POINT('Ctrl Pts',(-20.6923895501261,7.45690915859471,13.));
#13934=CARTESIAN_POINT('Ctrl Pts',(-20.698113262342,7.45574324794401,13.));
#13935=CARTESIAN_POINT('Ctrl Pts',(-18.1978687191668,12.3627494547115,0.));
#13936=CARTESIAN_POINT('Ctrl Pts',(-18.1978687191668,12.3627494547115,21.));
#13937=CARTESIAN_POINT('Ctrl Pts',(-18.1935275957711,12.3532177620787,0.));
#13938=CARTESIAN_POINT('Ctrl Pts',(-18.1935275957711,12.3532177620787,21.));
#13939=CARTESIAN_POINT('Ctrl Pts',(-18.1848265584754,12.3341713636489,0.));
#13940=CARTESIAN_POINT('Ctrl Pts',(-18.1848265584754,12.3341713636489,21.));
#13941=CARTESIAN_POINT('Ctrl Pts',(-18.1717186310224,12.3056527265146,0.));
#13942=CARTESIAN_POINT('Ctrl Pts',(-18.1717186310224,12.3056527265146,21.));
#13943=CARTESIAN_POINT('Ctrl Pts',(-18.1541286139166,12.2677298318549,0.));
#13944=CARTESIAN_POINT('Ctrl Pts',(-18.1541286139166,12.2677298318549,21.));
#13945=CARTESIAN_POINT('Ctrl Pts',(-18.1319528884305,12.2204964278426,0.));
#13946=CARTESIAN_POINT('Ctrl Pts',(-18.1319528884305,12.2204964278426,21.));
#13947=CARTESIAN_POINT('Ctrl Pts',(-18.109588624154,12.1734337668195,0.));
#13948=CARTESIAN_POINT('Ctrl Pts',(-18.109588624154,12.1734337668195,21.));
#13949=CARTESIAN_POINT('Ctrl Pts',(-18.0870354350128,12.1265426519718,0.));
#13950=CARTESIAN_POINT('Ctrl Pts',(-18.0870354350128,12.1265426519718,21.));
#13951=CARTESIAN_POINT('Ctrl Pts',(-18.0642929289333,12.0798241915081,0.));
#13952=CARTESIAN_POINT('Ctrl Pts',(-18.0642929289333,12.0798241915081,21.));
#13953=CARTESIAN_POINT('Ctrl Pts',(-18.0413607600052,12.0332798395991,0.));
#13954=CARTESIAN_POINT('Ctrl Pts',(-18.0413607600052,12.0332798395991,21.));
#13955=CARTESIAN_POINT('Ctrl Pts',(-18.0182386160553,11.986911314246,0.));
#13956=CARTESIAN_POINT('Ctrl Pts',(-18.0182386160553,11.986911314246,21.));
#13957=CARTESIAN_POINT('Ctrl Pts',(-17.9949261997754,11.9407205019619,0.));
#13958=CARTESIAN_POINT('Ctrl Pts',(-17.9949261997754,11.9407205019619,21.));
#13959=CARTESIAN_POINT('Ctrl Pts',(-17.9714232133203,11.8947093631895,0.));
#13960=CARTESIAN_POINT('Ctrl Pts',(-17.9714232133203,11.8947093631895,21.));
#13961=CARTESIAN_POINT('Ctrl Pts',(-17.9477293432951,11.8488798430201,0.));
#13962=CARTESIAN_POINT('Ctrl Pts',(-17.9477293432951,11.8488798430201,21.));
#13963=CARTESIAN_POINT('Ctrl Pts',(-17.9238442458356,11.8032337607271,0.));
#13964=CARTESIAN_POINT('Ctrl Pts',(-17.9238442458356,11.8032337607271,21.));
#13965=CARTESIAN_POINT('Ctrl Pts',(-17.8997675418752,11.7577728408871,0.));
#13966=CARTESIAN_POINT('Ctrl Pts',(-17.8997675418752,11.7577728408871,21.));
#13967=CARTESIAN_POINT('Ctrl Pts',(-17.8754988158862,11.7124987772363,0.));
#13968=CARTESIAN_POINT('Ctrl Pts',(-17.8754988158862,11.7124987772363,21.));
#13969=CARTESIAN_POINT('Ctrl Pts',(-17.8510376144926,11.6674132861792,0.));
#13970=CARTESIAN_POINT('Ctrl Pts',(-17.8510376144926,11.6674132861792,21.));
#13971=CARTESIAN_POINT('Ctrl Pts',(-17.8263834470057,11.6225181583564,0.));
#13972=CARTESIAN_POINT('Ctrl Pts',(-17.8263834470057,11.6225181583564,21.));
#13973=CARTESIAN_POINT('Ctrl Pts',(-17.8015357852426,11.5778153222435,0.));
#13974=CARTESIAN_POINT('Ctrl Pts',(-17.8015357852426,11.5778153222435,21.));
#13975=CARTESIAN_POINT('Ctrl Pts',(-17.7764940721306,11.5333068279911,0.));
#13976=CARTESIAN_POINT('Ctrl Pts',(-17.7764940721306,11.5333068279911,21.));
#13977=CARTESIAN_POINT('Ctrl Pts',(-17.7512577332768,11.4889948016216,0.));
#13978=CARTESIAN_POINT('Ctrl Pts',(-17.7512577332768,11.4889948016216,21.));
#13979=CARTESIAN_POINT('Ctrl Pts',(-17.725826190457,11.4448814046804,0.));
#13980=CARTESIAN_POINT('Ctrl Pts',(-17.725826190457,11.4448814046804,21.));
#13981=CARTESIAN_POINT('Ctrl Pts',(-17.700198872213,11.4009687970126,0.));
#13982=CARTESIAN_POINT('Ctrl Pts',(-17.700198872213,11.4009687970126,21.));
#13983=CARTESIAN_POINT('Ctrl Pts',(-17.674375235974,11.3572590796967,0.));
#13984=CARTESIAN_POINT('Ctrl Pts',(-17.674375235974,11.3572590796967,21.));
#13985=CARTESIAN_POINT('Ctrl Pts',(-17.6483547422688,11.3137543310722,0.));
#13986=CARTESIAN_POINT('Ctrl Pts',(-17.6483547422688,11.3137543310722,21.));
#13987=CARTESIAN_POINT('Ctrl Pts',(-17.6221368072528,11.2704566868205,0.));
#13988=CARTESIAN_POINT('Ctrl Pts',(-17.6221368072528,11.2704566868205,21.));
#13989=CARTESIAN_POINT('Ctrl Pts',(-17.5957207597803,11.2273684103051,0.));
#13990=CARTESIAN_POINT('Ctrl Pts',(-17.5957207597803,11.2273684103051,21.));
#13991=CARTESIAN_POINT('Ctrl Pts',(-17.5691058058227,11.1844919535058,0.));
#13992=CARTESIAN_POINT('Ctrl Pts',(-17.5691058058227,11.1844919535058,21.));
#13993=CARTESIAN_POINT('Ctrl Pts',(-17.5422909714139,11.1418300507683,0.));
#13994=CARTESIAN_POINT('Ctrl Pts',(-17.5422909714139,11.1418300507683,21.));
#13995=CARTESIAN_POINT('Ctrl Pts',(-17.5152751467292,11.0993856581394,0.));
#13996=CARTESIAN_POINT('Ctrl Pts',(-17.5152751467292,11.0993856581394,21.));
#13997=CARTESIAN_POINT('Ctrl Pts',(-17.4880571878157,11.0571618040371,0.));
#13998=CARTESIAN_POINT('Ctrl Pts',(-17.4880571878157,11.0571618040371,21.));
#13999=CARTESIAN_POINT('Ctrl Pts',(-17.460636011184,11.0151614525642,0.));
#14000=CARTESIAN_POINT('Ctrl Pts',(-17.460636011184,11.0151614525642,21.));
#14001=CARTESIAN_POINT('Ctrl Pts',(-17.4330106728622,10.9733873885115,0.));
#14002=CARTESIAN_POINT('Ctrl Pts',(-17.4330106728622,10.9733873885115,21.));
#14003=CARTESIAN_POINT('Ctrl Pts',(-17.4051805054129,10.9318420203801,0.));
#14004=CARTESIAN_POINT('Ctrl Pts',(-17.4051805054129,10.9318420203801,21.));
#14005=CARTESIAN_POINT('Ctrl Pts',(-17.377145012528,10.8905275295837,0.));
#14006=CARTESIAN_POINT('Ctrl Pts',(-17.377145012528,10.8905275295837,21.));
#14007=CARTESIAN_POINT('Ctrl Pts',(-17.3489036079991,10.8494462423128,0.));
#14008=CARTESIAN_POINT('Ctrl Pts',(-17.3489036079991,10.8494462423128,21.));
#14009=CARTESIAN_POINT('Ctrl Pts',(-17.3204553814537,10.8086009632423,0.));
#14010=CARTESIAN_POINT('Ctrl Pts',(-17.3204553814537,10.8086009632423,21.));
#14011=CARTESIAN_POINT('Ctrl Pts',(-17.2917988998581,10.7679952591482,0.));
#14012=CARTESIAN_POINT('Ctrl Pts',(-17.2917988998581,10.7679952591482,21.));
#14013=CARTESIAN_POINT('Ctrl Pts',(-17.2629318816279,10.7276339231608,0.));
#14014=CARTESIAN_POINT('Ctrl Pts',(-17.2629318816279,10.7276339231608,21.));
#14015=CARTESIAN_POINT('Ctrl Pts',(-17.2338514174708,10.6875226650217,0.));
#14016=CARTESIAN_POINT('Ctrl Pts',(-17.2338514174708,10.6875226650217,21.));
#14017=CARTESIAN_POINT('Ctrl Pts',(-17.2045545572011,10.6476672831754,0.));
#14018=CARTESIAN_POINT('Ctrl Pts',(-17.2045545572011,10.6476672831754,21.));
#14019=CARTESIAN_POINT('Ctrl Pts',(-17.1750388395657,10.6080729180997,0.));
#14020=CARTESIAN_POINT('Ctrl Pts',(-17.1750388395657,10.6080729180997,21.));
#14021=CARTESIAN_POINT('Ctrl Pts',(-17.1453027387554,10.5687434234512,0.));
#14022=CARTESIAN_POINT('Ctrl Pts',(-17.1453027387554,10.5687434234512,21.));
#14023=CARTESIAN_POINT('Ctrl Pts',(-17.1153464189932,10.5296803023445,0.));
#14024=CARTESIAN_POINT('Ctrl Pts',(-17.1153464189932,10.5296803023445,21.));
#14025=CARTESIAN_POINT('Ctrl Pts',(-17.0851711712016,10.4908835057575,0.));
#14026=CARTESIAN_POINT('Ctrl Pts',(-17.0851711712016,10.4908835057575,21.));
#14027=CARTESIAN_POINT('Ctrl Pts',(-17.0547779975888,10.452353435089,0.));
#14028=CARTESIAN_POINT('Ctrl Pts',(-17.0547779975888,10.452353435089,21.));
#14029=CARTESIAN_POINT('Ctrl Pts',(-17.0241663361802,10.4140927470882,0.));
#14030=CARTESIAN_POINT('Ctrl Pts',(-17.0241663361802,10.4140927470882,21.));
#14031=CARTESIAN_POINT('Ctrl Pts',(-16.9933329788855,10.3761078860454,0.));
#14032=CARTESIAN_POINT('Ctrl Pts',(-16.9933329788855,10.3761078860454,21.));
#14033=CARTESIAN_POINT('Ctrl Pts',(-16.9622702798438,10.3384116178624,0.));
#14034=CARTESIAN_POINT('Ctrl Pts',(-16.9622702798438,10.3384116178624,21.));
#14035=CARTESIAN_POINT('Ctrl Pts',(-16.9309675442425,10.3010210756062,0.));
#14036=CARTESIAN_POINT('Ctrl Pts',(-16.9309675442425,10.3010210756062,21.));
#14037=CARTESIAN_POINT('Ctrl Pts',(-16.8994142530447,10.2639532144219,0.));
#14038=CARTESIAN_POINT('Ctrl Pts',(-16.8994142530447,10.2639532144219,21.));
#14039=CARTESIAN_POINT('Ctrl Pts',(-16.8676029947679,10.2272206796636,0.));
#14040=CARTESIAN_POINT('Ctrl Pts',(-16.8676029947679,10.2272206796636,21.));
#14041=CARTESIAN_POINT('Ctrl Pts',(-16.8355319435838,10.1908283166713,0.));
#14042=CARTESIAN_POINT('Ctrl Pts',(-16.8355319435838,10.1908283166713,21.));
#14043=CARTESIAN_POINT('Ctrl Pts',(-16.8032089941901,10.1547673397274,0.));
#14044=CARTESIAN_POINT('Ctrl Pts',(-16.8032089941901,10.1547673397274,21.));
#14045=CARTESIAN_POINT('Ctrl Pts',(-16.7706479198888,10.1190207721353,0.));
#14046=CARTESIAN_POINT('Ctrl Pts',(-16.7706479198888,10.1190207721353,21.));
#14047=CARTESIAN_POINT('Ctrl Pts',(-16.7378607357337,10.0835742491038,0.));
#14048=CARTESIAN_POINT('Ctrl Pts',(-16.7378607357337,10.0835742491038,21.));
#14049=CARTESIAN_POINT('Ctrl Pts',(-16.7048506904207,10.0484259314257,0.));
#14050=CARTESIAN_POINT('Ctrl Pts',(-16.7048506904207,10.0484259314257,21.));
#14051=CARTESIAN_POINT('Ctrl Pts',(-16.6716062376277,10.0135950379525,0.));
#14052=CARTESIAN_POINT('Ctrl Pts',(-16.6716062376277,10.0135950379525,21.));
#14053=CARTESIAN_POINT('Ctrl Pts',(-16.6380914029057,9.97913546489641,0.));
#14054=CARTESIAN_POINT('Ctrl Pts',(-16.6380914029057,9.97913546489641,21.));
#14055=CARTESIAN_POINT('Ctrl Pts',(-16.6042559779574,9.9451214271291,0.));
#14056=CARTESIAN_POINT('Ctrl Pts',(-16.6042559779574,9.9451214271291,21.));
#14057=CARTESIAN_POINT('Ctrl Pts',(-16.5700527532381,9.91162317616649,0.));
#14058=CARTESIAN_POINT('Ctrl Pts',(-16.5700527532381,9.91162317616649,21.));
#14059=CARTESIAN_POINT('Ctrl Pts',(-16.5354535643506,9.8786843754698,0.));
#14060=CARTESIAN_POINT('Ctrl Pts',(-16.5354535643506,9.8786843754698,21.));
#14061=CARTESIAN_POINT('Ctrl Pts',(-16.5004633692332,9.84630229363522,0.));
#14062=CARTESIAN_POINT('Ctrl Pts',(-16.5004633692332,9.84630229363522,21.));
#14063=CARTESIAN_POINT('Ctrl Pts',(-16.4651416449558,9.81439757053279,0.));
#14064=CARTESIAN_POINT('Ctrl Pts',(-16.4651416449558,9.81439757053279,21.));
#14065=CARTESIAN_POINT('Ctrl Pts',(-16.4295725710378,9.78285689698057,0.));
#14066=CARTESIAN_POINT('Ctrl Pts',(-16.4295725710378,9.78285689698057,21.));
#14067=CARTESIAN_POINT('Ctrl Pts',(-16.3938231282759,9.75159288382685,0.));
#14068=CARTESIAN_POINT('Ctrl Pts',(-16.3938231282759,9.75159288382685,21.));
#14069=CARTESIAN_POINT('Ctrl Pts',(-16.3579039682519,9.72060002001012,0.));
#14070=CARTESIAN_POINT('Ctrl Pts',(-16.3579039682519,9.72060002001012,21.));
#14071=CARTESIAN_POINT('Ctrl Pts',(-16.3217321000366,9.69000797146315,0.));
#14072=CARTESIAN_POINT('Ctrl Pts',(-16.3217321000366,9.69000797146315,21.));
#14073=CARTESIAN_POINT('Ctrl Pts',(-16.2850845948324,9.66014786078746,0.));
#14074=CARTESIAN_POINT('Ctrl Pts',(-16.2850845948324,9.66014786078746,21.));
#14075=CARTESIAN_POINT('Ctrl Pts',(-16.2476599387841,9.63146315443273,0.));
#14076=CARTESIAN_POINT('Ctrl Pts',(-16.2476599387841,9.63146315443273,21.));
#14077=CARTESIAN_POINT('Ctrl Pts',(-16.2168537871666,9.60981421781524,0.));
#14078=CARTESIAN_POINT('Ctrl Pts',(-16.2168537871666,9.60981421781524,21.));
#14079=CARTESIAN_POINT('Ctrl Pts',(-16.1931534965272,9.59446643316597,0.));
#14080=CARTESIAN_POINT('Ctrl Pts',(-16.1931534965272,9.59446643316597,21.));
#14081=CARTESIAN_POINT('Ctrl Pts',(-16.1770747160769,9.58464985151483,0.));
#14082=CARTESIAN_POINT('Ctrl Pts',(-16.1770747160769,9.58464985151483,21.));
#14083=CARTESIAN_POINT('Ctrl Pts',(-16.1689656784104,9.57984538049455,0.));
#14084=CARTESIAN_POINT('Ctrl Pts',(-16.1689656784104,9.57984538049455,21.));
#14085=CARTESIAN_POINT('',(-18.1978687191669,12.3627494547114,0.));
#14086=CARTESIAN_POINT('Ctrl Pts',(-16.1689656784104,9.57984538049455,0.));
#14087=CARTESIAN_POINT('Ctrl Pts',(-16.1770747160769,9.58464985151483,0.));
#14088=CARTESIAN_POINT('Ctrl Pts',(-16.1931534965272,9.59446643316597,0.));
#14089=CARTESIAN_POINT('Ctrl Pts',(-16.2168537871666,9.60981421781524,0.));
#14090=CARTESIAN_POINT('Ctrl Pts',(-16.2476599387841,9.63146315443273,0.));
#14091=CARTESIAN_POINT('Ctrl Pts',(-16.2850845948324,9.66014786078746,0.));
#14092=CARTESIAN_POINT('Ctrl Pts',(-16.3217321000366,9.69000797146315,0.));
#14093=CARTESIAN_POINT('Ctrl Pts',(-16.3579039682519,9.72060002001012,0.));
#14094=CARTESIAN_POINT('Ctrl Pts',(-16.3938231282759,9.75159288382685,0.));
#14095=CARTESIAN_POINT('Ctrl Pts',(-16.4295725710378,9.78285689698057,0.));
#14096=CARTESIAN_POINT('Ctrl Pts',(-16.4651416449558,9.81439757053279,0.));
#14097=CARTESIAN_POINT('Ctrl Pts',(-16.5004633692332,9.84630229363522,0.));
#14098=CARTESIAN_POINT('Ctrl Pts',(-16.5354535643506,9.8786843754698,0.));
#14099=CARTESIAN_POINT('Ctrl Pts',(-16.5700527532381,9.91162317616649,0.));
#14100=CARTESIAN_POINT('Ctrl Pts',(-16.6042559779574,9.9451214271291,0.));
#14101=CARTESIAN_POINT('Ctrl Pts',(-16.6380914029057,9.97913546489641,0.));
#14102=CARTESIAN_POINT('Ctrl Pts',(-16.6716062376277,10.0135950379525,0.));
#14103=CARTESIAN_POINT('Ctrl Pts',(-16.7048506904207,10.0484259314257,0.));
#14104=CARTESIAN_POINT('Ctrl Pts',(-16.7378607357337,10.0835742491038,0.));
#14105=CARTESIAN_POINT('Ctrl Pts',(-16.7706479198888,10.1190207721353,0.));
#14106=CARTESIAN_POINT('Ctrl Pts',(-16.8032089941901,10.1547673397274,0.));
#14107=CARTESIAN_POINT('Ctrl Pts',(-16.8355319435838,10.1908283166713,0.));
#14108=CARTESIAN_POINT('Ctrl Pts',(-16.8676029947679,10.2272206796636,0.));
#14109=CARTESIAN_POINT('Ctrl Pts',(-16.8994142530447,10.2639532144219,0.));
#14110=CARTESIAN_POINT('Ctrl Pts',(-16.9309675442425,10.3010210756062,0.));
#14111=CARTESIAN_POINT('Ctrl Pts',(-16.9622702798438,10.3384116178624,0.));
#14112=CARTESIAN_POINT('Ctrl Pts',(-16.9933329788855,10.3761078860454,0.));
#14113=CARTESIAN_POINT('Ctrl Pts',(-17.0241663361802,10.4140927470882,0.));
#14114=CARTESIAN_POINT('Ctrl Pts',(-17.0547779975888,10.452353435089,0.));
#14115=CARTESIAN_POINT('Ctrl Pts',(-17.0851711712016,10.4908835057575,0.));
#14116=CARTESIAN_POINT('Ctrl Pts',(-17.1153464189932,10.5296803023445,0.));
#14117=CARTESIAN_POINT('Ctrl Pts',(-17.1453027387554,10.5687434234512,0.));
#14118=CARTESIAN_POINT('Ctrl Pts',(-17.1750388395657,10.6080729180997,0.));
#14119=CARTESIAN_POINT('Ctrl Pts',(-17.2045545572011,10.6476672831754,0.));
#14120=CARTESIAN_POINT('Ctrl Pts',(-17.2338514174708,10.6875226650217,0.));
#14121=CARTESIAN_POINT('Ctrl Pts',(-17.2629318816279,10.7276339231608,0.));
#14122=CARTESIAN_POINT('Ctrl Pts',(-17.2917988998581,10.7679952591482,0.));
#14123=CARTESIAN_POINT('Ctrl Pts',(-17.3204553814537,10.8086009632423,0.));
#14124=CARTESIAN_POINT('Ctrl Pts',(-17.3489036079991,10.8494462423128,0.));
#14125=CARTESIAN_POINT('Ctrl Pts',(-17.377145012528,10.8905275295837,0.));
#14126=CARTESIAN_POINT('Ctrl Pts',(-17.4051805054129,10.9318420203801,0.));
#14127=CARTESIAN_POINT('Ctrl Pts',(-17.4330106728622,10.9733873885115,0.));
#14128=CARTESIAN_POINT('Ctrl Pts',(-17.460636011184,11.0151614525642,0.));
#14129=CARTESIAN_POINT('Ctrl Pts',(-17.4880571878157,11.0571618040371,0.));
#14130=CARTESIAN_POINT('Ctrl Pts',(-17.5152751467292,11.0993856581394,0.));
#14131=CARTESIAN_POINT('Ctrl Pts',(-17.5422909714139,11.1418300507683,0.));
#14132=CARTESIAN_POINT('Ctrl Pts',(-17.5691058058227,11.1844919535058,0.));
#14133=CARTESIAN_POINT('Ctrl Pts',(-17.5957207597803,11.2273684103051,0.));
#14134=CARTESIAN_POINT('Ctrl Pts',(-17.6221368072528,11.2704566868205,0.));
#14135=CARTESIAN_POINT('Ctrl Pts',(-17.6483547422688,11.3137543310722,0.));
#14136=CARTESIAN_POINT('Ctrl Pts',(-17.674375235974,11.3572590796967,0.));
#14137=CARTESIAN_POINT('Ctrl Pts',(-17.700198872213,11.4009687970126,0.));
#14138=CARTESIAN_POINT('Ctrl Pts',(-17.725826190457,11.4448814046804,0.));
#14139=CARTESIAN_POINT('Ctrl Pts',(-17.7512577332768,11.4889948016216,0.));
#14140=CARTESIAN_POINT('Ctrl Pts',(-17.7764940721306,11.5333068279911,0.));
#14141=CARTESIAN_POINT('Ctrl Pts',(-17.8015357852426,11.5778153222435,0.));
#14142=CARTESIAN_POINT('Ctrl Pts',(-17.8263834470057,11.6225181583564,0.));
#14143=CARTESIAN_POINT('Ctrl Pts',(-17.8510376144926,11.6674132861792,0.));
#14144=CARTESIAN_POINT('Ctrl Pts',(-17.8754988158862,11.7124987772363,0.));
#14145=CARTESIAN_POINT('Ctrl Pts',(-17.8997675418752,11.7577728408871,0.));
#14146=CARTESIAN_POINT('Ctrl Pts',(-17.9238442458356,11.8032337607271,0.));
#14147=CARTESIAN_POINT('Ctrl Pts',(-17.9477293432951,11.8488798430201,0.));
#14148=CARTESIAN_POINT('Ctrl Pts',(-17.9714232133203,11.8947093631895,0.));
#14149=CARTESIAN_POINT('Ctrl Pts',(-17.9949261997754,11.9407205019619,0.));
#14150=CARTESIAN_POINT('Ctrl Pts',(-18.0182386160553,11.986911314246,0.));
#14151=CARTESIAN_POINT('Ctrl Pts',(-18.0413607600052,12.0332798395991,0.));
#14152=CARTESIAN_POINT('Ctrl Pts',(-18.0642929289333,12.0798241915081,0.));
#14153=CARTESIAN_POINT('Ctrl Pts',(-18.0870354350128,12.1265426519718,0.));
#14154=CARTESIAN_POINT('Ctrl Pts',(-18.109588624154,12.1734337668195,0.));
#14155=CARTESIAN_POINT('Ctrl Pts',(-18.1364257412858,12.2299089600472,0.));
#14156=CARTESIAN_POINT('Ctrl Pts',(-18.1585543320743,12.2771850498068,0.));
#14157=CARTESIAN_POINT('Ctrl Pts',(-18.1761067306718,12.3151419520839,0.));
#14158=CARTESIAN_POINT('Ctrl Pts',(-18.1891864723772,12.3436860694314,0.));
#14159=CARTESIAN_POINT('Ctrl Pts',(-18.1978687191668,12.3627494547115,0.));
#14160=CARTESIAN_POINT('',(-18.1978687191669,12.3627494547114,13.));
#14161=CARTESIAN_POINT('Ctrl Pts',(-18.1978687191668,12.3627494547115,13.));
#14162=CARTESIAN_POINT('Ctrl Pts',(-18.1551298837072,12.2689088964153,13.));
#14163=CARTESIAN_POINT('Ctrl Pts',(-18.111299637656,12.1760519707549,13.));
#14164=CARTESIAN_POINT('Ctrl Pts',(-18.0663670681848,12.0842021157222,13.));
#14165=CARTESIAN_POINT('Ctrl Pts',(-17.9919118454842,11.9320029094011,13.));
#14166=CARTESIAN_POINT('Ctrl Pts',(-17.9144310022929,11.7825824042094,13.));
#14167=CARTESIAN_POINT('Ctrl Pts',(-17.8338669529311,11.6362239728201,13.));
#14168=CARTESIAN_POINT('Ctrl Pts',(-17.7719406994714,11.523724298462,13.));
#14169=CARTESIAN_POINT('Ctrl Pts',(-17.708190453754,11.4130324604454,13.));
#14170=CARTESIAN_POINT('Ctrl Pts',(-17.6425762029941,11.3042990938976,13.));
#14171=CARTESIAN_POINT('Ctrl Pts',(-17.571944040219,11.1872502400868,13.));
#14172=CARTESIAN_POINT('Ctrl Pts',(-17.499154807149,11.0724652191949,13.));
#14173=CARTESIAN_POINT('Ctrl Pts',(-17.4241207695605,10.9601920980076,13.));
#14174=CARTESIAN_POINT('Ctrl Pts',(-17.3825798919753,10.8980346540897,13.));
#14175=CARTESIAN_POINT('Ctrl Pts',(-17.3403540655037,10.8366430107889,13.));
#14176=CARTESIAN_POINT('Ctrl Pts',(-17.2974271318847,10.7760628634082,13.));
#14177=CARTESIAN_POINT('Ctrl Pts',(-17.2560610466519,10.71768544558,13.));
#14178=CARTESIAN_POINT('Ctrl Pts',(-17.2140399833079,10.6600671046061,13.));
#14179=CARTESIAN_POINT('Ctrl Pts',(-17.1713305004863,10.6032772242041,13.));
#14180=CARTESIAN_POINT('Ctrl Pts',(-17.1344164148599,10.5541933587631,13.));
#14181=CARTESIAN_POINT('Ctrl Pts',(-17.096989955235,10.5057257098335,13.));
#14182=CARTESIAN_POINT('Ctrl Pts',(-17.0590571075016,10.4578814177545,13.));
#14183=CARTESIAN_POINT('Ctrl Pts',(-17.0318344187272,10.423545733757,13.));
#14184=CARTESIAN_POINT('Ctrl Pts',(-17.004352569251,10.3895287972434,13.));
#14185=CARTESIAN_POINT('Ctrl Pts',(-16.9765917293735,10.3558648787318,13.));
#14186=CARTESIAN_POINT('Ctrl Pts',(-16.9492829411712,10.3227491363857,13.));
#14187=CARTESIAN_POINT('Ctrl Pts',(-16.9217004795811,10.2899802165512,13.));
#14188=CARTESIAN_POINT('Ctrl Pts',(-16.8938171684013,10.257603002843,13.));
#14189=CARTESIAN_POINT('Ctrl Pts',(-16.8696406992028,10.2295300560935,13.));
#14190=CARTESIAN_POINT('Ctrl Pts',(-16.8452366235594,10.2017536135352,13.));
#14191=CARTESIAN_POINT('Ctrl Pts',(-16.8206160301345,10.1742626909659,13.));
#14192=CARTESIAN_POINT('Ctrl Pts',(-16.7983154204895,10.1493622215735,13.));
#14193=CARTESIAN_POINT('Ctrl Pts',(-16.7758403904972,10.1246914564006,13.));
#14194=CARTESIAN_POINT('Ctrl Pts',(-16.7532063442149,10.1002324979069,13.));
#14195=CARTESIAN_POINT('Ctrl Pts',(-16.7341406196096,10.079629563683,13.));
#14196=CARTESIAN_POINT('Ctrl Pts',(-16.7149630708293,10.0591755003946,13.));
#14197=CARTESIAN_POINT('Ctrl Pts',(-16.6956634327229,10.0388873687047,13.));
#14198=CARTESIAN_POINT('Ctrl Pts',(-16.6677347574757,10.0095282357399,13.));
#14199=CARTESIAN_POINT('Ctrl Pts',(-16.6395499070626,9.98051721208624,13.));
#14200=CARTESIAN_POINT('Ctrl Pts',(-16.6109867038064,9.95203577377263,13.));
#14201=CARTESIAN_POINT('Ctrl Pts',(-16.5937277075416,9.9348261830604,13.));
#14202=CARTESIAN_POINT('Ctrl Pts',(-16.5763285722608,9.91781279953151,13.));
#14203=CARTESIAN_POINT('Ctrl Pts',(-16.5587751451304,9.90101792991858,13.));
#14204=CARTESIAN_POINT('Ctrl Pts',(-16.5425859473257,9.88552833553625,13.));
#14205=CARTESIAN_POINT('Ctrl Pts',(-16.5262647433908,9.87022569084434,13.));
#14206=CARTESIAN_POINT('Ctrl Pts',(-16.5098269904329,9.85509024411449,13.));
#14207=CARTESIAN_POINT('Ctrl Pts',(-16.4872151946467,9.83426990258338,13.));
#14208=CARTESIAN_POINT('Ctrl Pts',(-16.4643869859202,9.81375991310154,13.));
#14209=CARTESIAN_POINT('Ctrl Pts',(-16.4414328801903,9.7934396802235,13.));
#14210=CARTESIAN_POINT('Ctrl Pts',(-16.4268703865311,9.7805481624305,13.));
#14211=CARTESIAN_POINT('Ctrl Pts',(-16.4122582103724,9.76773166757831,13.));
#14212=CARTESIAN_POINT('Ctrl Pts',(-16.3976025796313,9.75498419478216,13.));
#14213=CARTESIAN_POINT('Ctrl Pts',(-16.3844498331849,9.74354393127652,13.));
#14214=CARTESIAN_POINT('Ctrl Pts',(-16.3712625079592,9.73215866496981,13.));
#14215=CARTESIAN_POINT('Ctrl Pts',(-16.3580219469452,9.72085751043954,13.));
#14216=CARTESIAN_POINT('Ctrl Pts',(-16.3441034802572,9.70897774622862,13.));
#14217=CARTESIAN_POINT('Ctrl Pts',(-16.330126283354,9.69719080116679,13.));
#14218=CARTESIAN_POINT('Ctrl Pts',(-16.3160331239166,9.68558166507924,13.));
#14219=CARTESIAN_POINT('Ctrl Pts',(-16.292624417431,9.66629891585391,13.));
#14220=CARTESIAN_POINT('Ctrl Pts',(-16.268891093964,9.64751373148189,13.));
#14221=CARTESIAN_POINT('Ctrl Pts',(-16.2444806681934,9.62974342615828,13.));
#14222=CARTESIAN_POINT('Ctrl Pts',(-16.231019890619,9.61994424733045,13.));
#14223=CARTESIAN_POINT('Ctrl Pts',(-16.2173524098339,9.61045478083913,13.));
#14224=CARTESIAN_POINT('Ctrl Pts',(-16.2034347659916,9.60133856554245,13.));
#14225=CARTESIAN_POINT('Ctrl Pts',(-16.1921134806533,9.59392299464928,13.));
#14226=CARTESIAN_POINT('Ctrl Pts',(-16.1806266997688,9.58675434324541,13.));
#14227=CARTESIAN_POINT('Ctrl Pts',(-16.1689656784104,9.57984538049455,13.));
#14228=CARTESIAN_POINT('',(-18.1978687191669,12.3627494547114,0.));
#14229=CARTESIAN_POINT('Origin',(-4.58435815896522E-12,3.33073116609659E-12,
0.));
#14230=CARTESIAN_POINT('',(-17.3811241238545,13.4869019493419,0.));
#14231=CARTESIAN_POINT('Origin',(-4.58435815896522E-12,3.33073116609659E-12,
0.));
#14232=CARTESIAN_POINT('',(-17.3811241238545,13.4869019493419,13.));
#14233=CARTESIAN_POINT('Origin',(-4.58435815896522E-12,3.33073116609659E-12,
13.));
#14234=CARTESIAN_POINT('',(-17.3811241238545,13.4869019493419,0.));
#14235=CARTESIAN_POINT('Ctrl Pts',(-14.1074595503134,12.4172651441477,0.));
#14236=CARTESIAN_POINT('Ctrl Pts',(-14.1074595503134,12.4172651441477,21.));
#14237=CARTESIAN_POINT('Ctrl Pts',(-14.1145347042316,12.4234926340671,0.));
#14238=CARTESIAN_POINT('Ctrl Pts',(-14.1145347042316,12.4234926340671,21.));
#14239=CARTESIAN_POINT('Ctrl Pts',(-14.1288394445866,12.4357509724316,0.));
#14240=CARTESIAN_POINT('Ctrl Pts',(-14.1288394445866,12.4357509724316,21.));
#14241=CARTESIAN_POINT('Ctrl Pts',(-14.1507598477672,12.4535485619996,0.));
#14242=CARTESIAN_POINT('Ctrl Pts',(-14.1507598477672,12.4535485619996,21.));
#14243=CARTESIAN_POINT('Ctrl Pts',(-14.1808688343892,12.4761570639125,0.));
#14244=CARTESIAN_POINT('Ctrl Pts',(-14.1808688343892,12.4761570639125,21.));
#14245=CARTESIAN_POINT('Ctrl Pts',(-14.2197144660135,12.5028859651751,0.));
#14246=CARTESIAN_POINT('Ctrl Pts',(-14.2197144660135,12.5028859651751,21.));
#14247=CARTESIAN_POINT('Ctrl Pts',(-14.2594378207584,12.5285125321527,0.));
#14248=CARTESIAN_POINT('Ctrl Pts',(-14.2594378207584,12.5285125321527,21.));
#14249=CARTESIAN_POINT('Ctrl Pts',(-14.2997103098726,12.5534605602317,0.));
#14250=CARTESIAN_POINT('Ctrl Pts',(-14.2997103098726,12.5534605602317,21.));
#14251=CARTESIAN_POINT('Ctrl Pts',(-14.3402859058353,12.5780443898087,0.));
#14252=CARTESIAN_POINT('Ctrl Pts',(-14.3402859058353,12.5780443898087,21.));
#14253=CARTESIAN_POINT('Ctrl Pts',(-14.3810669346235,12.6023830189244,0.));
#14254=CARTESIAN_POINT('Ctrl Pts',(-14.3810669346235,12.6023830189244,21.));
#14255=CARTESIAN_POINT('Ctrl Pts',(-14.4220553460485,12.626464614311,0.));
#14256=CARTESIAN_POINT('Ctrl Pts',(-14.4220553460485,12.626464614311,21.));
#14257=CARTESIAN_POINT('Ctrl Pts',(-14.463313553928,12.6501984687124,0.));
#14258=CARTESIAN_POINT('Ctrl Pts',(-14.463313553928,12.6501984687124,21.));
#14259=CARTESIAN_POINT('Ctrl Pts',(-14.5049233087958,12.6734695081852,0.));
#14260=CARTESIAN_POINT('Ctrl Pts',(-14.5049233087958,12.6734695081852,21.));
#14261=CARTESIAN_POINT('Ctrl Pts',(-14.5469417071951,12.6961966430455,0.));
#14262=CARTESIAN_POINT('Ctrl Pts',(-14.5469417071951,12.6961966430455,21.));
#14263=CARTESIAN_POINT('Ctrl Pts',(-14.5893698147583,12.7183743139638,0.));
#14264=CARTESIAN_POINT('Ctrl Pts',(-14.5893698147583,12.7183743139638,21.));
#14265=CARTESIAN_POINT('Ctrl Pts',(-14.6321748083434,12.7400427996251,0.));
#14266=CARTESIAN_POINT('Ctrl Pts',(-14.6321748083434,12.7400427996251,21.));
#14267=CARTESIAN_POINT('Ctrl Pts',(-14.6753044633399,12.7612687078867,0.));
#14268=CARTESIAN_POINT('Ctrl Pts',(-14.6753044633399,12.7612687078867,21.));
#14269=CARTESIAN_POINT('Ctrl Pts',(-14.7187037124277,12.7821227233337,0.));
#14270=CARTESIAN_POINT('Ctrl Pts',(-14.7187037124277,12.7821227233337,21.));
#14271=CARTESIAN_POINT('Ctrl Pts',(-14.7623324139791,12.8026557145457,0.));
#14272=CARTESIAN_POINT('Ctrl Pts',(-14.7623324139791,12.8026557145457,21.));
#14273=CARTESIAN_POINT('Ctrl Pts',(-14.8061758577898,12.8228846016791,0.));
#14274=CARTESIAN_POINT('Ctrl Pts',(-14.8061758577898,12.8228846016791,21.));
#14275=CARTESIAN_POINT('Ctrl Pts',(-14.8502347891476,12.8428057266944,0.));
#14276=CARTESIAN_POINT('Ctrl Pts',(-14.8502347891476,12.8428057266944,21.));
#14277=CARTESIAN_POINT('Ctrl Pts',(-14.8945191569251,12.8624032236317,0.));
#14278=CARTESIAN_POINT('Ctrl Pts',(-14.8945191569251,12.8624032236317,21.));
#14279=CARTESIAN_POINT('Ctrl Pts',(-14.9390408507356,12.8816587472147,0.));
#14280=CARTESIAN_POINT('Ctrl Pts',(-14.9390408507356,12.8816587472147,21.));
#14281=CARTESIAN_POINT('Ctrl Pts',(-14.9838057866976,12.9005620742036,0.));
#14282=CARTESIAN_POINT('Ctrl Pts',(-14.9838057866976,12.9005620742036,21.));
#14283=CARTESIAN_POINT('Ctrl Pts',(-15.0288099208306,12.9191164383568,0.));
#14284=CARTESIAN_POINT('Ctrl Pts',(-15.0288099208306,12.9191164383568,21.));
#14285=CARTESIAN_POINT('Ctrl Pts',(-15.0740435169624,12.9373327960422,0.));
#14286=CARTESIAN_POINT('Ctrl Pts',(-15.0740435169624,12.9373327960422,21.));
#14287=CARTESIAN_POINT('Ctrl Pts',(-15.1194937003528,12.9552263908864,0.));
#14288=CARTESIAN_POINT('Ctrl Pts',(-15.1194937003528,12.9552263908864,21.));
#14289=CARTESIAN_POINT('Ctrl Pts',(-15.1651474813659,12.9728126886697,0.));
#14290=CARTESIAN_POINT('Ctrl Pts',(-15.1651474813659,12.9728126886697,21.));
#14291=CARTESIAN_POINT('Ctrl Pts',(-15.2109950816083,12.9901029059182,0.));
#14292=CARTESIAN_POINT('Ctrl Pts',(-15.2109950816083,12.9901029059182,21.));
#14293=CARTESIAN_POINT('Ctrl Pts',(-15.2570313635503,13.0071020851025,0.));
#14294=CARTESIAN_POINT('Ctrl Pts',(-15.2570313635503,13.0071020851025,21.));
#14295=CARTESIAN_POINT('Ctrl Pts',(-15.3032539741328,13.0238115816728,0.));
#14296=CARTESIAN_POINT('Ctrl Pts',(-15.3032539741328,13.0238115816728,21.));
#14297=CARTESIAN_POINT('Ctrl Pts',(-15.3496622219036,13.0402305665115,0.));
#14298=CARTESIAN_POINT('Ctrl Pts',(-15.3496622219036,13.0402305665115,21.));
#14299=CARTESIAN_POINT('Ctrl Pts',(-15.3962557545684,13.0563577967298,0.));
#14300=CARTESIAN_POINT('Ctrl Pts',(-15.3962557545684,13.0563577967298,21.));
#14301=CARTESIAN_POINT('Ctrl Pts',(-15.4430330918328,13.0721935806302,0.));
#14302=CARTESIAN_POINT('Ctrl Pts',(-15.4430330918328,13.0721935806302,21.));
#14303=CARTESIAN_POINT('Ctrl Pts',(-15.4899910401523,13.087740560189,0.));
#14304=CARTESIAN_POINT('Ctrl Pts',(-15.4899910401523,13.087740560189,21.));
#14305=CARTESIAN_POINT('Ctrl Pts',(-15.5371254712111,13.1030026646917,0.));
#14306=CARTESIAN_POINT('Ctrl Pts',(-15.5371254712111,13.1030026646917,21.));
#14307=CARTESIAN_POINT('Ctrl Pts',(-15.5844317820184,13.1179844917497,0.));
#14308=CARTESIAN_POINT('Ctrl Pts',(-15.5844317820184,13.1179844917497,21.));
#14309=CARTESIAN_POINT('Ctrl Pts',(-15.6319054413079,13.1326905726717,0.));
#14310=CARTESIAN_POINT('Ctrl Pts',(-15.6319054413079,13.1326905726717,21.));
#14311=CARTESIAN_POINT('Ctrl Pts',(-15.6795425955901,13.147124558532,0.));
#14312=CARTESIAN_POINT('Ctrl Pts',(-15.6795425955901,13.147124558532,21.));
#14313=CARTESIAN_POINT('Ctrl Pts',(-15.7273402954914,13.161288914421,0.));
#14314=CARTESIAN_POINT('Ctrl Pts',(-15.7273402954914,13.161288914421,21.));
#14315=CARTESIAN_POINT('Ctrl Pts',(-15.7752961549278,13.1751853728467,0.));
#14316=CARTESIAN_POINT('Ctrl Pts',(-15.7752961549278,13.1751853728467,21.));
#14317=CARTESIAN_POINT('Ctrl Pts',(-15.8234081427091,13.1888152101588,0.));
#14318=CARTESIAN_POINT('Ctrl Pts',(-15.8234081427091,13.1888152101588,21.));
#14319=CARTESIAN_POINT('Ctrl Pts',(-15.8716743375555,13.2021795724682,0.));
#14320=CARTESIAN_POINT('Ctrl Pts',(-15.8716743375555,13.2021795724682,21.));
#14321=CARTESIAN_POINT('Ctrl Pts',(-15.9200926550954,13.2152798388134,0.));
#14322=CARTESIAN_POINT('Ctrl Pts',(-15.9200926550954,13.2152798388134,21.));
#14323=CARTESIAN_POINT('Ctrl Pts',(-15.9686607385389,13.2281177675127,0.));
#14324=CARTESIAN_POINT('Ctrl Pts',(-15.9686607385389,13.2281177675127,21.));
#14325=CARTESIAN_POINT('Ctrl Pts',(-16.0173761036734,13.240695304984,0.));
#14326=CARTESIAN_POINT('Ctrl Pts',(-16.0173761036734,13.240695304984,21.));
#14327=CARTESIAN_POINT('Ctrl Pts',(-16.0662362238032,13.2530144750236,0.));
#14328=CARTESIAN_POINT('Ctrl Pts',(-16.0662362238032,13.2530144750236,21.));
#14329=CARTESIAN_POINT('Ctrl Pts',(-16.1152386305152,13.2650772466062,0.));
#14330=CARTESIAN_POINT('Ctrl Pts',(-16.1152386305152,13.2650772466062,21.));
#14331=CARTESIAN_POINT('Ctrl Pts',(-16.1643810242643,13.2768853909882,0.));
#14332=CARTESIAN_POINT('Ctrl Pts',(-16.1643810242643,13.2768853909882,21.));
#14333=CARTESIAN_POINT('Ctrl Pts',(-16.2136613184475,13.2884404210388,0.));
#14334=CARTESIAN_POINT('Ctrl Pts',(-16.2136613184475,13.2884404210388,21.));
#14335=CARTESIAN_POINT('Ctrl Pts',(-16.2630775678735,13.2997436744733,0.));
#14336=CARTESIAN_POINT('Ctrl Pts',(-16.2630775678735,13.2997436744733,21.));
#14337=CARTESIAN_POINT('Ctrl Pts',(-16.3126279218067,13.3107963665229,0.));
#14338=CARTESIAN_POINT('Ctrl Pts',(-16.3126279218067,13.3107963665229,21.));
#14339=CARTESIAN_POINT('Ctrl Pts',(-16.3623105703343,13.3215996524974,0.));
#14340=CARTESIAN_POINT('Ctrl Pts',(-16.3623105703343,13.3215996524974,21.));
#14341=CARTESIAN_POINT('Ctrl Pts',(-16.4121236828756,13.3321546976812,0.));
#14342=CARTESIAN_POINT('Ctrl Pts',(-16.4121236828756,13.3321546976812,21.));
#14343=CARTESIAN_POINT('Ctrl Pts',(-16.4620653818862,13.3424627129921,0.));
#14344=CARTESIAN_POINT('Ctrl Pts',(-16.4620653818862,13.3424627129921,21.));
#14345=CARTESIAN_POINT('Ctrl Pts',(-16.5121337902953,13.3525249163084,0.));
#14346=CARTESIAN_POINT('Ctrl Pts',(-16.5121337902953,13.3525249163084,21.));
#14347=CARTESIAN_POINT('Ctrl Pts',(-16.5623270636327,13.3623425108873,0.));
#14348=CARTESIAN_POINT('Ctrl Pts',(-16.5623270636327,13.3623425108873,21.));
#14349=CARTESIAN_POINT('Ctrl Pts',(-16.612643424234,13.3719166600676,0.));
#14350=CARTESIAN_POINT('Ctrl Pts',(-16.612643424234,13.3719166600676,21.));
#14351=CARTESIAN_POINT('Ctrl Pts',(-16.6630812012276,13.381248462113,0.));
#14352=CARTESIAN_POINT('Ctrl Pts',(-16.6630812012276,13.381248462113,21.));
#14353=CARTESIAN_POINT('Ctrl Pts',(-16.7136388432444,13.3903389370346,0.));
#14354=CARTESIAN_POINT('Ctrl Pts',(-16.7136388432444,13.3903389370346,21.));
#14355=CARTESIAN_POINT('Ctrl Pts',(-16.7643148579872,13.3991890464165,0.));
#14356=CARTESIAN_POINT('Ctrl Pts',(-16.7643148579872,13.3991890464165,21.));
#14357=CARTESIAN_POINT('Ctrl Pts',(-16.8151077630226,13.4077997088426,0.));
#14358=CARTESIAN_POINT('Ctrl Pts',(-16.8151077630226,13.4077997088426,21.));
#14359=CARTESIAN_POINT('Ctrl Pts',(-16.8660160353187,13.4161718177499,0.));
#14360=CARTESIAN_POINT('Ctrl Pts',(-16.8660160353187,13.4161718177499,21.));
#14361=CARTESIAN_POINT('Ctrl Pts',(-16.9170380509036,13.4243062623592,0.));
#14362=CARTESIAN_POINT('Ctrl Pts',(-16.9170380509036,13.4243062623592,21.));
#14363=CARTESIAN_POINT('Ctrl Pts',(-16.9681720567298,13.432203941793,0.));
#14364=CARTESIAN_POINT('Ctrl Pts',(-16.9681720567298,13.432203941793,21.));
#14365=CARTESIAN_POINT('Ctrl Pts',(-17.0194162803447,13.4398657451291,0.));
#14366=CARTESIAN_POINT('Ctrl Pts',(-17.0194162803447,13.4398657451291,21.));
#14367=CARTESIAN_POINT('Ctrl Pts',(-17.0707690194411,13.4472925380889,0.));
#14368=CARTESIAN_POINT('Ctrl Pts',(-17.0707690194411,13.4472925380889,21.));
#14369=CARTESIAN_POINT('Ctrl Pts',(-17.1222287365697,13.4544851484583,0.));
#14370=CARTESIAN_POINT('Ctrl Pts',(-17.1222287365697,13.4544851484583,21.));
#14371=CARTESIAN_POINT('Ctrl Pts',(-17.1737941556239,13.4614443545811,0.));
#14372=CARTESIAN_POINT('Ctrl Pts',(-17.1737941556239,13.4614443545811,21.));
#14373=CARTESIAN_POINT('Ctrl Pts',(-17.2254643437923,13.4681708717969,0.));
#14374=CARTESIAN_POINT('Ctrl Pts',(-17.2254643437923,13.4681708717969,21.));
#14375=CARTESIAN_POINT('Ctrl Pts',(-17.2772386565028,13.474665315482,0.));
#14376=CARTESIAN_POINT('Ctrl Pts',(-17.2772386565028,13.474665315482,21.));
#14377=CARTESIAN_POINT('Ctrl Pts',(-17.3187410868027,13.4796755969465,0.));
#14378=CARTESIAN_POINT('Ctrl Pts',(-17.3187410868027,13.4796755969465,21.));
#14379=CARTESIAN_POINT('Ctrl Pts',(-17.3499144948292,13.4833292332349,0.));
#14380=CARTESIAN_POINT('Ctrl Pts',(-17.3499144948292,13.4833292332349,21.));
#14381=CARTESIAN_POINT('Ctrl Pts',(-17.3707174645609,13.485718750657,0.));
#14382=CARTESIAN_POINT('Ctrl Pts',(-17.3707174645609,13.485718750657,21.));
#14383=CARTESIAN_POINT('Ctrl Pts',(-17.3811241238545,13.4869019493419,0.));
#14384=CARTESIAN_POINT('Ctrl Pts',(-17.3811241238545,13.4869019493419,21.));
#14385=CARTESIAN_POINT('Ctrl Pts',(-14.1074595503134,12.4172651441477,0.));
#14386=CARTESIAN_POINT('Ctrl Pts',(-14.1145347042316,12.4234926340671,0.));
#14387=CARTESIAN_POINT('Ctrl Pts',(-14.1288394445866,12.4357509724316,0.));
#14388=CARTESIAN_POINT('Ctrl Pts',(-14.1507598477672,12.4535485619996,0.));
#14389=CARTESIAN_POINT('Ctrl Pts',(-14.1808688343892,12.4761570639125,0.));
#14390=CARTESIAN_POINT('Ctrl Pts',(-14.2197144660135,12.5028859651751,0.));
#14391=CARTESIAN_POINT('Ctrl Pts',(-14.2594378207584,12.5285125321527,0.));
#14392=CARTESIAN_POINT('Ctrl Pts',(-14.2997103098726,12.5534605602317,0.));
#14393=CARTESIAN_POINT('Ctrl Pts',(-14.3402859058353,12.5780443898087,0.));
#14394=CARTESIAN_POINT('Ctrl Pts',(-14.3810669346235,12.6023830189244,0.));
#14395=CARTESIAN_POINT('Ctrl Pts',(-14.4220553460485,12.626464614311,0.));
#14396=CARTESIAN_POINT('Ctrl Pts',(-14.463313553928,12.6501984687124,0.));
#14397=CARTESIAN_POINT('Ctrl Pts',(-14.5049233087958,12.6734695081852,0.));
#14398=CARTESIAN_POINT('Ctrl Pts',(-14.5469417071951,12.6961966430455,0.));
#14399=CARTESIAN_POINT('Ctrl Pts',(-14.5893698147583,12.7183743139638,0.));
#14400=CARTESIAN_POINT('Ctrl Pts',(-14.6321748083434,12.7400427996251,0.));
#14401=CARTESIAN_POINT('Ctrl Pts',(-14.6753044633399,12.7612687078867,0.));
#14402=CARTESIAN_POINT('Ctrl Pts',(-14.7187037124277,12.7821227233337,0.));
#14403=CARTESIAN_POINT('Ctrl Pts',(-14.7623324139791,12.8026557145457,0.));
#14404=CARTESIAN_POINT('Ctrl Pts',(-14.8061758577898,12.8228846016791,0.));
#14405=CARTESIAN_POINT('Ctrl Pts',(-14.8502347891476,12.8428057266944,0.));
#14406=CARTESIAN_POINT('Ctrl Pts',(-14.8945191569251,12.8624032236317,0.));
#14407=CARTESIAN_POINT('Ctrl Pts',(-14.9390408507356,12.8816587472147,0.));
#14408=CARTESIAN_POINT('Ctrl Pts',(-14.9838057866976,12.9005620742036,0.));
#14409=CARTESIAN_POINT('Ctrl Pts',(-15.0288099208306,12.9191164383568,0.));
#14410=CARTESIAN_POINT('Ctrl Pts',(-15.0740435169624,12.9373327960422,0.));
#14411=CARTESIAN_POINT('Ctrl Pts',(-15.1194937003528,12.9552263908864,0.));
#14412=CARTESIAN_POINT('Ctrl Pts',(-15.1651474813659,12.9728126886697,0.));
#14413=CARTESIAN_POINT('Ctrl Pts',(-15.2109950816083,12.9901029059182,0.));
#14414=CARTESIAN_POINT('Ctrl Pts',(-15.2570313635503,13.0071020851025,0.));
#14415=CARTESIAN_POINT('Ctrl Pts',(-15.3032539741328,13.0238115816728,0.));
#14416=CARTESIAN_POINT('Ctrl Pts',(-15.3496622219036,13.0402305665115,0.));
#14417=CARTESIAN_POINT('Ctrl Pts',(-15.3962557545684,13.0563577967298,0.));
#14418=CARTESIAN_POINT('Ctrl Pts',(-15.4430330918328,13.0721935806302,0.));
#14419=CARTESIAN_POINT('Ctrl Pts',(-15.4899910401523,13.087740560189,0.));
#14420=CARTESIAN_POINT('Ctrl Pts',(-15.5371254712111,13.1030026646917,0.));
#14421=CARTESIAN_POINT('Ctrl Pts',(-15.5844317820184,13.1179844917497,0.));
#14422=CARTESIAN_POINT('Ctrl Pts',(-15.6319054413079,13.1326905726717,0.));
#14423=CARTESIAN_POINT('Ctrl Pts',(-15.6795425955901,13.147124558532,0.));
#14424=CARTESIAN_POINT('Ctrl Pts',(-15.7273402954914,13.161288914421,0.));
#14425=CARTESIAN_POINT('Ctrl Pts',(-15.7752961549278,13.1751853728467,0.));
#14426=CARTESIAN_POINT('Ctrl Pts',(-15.8234081427091,13.1888152101588,0.));
#14427=CARTESIAN_POINT('Ctrl Pts',(-15.8716743375555,13.2021795724682,0.));
#14428=CARTESIAN_POINT('Ctrl Pts',(-15.9200926550954,13.2152798388134,0.));
#14429=CARTESIAN_POINT('Ctrl Pts',(-15.9686607385389,13.2281177675127,0.));
#14430=CARTESIAN_POINT('Ctrl Pts',(-16.0173761036734,13.240695304984,0.));
#14431=CARTESIAN_POINT('Ctrl Pts',(-16.0662362238032,13.2530144750236,0.));
#14432=CARTESIAN_POINT('Ctrl Pts',(-16.1152386305152,13.2650772466062,0.));
#14433=CARTESIAN_POINT('Ctrl Pts',(-16.1643810242643,13.2768853909882,0.));
#14434=CARTESIAN_POINT('Ctrl Pts',(-16.2136613184475,13.2884404210388,0.));
#14435=CARTESIAN_POINT('Ctrl Pts',(-16.2630775678735,13.2997436744733,0.));
#14436=CARTESIAN_POINT('Ctrl Pts',(-16.3126279218067,13.3107963665229,0.));
#14437=CARTESIAN_POINT('Ctrl Pts',(-16.3623105703343,13.3215996524974,0.));
#14438=CARTESIAN_POINT('Ctrl Pts',(-16.4121236828756,13.3321546976812,0.));
#14439=CARTESIAN_POINT('Ctrl Pts',(-16.4620653818862,13.3424627129921,0.));
#14440=CARTESIAN_POINT('Ctrl Pts',(-16.5121337902953,13.3525249163084,0.));
#14441=CARTESIAN_POINT('Ctrl Pts',(-16.5623270636327,13.3623425108873,0.));
#14442=CARTESIAN_POINT('Ctrl Pts',(-16.612643424234,13.3719166600676,0.));
#14443=CARTESIAN_POINT('Ctrl Pts',(-16.6630812012276,13.381248462113,0.));
#14444=CARTESIAN_POINT('Ctrl Pts',(-16.7136388432444,13.3903389370346,0.));
#14445=CARTESIAN_POINT('Ctrl Pts',(-16.7643148579872,13.3991890464165,0.));
#14446=CARTESIAN_POINT('Ctrl Pts',(-16.8151077630226,13.4077997088426,0.));
#14447=CARTESIAN_POINT('Ctrl Pts',(-16.8660160353187,13.4161718177499,0.));
#14448=CARTESIAN_POINT('Ctrl Pts',(-16.9170380509036,13.4243062623592,0.));
#14449=CARTESIAN_POINT('Ctrl Pts',(-16.9681720567298,13.432203941793,0.));
#14450=CARTESIAN_POINT('Ctrl Pts',(-17.0194162803447,13.4398657451291,0.));
#14451=CARTESIAN_POINT('Ctrl Pts',(-17.0707690194411,13.4472925380889,0.));
#14452=CARTESIAN_POINT('Ctrl Pts',(-17.1222287365697,13.4544851484583,0.));
#14453=CARTESIAN_POINT('Ctrl Pts',(-17.1737941556239,13.4614443545811,0.));
#14454=CARTESIAN_POINT('Ctrl Pts',(-17.235798381426,13.4695161752401,0.));
#14455=CARTESIAN_POINT('Ctrl Pts',(-17.287598725272,13.4759526005425,0.));
#14456=CARTESIAN_POINT('Ctrl Pts',(-17.3291218739796,13.4809165957478,0.));
#14457=CARTESIAN_POINT('Ctrl Pts',(-17.360310805254,13.4845355519784,0.));
#14458=CARTESIAN_POINT('Ctrl Pts',(-17.3811241238545,13.4869019493419,0.));
#14459=CARTESIAN_POINT('Ctrl Pts',(-14.1074595503134,12.4172651441477,13.));
#14460=CARTESIAN_POINT('Ctrl Pts',(-14.1193844248164,12.4277613166149,13.));
#14461=CARTESIAN_POINT('Ctrl Pts',(-14.1315753314249,12.4379186757848,13.));
#14462=CARTESIAN_POINT('Ctrl Pts',(-14.14401474732,12.4477599775084,13.));
#14463=CARTESIAN_POINT('Ctrl Pts',(-14.1585946731696,12.45929471922,13.));
#14464=CARTESIAN_POINT('Ctrl Pts',(-14.1735154808295,12.4703959522577,13.));
#14465=CARTESIAN_POINT('Ctrl Pts',(-14.1887053040703,12.4811568677436,13.));
#14466=CARTESIAN_POINT('Ctrl Pts',(-14.2100781123335,12.4962979908344,13.));
#14467=CARTESIAN_POINT('Ctrl Pts',(-14.2319791941756,12.5107710847127,13.));
#14468=CARTESIAN_POINT('Ctrl Pts',(-14.254157574695,12.5249003586941,13.));
#14469=CARTESIAN_POINT('Ctrl Pts',(-14.2689096955178,12.5342985542355,13.));
#14470=CARTESIAN_POINT('Ctrl Pts',(-14.2837832480516,12.5435462296413,13.));
#14471=CARTESIAN_POINT('Ctrl Pts',(-14.298722508524,12.5527146050322,13.));
#14472=CARTESIAN_POINT('Ctrl Pts',(-14.3144485290642,12.5623658230416,13.));
#14473=CARTESIAN_POINT('Ctrl Pts',(-14.330246820686,12.5719298675028,13.));
#14474=CARTESIAN_POINT('Ctrl Pts',(-14.3460912752807,12.5814385821519,13.));
#14475=CARTESIAN_POINT('Ctrl Pts',(-14.3636874094394,12.5919985302804,13.));
#14476=CARTESIAN_POINT('Ctrl Pts',(-14.381341260665,12.6024891912727,13.));
#14477=CARTESIAN_POINT('Ctrl Pts',(-14.3990589912032,12.6128991700701,13.));
#14478=CARTESIAN_POINT('Ctrl Pts',(-14.4257693299403,12.6285927183677,13.));
#14479=CARTESIAN_POINT('Ctrl Pts',(-14.452628589856,12.6440977931351,13.));
#14480=CARTESIAN_POINT('Ctrl Pts',(-14.4797266308813,12.6592867998067,13.));
#14481=CARTESIAN_POINT('Ctrl Pts',(-14.4994127652612,12.6703212810873,13.));
#14482=CARTESIAN_POINT('Ctrl Pts',(-14.5192269386383,12.6811863451307,13.));
#14483=CARTESIAN_POINT('Ctrl Pts',(-14.5391805041508,12.6918647171384,13.));
#14484=CARTESIAN_POINT('Ctrl Pts',(-14.5635720293892,12.7049181125412,13.));
#14485=CARTESIAN_POINT('Ctrl Pts',(-14.5881710816651,12.7176935524276,13.));
#14486=CARTESIAN_POINT('Ctrl Pts',(-14.612947560673,12.7302281821981,13.));
#14487=CARTESIAN_POINT('Ctrl Pts',(-14.6397102700639,12.7437676626773,13.));
#14488=CARTESIAN_POINT('Ctrl Pts',(-14.6666764215902,12.7570309720221,13.));
#14489=CARTESIAN_POINT('Ctrl Pts',(-14.6937895363403,12.7700903554915,13.));
#14490=CARTESIAN_POINT('Ctrl Pts',(-14.7188202365146,12.7821467169645,13.));
#14491=CARTESIAN_POINT('Ctrl Pts',(-14.7439746960234,12.7940312932614,13.));
#14492=CARTESIAN_POINT('Ctrl Pts',(-14.7692347187417,12.8057660290113,13.));
#14493=CARTESIAN_POINT('Ctrl Pts',(-14.803551756556,12.8217082700361,13.));
#14494=CARTESIAN_POINT('Ctrl Pts',(-14.8380647951195,12.8373723698026,13.));
#14495=CARTESIAN_POINT('Ctrl Pts',(-14.8727890594695,12.8527323828632,13.));
#14496=CARTESIAN_POINT('Ctrl Pts',(-14.9062972246235,12.8675544637349,13.));
#14497=CARTESIAN_POINT('Ctrl Pts',(-14.9400067536049,12.8820871276608,13.));
#14498=CARTESIAN_POINT('Ctrl Pts',(-14.9739251233868,12.8963159096104,13.));
#14499=CARTESIAN_POINT('Ctrl Pts',(-15.0200041787641,12.9156461084266,13.));
#14500=CARTESIAN_POINT('Ctrl Pts',(-15.0664667162746,12.9344180544673,13.));
#14501=CARTESIAN_POINT('Ctrl Pts',(-15.1132567586771,12.9526968521306,13.));
#14502=CARTESIAN_POINT('Ctrl Pts',(-15.1543841890161,12.968763518006,13.));
#14503=CARTESIAN_POINT('Ctrl Pts',(-15.195760575808,12.9844546719519,13.));
#14504=CARTESIAN_POINT('Ctrl Pts',(-15.2373637638391,12.9997938464524,13.));
#14505=CARTESIAN_POINT('Ctrl Pts',(-15.298696963875,13.0224075138791,13.));
#14506=CARTESIAN_POINT('Ctrl Pts',(-15.3605284720727,13.0442489122199,13.));
#14507=CARTESIAN_POINT('Ctrl Pts',(-15.4228468913963,13.0653151028182,13.));
#14508=CARTESIAN_POINT('Ctrl Pts',(-15.501493344391,13.0919008408175,13.));
#14509=CARTESIAN_POINT('Ctrl Pts',(-15.580912148319,13.1172560779889,13.));
#14510=CARTESIAN_POINT('Ctrl Pts',(-15.6610132193903,13.1414683121723,13.));
#14511=CARTESIAN_POINT('Ctrl Pts',(-15.7695162957074,13.1742656500639,13.));
#14512=CARTESIAN_POINT('Ctrl Pts',(-15.8792747460898,13.2049609859192,13.));
#14513=CARTESIAN_POINT('Ctrl Pts',(-15.9901726544041,13.2336341230354,13.));
#14514=CARTESIAN_POINT('Ctrl Pts',(-16.089041043312,13.2591969755247,13.));
#14515=CARTESIAN_POINT('Ctrl Pts',(-16.1888100042035,13.2831593506295,13.));
#14516=CARTESIAN_POINT('Ctrl Pts',(-16.2893994149303,13.305579935219,13.));
#14517=CARTESIAN_POINT('Ctrl Pts',(-16.4319622721867,13.3373560692807,13.));
#14518=CARTESIAN_POINT('Ctrl Pts',(-16.5761757269041,13.3660302366011,13.));
#14519=CARTESIAN_POINT('Ctrl Pts',(-16.7218506225541,13.3917254924233,13.));
#14520=CARTESIAN_POINT('Ctrl Pts',(-16.8350074321741,13.4116849587284,13.));
#14521=CARTESIAN_POINT('Ctrl Pts',(-16.9490507104974,13.4298451938425,13.));
#14522=CARTESIAN_POINT('Ctrl Pts',(-17.063896781128,13.4462507334689,13.));
#14523=CARTESIAN_POINT('Ctrl Pts',(-17.1632473211086,13.4604427664362,13.));
#14524=CARTESIAN_POINT('Ctrl Pts',(-17.2631945741556,13.4733230167208,13.));
#14525=CARTESIAN_POINT('Ctrl Pts',(-17.363718437608,13.4849093843288,13.));
#14526=CARTESIAN_POINT('Ctrl Pts',(-17.3695184016672,13.4855778874423,13.));
#14527=CARTESIAN_POINT('Ctrl Pts',(-17.3753202971203,13.4862420757008,13.));
#14528=CARTESIAN_POINT('Ctrl Pts',(-17.3811241238545,13.4869019493419,13.));
#14529=CARTESIAN_POINT('Ctrl Pts',(-13.4869019493419,17.3811241238545,0.));
#14530=CARTESIAN_POINT('Ctrl Pts',(-13.4869019493419,17.3811241238545,21.));
#14531=CARTESIAN_POINT('Ctrl Pts',(-13.485718750657,17.3707174645609,0.));
#14532=CARTESIAN_POINT('Ctrl Pts',(-13.485718750657,17.3707174645609,21.));
#14533=CARTESIAN_POINT('Ctrl Pts',(-13.4833292332349,17.3499144948292,0.));
#14534=CARTESIAN_POINT('Ctrl Pts',(-13.4833292332349,17.3499144948292,21.));
#14535=CARTESIAN_POINT('Ctrl Pts',(-13.4796755969465,17.3187410868027,0.));
#14536=CARTESIAN_POINT('Ctrl Pts',(-13.4796755969465,17.3187410868027,21.));
#14537=CARTESIAN_POINT('Ctrl Pts',(-13.474665315482,17.2772386565028,0.));
#14538=CARTESIAN_POINT('Ctrl Pts',(-13.474665315482,17.2772386565028,21.));
#14539=CARTESIAN_POINT('Ctrl Pts',(-13.4681708717969,17.2254643437923,0.));
#14540=CARTESIAN_POINT('Ctrl Pts',(-13.4681708717969,17.2254643437923,21.));
#14541=CARTESIAN_POINT('Ctrl Pts',(-13.4614443545811,17.173794155624,0.));
#14542=CARTESIAN_POINT('Ctrl Pts',(-13.4614443545811,17.173794155624,21.));
#14543=CARTESIAN_POINT('Ctrl Pts',(-13.4544851484583,17.1222287365697,0.));
#14544=CARTESIAN_POINT('Ctrl Pts',(-13.4544851484583,17.1222287365697,21.));
#14545=CARTESIAN_POINT('Ctrl Pts',(-13.4472925380889,17.0707690194412,0.));
#14546=CARTESIAN_POINT('Ctrl Pts',(-13.4472925380889,17.0707690194412,21.));
#14547=CARTESIAN_POINT('Ctrl Pts',(-13.4398657451291,17.0194162803447,0.));
#14548=CARTESIAN_POINT('Ctrl Pts',(-13.4398657451291,17.0194162803447,21.));
#14549=CARTESIAN_POINT('Ctrl Pts',(-13.432203941793,16.9681720567298,0.));
#14550=CARTESIAN_POINT('Ctrl Pts',(-13.432203941793,16.9681720567298,21.));
#14551=CARTESIAN_POINT('Ctrl Pts',(-13.4243062623592,16.9170380509036,0.));
#14552=CARTESIAN_POINT('Ctrl Pts',(-13.4243062623592,16.9170380509036,21.));
#14553=CARTESIAN_POINT('Ctrl Pts',(-13.4161718177499,16.8660160353187,0.));
#14554=CARTESIAN_POINT('Ctrl Pts',(-13.4161718177499,16.8660160353187,21.));
#14555=CARTESIAN_POINT('Ctrl Pts',(-13.4077997088426,16.8151077630226,0.));
#14556=CARTESIAN_POINT('Ctrl Pts',(-13.4077997088426,16.8151077630226,21.));
#14557=CARTESIAN_POINT('Ctrl Pts',(-13.3991890464165,16.7643148579873,0.));
#14558=CARTESIAN_POINT('Ctrl Pts',(-13.3991890464165,16.7643148579873,21.));
#14559=CARTESIAN_POINT('Ctrl Pts',(-13.3903389370346,16.7136388432444,0.));
#14560=CARTESIAN_POINT('Ctrl Pts',(-13.3903389370346,16.7136388432444,21.));
#14561=CARTESIAN_POINT('Ctrl Pts',(-13.381248462113,16.6630812012276,0.));
#14562=CARTESIAN_POINT('Ctrl Pts',(-13.381248462113,16.6630812012276,21.));
#14563=CARTESIAN_POINT('Ctrl Pts',(-13.3719166600676,16.612643424234,0.));
#14564=CARTESIAN_POINT('Ctrl Pts',(-13.3719166600676,16.612643424234,21.));
#14565=CARTESIAN_POINT('Ctrl Pts',(-13.3623425108873,16.5623270636327,0.));
#14566=CARTESIAN_POINT('Ctrl Pts',(-13.3623425108873,16.5623270636327,21.));
#14567=CARTESIAN_POINT('Ctrl Pts',(-13.3525249163084,16.5121337902953,0.));
#14568=CARTESIAN_POINT('Ctrl Pts',(-13.3525249163084,16.5121337902953,21.));
#14569=CARTESIAN_POINT('Ctrl Pts',(-13.3424627129921,16.4620653818862,0.));
#14570=CARTESIAN_POINT('Ctrl Pts',(-13.3424627129921,16.4620653818862,21.));
#14571=CARTESIAN_POINT('Ctrl Pts',(-13.3321546976812,16.4121236828756,0.));
#14572=CARTESIAN_POINT('Ctrl Pts',(-13.3321546976812,16.4121236828756,21.));
#14573=CARTESIAN_POINT('Ctrl Pts',(-13.3215996524974,16.3623105703343,0.));
#14574=CARTESIAN_POINT('Ctrl Pts',(-13.3215996524974,16.3623105703343,21.));
#14575=CARTESIAN_POINT('Ctrl Pts',(-13.3107963665229,16.3126279218067,0.));
#14576=CARTESIAN_POINT('Ctrl Pts',(-13.3107963665229,16.3126279218067,21.));
#14577=CARTESIAN_POINT('Ctrl Pts',(-13.2997436744733,16.2630775678735,0.));
#14578=CARTESIAN_POINT('Ctrl Pts',(-13.2997436744733,16.2630775678735,21.));
#14579=CARTESIAN_POINT('Ctrl Pts',(-13.2884404210387,16.2136613184475,0.));
#14580=CARTESIAN_POINT('Ctrl Pts',(-13.2884404210387,16.2136613184475,21.));
#14581=CARTESIAN_POINT('Ctrl Pts',(-13.2768853909882,16.1643810242643,0.));
#14582=CARTESIAN_POINT('Ctrl Pts',(-13.2768853909882,16.1643810242643,21.));
#14583=CARTESIAN_POINT('Ctrl Pts',(-13.2650772466062,16.1152386305152,0.));
#14584=CARTESIAN_POINT('Ctrl Pts',(-13.2650772466062,16.1152386305152,21.));
#14585=CARTESIAN_POINT('Ctrl Pts',(-13.2530144750236,16.0662362238032,0.));
#14586=CARTESIAN_POINT('Ctrl Pts',(-13.2530144750236,16.0662362238032,21.));
#14587=CARTESIAN_POINT('Ctrl Pts',(-13.240695304984,16.0173761036734,0.));
#14588=CARTESIAN_POINT('Ctrl Pts',(-13.240695304984,16.0173761036734,21.));
#14589=CARTESIAN_POINT('Ctrl Pts',(-13.2281177675127,15.9686607385389,0.));
#14590=CARTESIAN_POINT('Ctrl Pts',(-13.2281177675127,15.9686607385389,21.));
#14591=CARTESIAN_POINT('Ctrl Pts',(-13.2152798388134,15.9200926550954,0.));
#14592=CARTESIAN_POINT('Ctrl Pts',(-13.2152798388134,15.9200926550954,21.));
#14593=CARTESIAN_POINT('Ctrl Pts',(-13.2021795724682,15.8716743375555,0.));
#14594=CARTESIAN_POINT('Ctrl Pts',(-13.2021795724682,15.8716743375555,21.));
#14595=CARTESIAN_POINT('Ctrl Pts',(-13.1888152101588,15.8234081427091,0.));
#14596=CARTESIAN_POINT('Ctrl Pts',(-13.1888152101588,15.8234081427091,21.));
#14597=CARTESIAN_POINT('Ctrl Pts',(-13.1751853728467,15.7752961549278,0.));
#14598=CARTESIAN_POINT('Ctrl Pts',(-13.1751853728467,15.7752961549278,21.));
#14599=CARTESIAN_POINT('Ctrl Pts',(-13.161288914421,15.7273402954914,0.));
#14600=CARTESIAN_POINT('Ctrl Pts',(-13.161288914421,15.7273402954914,21.));
#14601=CARTESIAN_POINT('Ctrl Pts',(-13.147124558532,15.6795425955901,0.));
#14602=CARTESIAN_POINT('Ctrl Pts',(-13.147124558532,15.6795425955901,21.));
#14603=CARTESIAN_POINT('Ctrl Pts',(-13.1326905726717,15.6319054413079,0.));
#14604=CARTESIAN_POINT('Ctrl Pts',(-13.1326905726717,15.6319054413079,21.));
#14605=CARTESIAN_POINT('Ctrl Pts',(-13.1179844917497,15.5844317820184,0.));
#14606=CARTESIAN_POINT('Ctrl Pts',(-13.1179844917497,15.5844317820184,21.));
#14607=CARTESIAN_POINT('Ctrl Pts',(-13.1030026646917,15.5371254712111,0.));
#14608=CARTESIAN_POINT('Ctrl Pts',(-13.1030026646917,15.5371254712111,21.));
#14609=CARTESIAN_POINT('Ctrl Pts',(-13.087740560189,15.4899910401523,0.));
#14610=CARTESIAN_POINT('Ctrl Pts',(-13.087740560189,15.4899910401523,21.));
#14611=CARTESIAN_POINT('Ctrl Pts',(-13.0721935806302,15.4430330918328,0.));
#14612=CARTESIAN_POINT('Ctrl Pts',(-13.0721935806302,15.4430330918328,21.));
#14613=CARTESIAN_POINT('Ctrl Pts',(-13.0563577967298,15.3962557545684,0.));
#14614=CARTESIAN_POINT('Ctrl Pts',(-13.0563577967298,15.3962557545684,21.));
#14615=CARTESIAN_POINT('Ctrl Pts',(-13.0402305665115,15.3496622219036,0.));
#14616=CARTESIAN_POINT('Ctrl Pts',(-13.0402305665115,15.3496622219036,21.));
#14617=CARTESIAN_POINT('Ctrl Pts',(-13.0238115816728,15.3032539741328,0.));
#14618=CARTESIAN_POINT('Ctrl Pts',(-13.0238115816728,15.3032539741328,21.));
#14619=CARTESIAN_POINT('Ctrl Pts',(-13.0071020851025,15.2570313635503,0.));
#14620=CARTESIAN_POINT('Ctrl Pts',(-13.0071020851025,15.2570313635503,21.));
#14621=CARTESIAN_POINT('Ctrl Pts',(-12.9901029059182,15.2109950816083,0.));
#14622=CARTESIAN_POINT('Ctrl Pts',(-12.9901029059182,15.2109950816083,21.));
#14623=CARTESIAN_POINT('Ctrl Pts',(-12.9728126886697,15.1651474813659,0.));
#14624=CARTESIAN_POINT('Ctrl Pts',(-12.9728126886697,15.1651474813659,21.));
#14625=CARTESIAN_POINT('Ctrl Pts',(-12.9552263908864,15.1194937003528,0.));
#14626=CARTESIAN_POINT('Ctrl Pts',(-12.9552263908864,15.1194937003528,21.));
#14627=CARTESIAN_POINT('Ctrl Pts',(-12.9373327960422,15.0740435169624,0.));
#14628=CARTESIAN_POINT('Ctrl Pts',(-12.9373327960422,15.0740435169624,21.));
#14629=CARTESIAN_POINT('Ctrl Pts',(-12.9191164383568,15.0288099208306,0.));
#14630=CARTESIAN_POINT('Ctrl Pts',(-12.9191164383568,15.0288099208306,21.));
#14631=CARTESIAN_POINT('Ctrl Pts',(-12.9005620742036,14.9838057866976,0.));
#14632=CARTESIAN_POINT('Ctrl Pts',(-12.9005620742036,14.9838057866976,21.));
#14633=CARTESIAN_POINT('Ctrl Pts',(-12.8816587472147,14.9390408507356,0.));
#14634=CARTESIAN_POINT('Ctrl Pts',(-12.8816587472147,14.9390408507356,21.));
#14635=CARTESIAN_POINT('Ctrl Pts',(-12.8624032236317,14.8945191569251,0.));
#14636=CARTESIAN_POINT('Ctrl Pts',(-12.8624032236317,14.8945191569251,21.));
#14637=CARTESIAN_POINT('Ctrl Pts',(-12.8428057266944,14.8502347891476,0.));
#14638=CARTESIAN_POINT('Ctrl Pts',(-12.8428057266944,14.8502347891476,21.));
#14639=CARTESIAN_POINT('Ctrl Pts',(-12.8228846016791,14.8061758577898,0.));
#14640=CARTESIAN_POINT('Ctrl Pts',(-12.8228846016791,14.8061758577898,21.));
#14641=CARTESIAN_POINT('Ctrl Pts',(-12.8026557145457,14.7623324139791,0.));
#14642=CARTESIAN_POINT('Ctrl Pts',(-12.8026557145457,14.7623324139791,21.));
#14643=CARTESIAN_POINT('Ctrl Pts',(-12.7821227233337,14.7187037124277,0.));
#14644=CARTESIAN_POINT('Ctrl Pts',(-12.7821227233337,14.7187037124277,21.));
#14645=CARTESIAN_POINT('Ctrl Pts',(-12.7612687078867,14.6753044633399,0.));
#14646=CARTESIAN_POINT('Ctrl Pts',(-12.7612687078867,14.6753044633399,21.));
#14647=CARTESIAN_POINT('Ctrl Pts',(-12.7400427996251,14.6321748083434,0.));
#14648=CARTESIAN_POINT('Ctrl Pts',(-12.7400427996251,14.6321748083434,21.));
#14649=CARTESIAN_POINT('Ctrl Pts',(-12.7183743139638,14.5893698147583,0.));
#14650=CARTESIAN_POINT('Ctrl Pts',(-12.7183743139638,14.5893698147583,21.));
#14651=CARTESIAN_POINT('Ctrl Pts',(-12.6961966430455,14.5469417071952,0.));
#14652=CARTESIAN_POINT('Ctrl Pts',(-12.6961966430455,14.5469417071952,21.));
#14653=CARTESIAN_POINT('Ctrl Pts',(-12.6734695081852,14.5049233087958,0.));
#14654=CARTESIAN_POINT('Ctrl Pts',(-12.6734695081852,14.5049233087958,21.));
#14655=CARTESIAN_POINT('Ctrl Pts',(-12.6501984687124,14.463313553928,0.));
#14656=CARTESIAN_POINT('Ctrl Pts',(-12.6501984687124,14.463313553928,21.));
#14657=CARTESIAN_POINT('Ctrl Pts',(-12.626464614311,14.4220553460485,0.));
#14658=CARTESIAN_POINT('Ctrl Pts',(-12.626464614311,14.4220553460485,21.));
#14659=CARTESIAN_POINT('Ctrl Pts',(-12.6023830189244,14.3810669346235,0.));
#14660=CARTESIAN_POINT('Ctrl Pts',(-12.6023830189244,14.3810669346235,21.));
#14661=CARTESIAN_POINT('Ctrl Pts',(-12.5780443898087,14.3402859058353,0.));
#14662=CARTESIAN_POINT('Ctrl Pts',(-12.5780443898087,14.3402859058353,21.));
#14663=CARTESIAN_POINT('Ctrl Pts',(-12.5534605602317,14.2997103098726,0.));
#14664=CARTESIAN_POINT('Ctrl Pts',(-12.5534605602317,14.2997103098726,21.));
#14665=CARTESIAN_POINT('Ctrl Pts',(-12.5285125321527,14.2594378207584,0.));
#14666=CARTESIAN_POINT('Ctrl Pts',(-12.5285125321527,14.2594378207584,21.));
#14667=CARTESIAN_POINT('Ctrl Pts',(-12.502885965175,14.2197144660135,0.));
#14668=CARTESIAN_POINT('Ctrl Pts',(-12.502885965175,14.2197144660135,21.));
#14669=CARTESIAN_POINT('Ctrl Pts',(-12.4761570639125,14.1808688343892,0.));
#14670=CARTESIAN_POINT('Ctrl Pts',(-12.4761570639125,14.1808688343892,21.));
#14671=CARTESIAN_POINT('Ctrl Pts',(-12.4535485619996,14.1507598477672,0.));
#14672=CARTESIAN_POINT('Ctrl Pts',(-12.4535485619996,14.1507598477672,21.));
#14673=CARTESIAN_POINT('Ctrl Pts',(-12.4357509724316,14.1288394445866,0.));
#14674=CARTESIAN_POINT('Ctrl Pts',(-12.4357509724316,14.1288394445866,21.));
#14675=CARTESIAN_POINT('Ctrl Pts',(-12.4234926340671,14.1145347042316,0.));
#14676=CARTESIAN_POINT('Ctrl Pts',(-12.4234926340671,14.1145347042316,21.));
#14677=CARTESIAN_POINT('Ctrl Pts',(-12.4172651441477,14.1074595503134,0.));
#14678=CARTESIAN_POINT('Ctrl Pts',(-12.4172651441477,14.1074595503134,21.));
#14679=CARTESIAN_POINT('',(-13.486901949342,17.3811241238545,0.));
#14680=CARTESIAN_POINT('Ctrl Pts',(-12.4172651441477,14.1074595503134,0.));
#14681=CARTESIAN_POINT('Ctrl Pts',(-12.4234926340671,14.1145347042316,0.));
#14682=CARTESIAN_POINT('Ctrl Pts',(-12.4357509724316,14.1288394445866,0.));
#14683=CARTESIAN_POINT('Ctrl Pts',(-12.4535485619996,14.1507598477672,0.));
#14684=CARTESIAN_POINT('Ctrl Pts',(-12.4761570639125,14.1808688343892,0.));
#14685=CARTESIAN_POINT('Ctrl Pts',(-12.502885965175,14.2197144660135,0.));
#14686=CARTESIAN_POINT('Ctrl Pts',(-12.5285125321527,14.2594378207584,0.));
#14687=CARTESIAN_POINT('Ctrl Pts',(-12.5534605602317,14.2997103098726,0.));
#14688=CARTESIAN_POINT('Ctrl Pts',(-12.5780443898087,14.3402859058353,0.));
#14689=CARTESIAN_POINT('Ctrl Pts',(-12.6023830189244,14.3810669346235,0.));
#14690=CARTESIAN_POINT('Ctrl Pts',(-12.626464614311,14.4220553460485,0.));
#14691=CARTESIAN_POINT('Ctrl Pts',(-12.6501984687124,14.463313553928,0.));
#14692=CARTESIAN_POINT('Ctrl Pts',(-12.6734695081852,14.5049233087958,0.));
#14693=CARTESIAN_POINT('Ctrl Pts',(-12.6961966430455,14.5469417071952,0.));
#14694=CARTESIAN_POINT('Ctrl Pts',(-12.7183743139638,14.5893698147583,0.));
#14695=CARTESIAN_POINT('Ctrl Pts',(-12.7400427996251,14.6321748083434,0.));
#14696=CARTESIAN_POINT('Ctrl Pts',(-12.7612687078867,14.6753044633399,0.));
#14697=CARTESIAN_POINT('Ctrl Pts',(-12.7821227233337,14.7187037124277,0.));
#14698=CARTESIAN_POINT('Ctrl Pts',(-12.8026557145457,14.7623324139791,0.));
#14699=CARTESIAN_POINT('Ctrl Pts',(-12.8228846016791,14.8061758577898,0.));
#14700=CARTESIAN_POINT('Ctrl Pts',(-12.8428057266944,14.8502347891476,0.));
#14701=CARTESIAN_POINT('Ctrl Pts',(-12.8624032236317,14.8945191569251,0.));
#14702=CARTESIAN_POINT('Ctrl Pts',(-12.8816587472147,14.9390408507356,0.));
#14703=CARTESIAN_POINT('Ctrl Pts',(-12.9005620742036,14.9838057866976,0.));
#14704=CARTESIAN_POINT('Ctrl Pts',(-12.9191164383568,15.0288099208306,0.));
#14705=CARTESIAN_POINT('Ctrl Pts',(-12.9373327960422,15.0740435169624,0.));
#14706=CARTESIAN_POINT('Ctrl Pts',(-12.9552263908864,15.1194937003528,0.));
#14707=CARTESIAN_POINT('Ctrl Pts',(-12.9728126886697,15.1651474813659,0.));
#14708=CARTESIAN_POINT('Ctrl Pts',(-12.9901029059182,15.2109950816083,0.));
#14709=CARTESIAN_POINT('Ctrl Pts',(-13.0071020851025,15.2570313635503,0.));
#14710=CARTESIAN_POINT('Ctrl Pts',(-13.0238115816728,15.3032539741328,0.));
#14711=CARTESIAN_POINT('Ctrl Pts',(-13.0402305665115,15.3496622219036,0.));
#14712=CARTESIAN_POINT('Ctrl Pts',(-13.0563577967298,15.3962557545684,0.));
#14713=CARTESIAN_POINT('Ctrl Pts',(-13.0721935806302,15.4430330918328,0.));
#14714=CARTESIAN_POINT('Ctrl Pts',(-13.087740560189,15.4899910401523,0.));
#14715=CARTESIAN_POINT('Ctrl Pts',(-13.1030026646917,15.5371254712111,0.));
#14716=CARTESIAN_POINT('Ctrl Pts',(-13.1179844917497,15.5844317820184,0.));
#14717=CARTESIAN_POINT('Ctrl Pts',(-13.1326905726717,15.6319054413079,0.));
#14718=CARTESIAN_POINT('Ctrl Pts',(-13.147124558532,15.6795425955901,0.));
#14719=CARTESIAN_POINT('Ctrl Pts',(-13.161288914421,15.7273402954914,0.));
#14720=CARTESIAN_POINT('Ctrl Pts',(-13.1751853728467,15.7752961549278,0.));
#14721=CARTESIAN_POINT('Ctrl Pts',(-13.1888152101588,15.8234081427091,0.));
#14722=CARTESIAN_POINT('Ctrl Pts',(-13.2021795724682,15.8716743375555,0.));
#14723=CARTESIAN_POINT('Ctrl Pts',(-13.2152798388134,15.9200926550954,0.));
#14724=CARTESIAN_POINT('Ctrl Pts',(-13.2281177675127,15.9686607385389,0.));
#14725=CARTESIAN_POINT('Ctrl Pts',(-13.240695304984,16.0173761036734,0.));
#14726=CARTESIAN_POINT('Ctrl Pts',(-13.2530144750236,16.0662362238032,0.));
#14727=CARTESIAN_POINT('Ctrl Pts',(-13.2650772466062,16.1152386305152,0.));
#14728=CARTESIAN_POINT('Ctrl Pts',(-13.2768853909882,16.1643810242643,0.));
#14729=CARTESIAN_POINT('Ctrl Pts',(-13.2884404210387,16.2136613184475,0.));
#14730=CARTESIAN_POINT('Ctrl Pts',(-13.2997436744733,16.2630775678735,0.));
#14731=CARTESIAN_POINT('Ctrl Pts',(-13.3107963665229,16.3126279218067,0.));
#14732=CARTESIAN_POINT('Ctrl Pts',(-13.3215996524974,16.3623105703343,0.));
#14733=CARTESIAN_POINT('Ctrl Pts',(-13.3321546976812,16.4121236828756,0.));
#14734=CARTESIAN_POINT('Ctrl Pts',(-13.3424627129921,16.4620653818862,0.));
#14735=CARTESIAN_POINT('Ctrl Pts',(-13.3525249163084,16.5121337902953,0.));
#14736=CARTESIAN_POINT('Ctrl Pts',(-13.3623425108873,16.5623270636327,0.));
#14737=CARTESIAN_POINT('Ctrl Pts',(-13.3719166600676,16.612643424234,0.));
#14738=CARTESIAN_POINT('Ctrl Pts',(-13.381248462113,16.6630812012276,0.));
#14739=CARTESIAN_POINT('Ctrl Pts',(-13.3903389370346,16.7136388432444,0.));
#14740=CARTESIAN_POINT('Ctrl Pts',(-13.3991890464165,16.7643148579873,0.));
#14741=CARTESIAN_POINT('Ctrl Pts',(-13.4077997088426,16.8151077630226,0.));
#14742=CARTESIAN_POINT('Ctrl Pts',(-13.4161718177499,16.8660160353187,0.));
#14743=CARTESIAN_POINT('Ctrl Pts',(-13.4243062623592,16.9170380509036,0.));
#14744=CARTESIAN_POINT('Ctrl Pts',(-13.432203941793,16.9681720567298,0.));
#14745=CARTESIAN_POINT('Ctrl Pts',(-13.4398657451291,17.0194162803447,0.));
#14746=CARTESIAN_POINT('Ctrl Pts',(-13.4472925380889,17.0707690194412,0.));
#14747=CARTESIAN_POINT('Ctrl Pts',(-13.4544851484583,17.1222287365697,0.));
#14748=CARTESIAN_POINT('Ctrl Pts',(-13.4614443545811,17.173794155624,0.));
#14749=CARTESIAN_POINT('Ctrl Pts',(-13.4695161752401,17.235798381426,0.));
#14750=CARTESIAN_POINT('Ctrl Pts',(-13.4759526005425,17.287598725272,0.));
#14751=CARTESIAN_POINT('Ctrl Pts',(-13.4809165957478,17.3291218739796,0.));
#14752=CARTESIAN_POINT('Ctrl Pts',(-13.4845355519784,17.360310805254,0.));
#14753=CARTESIAN_POINT('Ctrl Pts',(-13.4869019493419,17.3811241238545,0.));
#14754=CARTESIAN_POINT('',(-13.486901949342,17.3811241238545,13.));
#14755=CARTESIAN_POINT('Ctrl Pts',(-13.4869019493419,17.3811241238545,13.));
#14756=CARTESIAN_POINT('Ctrl Pts',(-13.475253226354,17.2786694026925,13.));
#14757=CARTESIAN_POINT('Ctrl Pts',(-13.4622625504827,17.1768129075703,13.));
#14758=CARTESIAN_POINT('Ctrl Pts',(-13.4479123002588,17.0755735571127,13.));
#14759=CARTESIAN_POINT('Ctrl Pts',(-13.4241333152838,16.9078155768783,13.));
#14760=CARTESIAN_POINT('Ctrl Pts',(-13.3966181281356,16.7417653304334,13.));
#14761=CARTESIAN_POINT('Ctrl Pts',(-13.365224404591,16.57767452627,13.));
#14762=CARTESIAN_POINT('Ctrl Pts',(-13.341093348038,16.4515447134285,13.));
#14763=CARTESIAN_POINT('Ctrl Pts',(-13.3146689195875,16.3265706105421,13.));
#14764=CARTESIAN_POINT('Ctrl Pts',(-13.2858665160047,16.2028831155019,13.));
#14765=CARTESIAN_POINT('Ctrl Pts',(-13.2548614253288,16.06973651931,13.));
#14766=CARTESIAN_POINT('Ctrl Pts',(-13.221105276728,15.9380763844413,13.));
#14767=CARTESIAN_POINT('Ctrl Pts',(-13.1844379732027,15.8081115249869,13.));
#14768=CARTESIAN_POINT('Ctrl Pts',(-13.1641379552808,15.7361594390004,13.));
#14769=CARTESIAN_POINT('Ctrl Pts',(-13.1429498666824,15.6647240119351,13.));
#14770=CARTESIAN_POINT('Ctrl Pts',(-13.1208442193483,15.5938437094451,13.));
#14771=CARTESIAN_POINT('Ctrl Pts',(-13.0995423541465,15.5255406814322,13.));
#14772=CARTESIAN_POINT('Ctrl Pts',(-13.0773830005559,15.4577571787665,13.));
#14773=CARTESIAN_POINT('Ctrl Pts',(-13.0543129132427,15.3905488552889,13.));
#14774=CARTESIAN_POINT('Ctrl Pts',(-13.0343732800281,15.33246024466,13.));
#14775=CARTESIAN_POINT('Ctrl Pts',(-13.0137559287927,15.2747993584962,13.));
#14776=CARTESIAN_POINT('Ctrl Pts',(-12.9924643459712,15.2175748374047,13.));
#14777=CARTESIAN_POINT('Ctrl Pts',(-12.9771843404906,15.1765073882052,13.));
#14778=CARTESIAN_POINT('Ctrl Pts',(-12.9615593601525,15.1356630008116,13.));
#14779=CARTESIAN_POINT('Ctrl Pts',(-12.9455599556256,15.0950681407047,13.));
#14780=CARTESIAN_POINT('Ctrl Pts',(-12.9298210808671,15.0551343157937,13.));
#14781=CARTESIAN_POINT('Ctrl Pts',(-12.9137147531571,15.0154457689919,13.));
#14782=CARTESIAN_POINT('Ctrl Pts',(-12.8972012565818,14.9760367892541,13.));
#14783=CARTESIAN_POINT('Ctrl Pts',(-12.8828830850643,14.9418668889764,13.));
#14784=CARTESIAN_POINT('Ctrl Pts',(-12.8682568220943,14.9079086467,13.));
#14785=CARTESIAN_POINT('Ctrl Pts',(-12.853336407922,14.8741550424141,13.));
#14786=CARTESIAN_POINT('Ctrl Pts',(-12.8398219364233,14.8435820222663,13.));
#14787=CARTESIAN_POINT('Ctrl Pts',(-12.8260705988221,14.8131735649528,13.));
#14788=CARTESIAN_POINT('Ctrl Pts',(-12.8121025758909,14.782917409017,13.));
#14789=CARTESIAN_POINT('Ctrl Pts',(-12.8003366510026,14.7574312210357,13.));
#14790=CARTESIAN_POINT('Ctrl Pts',(-12.7884183713523,14.7320520621591,13.));
#14791=CARTESIAN_POINT('Ctrl Pts',(-12.7763327021684,14.7067929859341,13.));
#14792=CARTESIAN_POINT('Ctrl Pts',(-12.7588434232842,14.6702403530813,13.));
#14793=CARTESIAN_POINT('Ctrl Pts',(-12.7410029355977,14.6339396294117,13.));
#14794=CARTESIAN_POINT('Ctrl Pts',(-12.7226389620173,14.5980256539368,13.));
#14795=CARTESIAN_POINT('Ctrl Pts',(-12.7115427372118,14.5763250375761,13.));
#14796=CARTESIAN_POINT('Ctrl Pts',(-12.7002526009286,14.5547677199977,13.));
#14797=CARTESIAN_POINT('Ctrl Pts',(-12.6887481998661,14.533370542697,13.));
#14798=CARTESIAN_POINT('Ctrl Pts',(-12.6781379056319,14.513636325704,13.));
#14799=CARTESIAN_POINT('Ctrl Pts',(-12.6673442954742,14.494039116296,13.));
#14800=CARTESIAN_POINT('Ctrl Pts',(-12.656388173598,14.4745649059699,13.));
#14801=CARTESIAN_POINT('Ctrl Pts',(-12.6413169181342,14.4477761569858,13.));
#14802=CARTESIAN_POINT('Ctrl Pts',(-12.6259439377184,14.4212156950323,13.));
#14803=CARTESIAN_POINT('Ctrl Pts',(-12.610392584142,14.3947967980035,13.));
#14804=CARTESIAN_POINT('Ctrl Pts',(-12.6005265277046,14.3780361779186,13.));
#14805=CARTESIAN_POINT('Ctrl Pts',(-12.5905900370373,14.3613315561545,13.));
#14806=CARTESIAN_POINT('Ctrl Pts',(-12.5805908896179,14.3446791500623,13.));
#14807=CARTESIAN_POINT('Ctrl Pts',(-12.5716171202366,14.3297343907096,13.));
#14808=CARTESIAN_POINT('Ctrl Pts',(-12.5625934694128,14.3148312513707,13.));
#14809=CARTESIAN_POINT('Ctrl Pts',(-12.5534931963782,14.2999916563209,13.));
#14810=CARTESIAN_POINT('Ctrl Pts',(-12.543926997017,14.2843922864836,13.));
#14811=CARTESIAN_POINT('Ctrl Pts',(-12.5342762592095,14.2688630442666,13.));
#14812=CARTESIAN_POINT('Ctrl Pts',(-12.5244602884878,14.2534670740361,13.));
#14813=CARTESIAN_POINT('Ctrl Pts',(-12.5081559827352,14.2278944013872,13.));
#14814=CARTESIAN_POINT('Ctrl Pts',(-12.4913891918921,14.2026946288704,13.));
#14815=CARTESIAN_POINT('Ctrl Pts',(-12.4736648236058,14.1782508275765,13.));
#14816=CARTESIAN_POINT('Ctrl Pts',(-12.4638909761696,14.1647716456531,13.));
#14817=CARTESIAN_POINT('Ctrl Pts',(-12.4538248359232,14.1515231428601,13.));
#14818=CARTESIAN_POINT('Ctrl Pts',(-12.443405435509,14.1385523184119,13.));
#14819=CARTESIAN_POINT('Ctrl Pts',(-12.4349297906026,14.1280012216313,13.));
#14820=CARTESIAN_POINT('Ctrl Pts',(-12.4262204477521,14.1176338183099,13.));
#14821=CARTESIAN_POINT('Ctrl Pts',(-12.4172651441477,14.1074595503134,13.));
#14822=CARTESIAN_POINT('',(-13.486901949342,17.3811241238545,0.));
#14823=CARTESIAN_POINT('Origin',(-3.33073116609659E-12,4.58435815896522E-12,
0.));
#14824=CARTESIAN_POINT('',(-12.3627494547115,18.1978687191668,0.));
#14825=CARTESIAN_POINT('Origin',(-3.33073116609659E-12,4.58435815896522E-12,
0.));
#14826=CARTESIAN_POINT('',(-12.3627494547115,18.1978687191668,13.));
#14827=CARTESIAN_POINT('Origin',(-3.33073116609659E-12,4.58435815896522E-12,
13.));
#14828=CARTESIAN_POINT('',(-12.3627494547115,18.1978687191668,0.));
#14829=CARTESIAN_POINT('Ctrl Pts',(-9.57984538049455,16.1689656784104,0.));
#14830=CARTESIAN_POINT('Ctrl Pts',(-9.57984538049455,16.1689656784104,21.));
#14831=CARTESIAN_POINT('Ctrl Pts',(-9.58464985151482,16.1770747160769,0.));
#14832=CARTESIAN_POINT('Ctrl Pts',(-9.58464985151482,16.1770747160769,21.));
#14833=CARTESIAN_POINT('Ctrl Pts',(-9.59446643316596,16.1931534965272,0.));
#14834=CARTESIAN_POINT('Ctrl Pts',(-9.59446643316596,16.1931534965272,21.));
#14835=CARTESIAN_POINT('Ctrl Pts',(-9.60981421781524,16.2168537871666,0.));
#14836=CARTESIAN_POINT('Ctrl Pts',(-9.60981421781524,16.2168537871666,21.));
#14837=CARTESIAN_POINT('Ctrl Pts',(-9.63146315443273,16.2476599387841,0.));
#14838=CARTESIAN_POINT('Ctrl Pts',(-9.63146315443273,16.2476599387841,21.));
#14839=CARTESIAN_POINT('Ctrl Pts',(-9.66014786078746,16.2850845948324,0.));
#14840=CARTESIAN_POINT('Ctrl Pts',(-9.66014786078746,16.2850845948324,21.));
#14841=CARTESIAN_POINT('Ctrl Pts',(-9.69000797146315,16.3217321000366,0.));
#14842=CARTESIAN_POINT('Ctrl Pts',(-9.69000797146315,16.3217321000366,21.));
#14843=CARTESIAN_POINT('Ctrl Pts',(-9.72060002001012,16.3579039682519,0.));
#14844=CARTESIAN_POINT('Ctrl Pts',(-9.72060002001012,16.3579039682519,21.));
#14845=CARTESIAN_POINT('Ctrl Pts',(-9.75159288382684,16.3938231282759,0.));
#14846=CARTESIAN_POINT('Ctrl Pts',(-9.75159288382684,16.3938231282759,21.));
#14847=CARTESIAN_POINT('Ctrl Pts',(-9.78285689698057,16.4295725710378,0.));
#14848=CARTESIAN_POINT('Ctrl Pts',(-9.78285689698057,16.4295725710378,21.));
#14849=CARTESIAN_POINT('Ctrl Pts',(-9.81439757053278,16.4651416449558,0.));
#14850=CARTESIAN_POINT('Ctrl Pts',(-9.81439757053278,16.4651416449558,21.));
#14851=CARTESIAN_POINT('Ctrl Pts',(-9.84630229363521,16.5004633692332,0.));
#14852=CARTESIAN_POINT('Ctrl Pts',(-9.84630229363521,16.5004633692332,21.));
#14853=CARTESIAN_POINT('Ctrl Pts',(-9.8786843754698,16.5354535643506,0.));
#14854=CARTESIAN_POINT('Ctrl Pts',(-9.8786843754698,16.5354535643506,21.));
#14855=CARTESIAN_POINT('Ctrl Pts',(-9.91162317616648,16.5700527532381,0.));
#14856=CARTESIAN_POINT('Ctrl Pts',(-9.91162317616648,16.5700527532381,21.));
#14857=CARTESIAN_POINT('Ctrl Pts',(-9.9451214271291,16.6042559779574,0.));
#14858=CARTESIAN_POINT('Ctrl Pts',(-9.9451214271291,16.6042559779574,21.));
#14859=CARTESIAN_POINT('Ctrl Pts',(-9.97913546489641,16.6380914029057,0.));
#14860=CARTESIAN_POINT('Ctrl Pts',(-9.97913546489641,16.6380914029057,21.));
#14861=CARTESIAN_POINT('Ctrl Pts',(-10.0135950379525,16.6716062376277,0.));
#14862=CARTESIAN_POINT('Ctrl Pts',(-10.0135950379525,16.6716062376277,21.));
#14863=CARTESIAN_POINT('Ctrl Pts',(-10.0484259314257,16.7048506904207,0.));
#14864=CARTESIAN_POINT('Ctrl Pts',(-10.0484259314257,16.7048506904207,21.));
#14865=CARTESIAN_POINT('Ctrl Pts',(-10.0835742491038,16.7378607357337,0.));
#14866=CARTESIAN_POINT('Ctrl Pts',(-10.0835742491038,16.7378607357337,21.));
#14867=CARTESIAN_POINT('Ctrl Pts',(-10.1190207721353,16.7706479198888,0.));
#14868=CARTESIAN_POINT('Ctrl Pts',(-10.1190207721353,16.7706479198888,21.));
#14869=CARTESIAN_POINT('Ctrl Pts',(-10.1547673397274,16.8032089941901,0.));
#14870=CARTESIAN_POINT('Ctrl Pts',(-10.1547673397274,16.8032089941901,21.));
#14871=CARTESIAN_POINT('Ctrl Pts',(-10.1908283166713,16.8355319435838,0.));
#14872=CARTESIAN_POINT('Ctrl Pts',(-10.1908283166713,16.8355319435838,21.));
#14873=CARTESIAN_POINT('Ctrl Pts',(-10.2272206796636,16.8676029947679,0.));
#14874=CARTESIAN_POINT('Ctrl Pts',(-10.2272206796636,16.8676029947679,21.));
#14875=CARTESIAN_POINT('Ctrl Pts',(-10.2639532144219,16.8994142530447,0.));
#14876=CARTESIAN_POINT('Ctrl Pts',(-10.2639532144219,16.8994142530447,21.));
#14877=CARTESIAN_POINT('Ctrl Pts',(-10.3010210756062,16.9309675442426,0.));
#14878=CARTESIAN_POINT('Ctrl Pts',(-10.3010210756062,16.9309675442426,21.));
#14879=CARTESIAN_POINT('Ctrl Pts',(-10.3384116178624,16.9622702798438,0.));
#14880=CARTESIAN_POINT('Ctrl Pts',(-10.3384116178624,16.9622702798438,21.));
#14881=CARTESIAN_POINT('Ctrl Pts',(-10.3761078860454,16.9933329788855,0.));
#14882=CARTESIAN_POINT('Ctrl Pts',(-10.3761078860454,16.9933329788855,21.));
#14883=CARTESIAN_POINT('Ctrl Pts',(-10.4140927470882,17.0241663361802,0.));
#14884=CARTESIAN_POINT('Ctrl Pts',(-10.4140927470882,17.0241663361802,21.));
#14885=CARTESIAN_POINT('Ctrl Pts',(-10.452353435089,17.0547779975888,0.));
#14886=CARTESIAN_POINT('Ctrl Pts',(-10.452353435089,17.0547779975888,21.));
#14887=CARTESIAN_POINT('Ctrl Pts',(-10.4908835057575,17.0851711712016,0.));
#14888=CARTESIAN_POINT('Ctrl Pts',(-10.4908835057575,17.0851711712016,21.));
#14889=CARTESIAN_POINT('Ctrl Pts',(-10.5296803023445,17.1153464189932,0.));
#14890=CARTESIAN_POINT('Ctrl Pts',(-10.5296803023445,17.1153464189932,21.));
#14891=CARTESIAN_POINT('Ctrl Pts',(-10.5687434234512,17.1453027387554,0.));
#14892=CARTESIAN_POINT('Ctrl Pts',(-10.5687434234512,17.1453027387554,21.));
#14893=CARTESIAN_POINT('Ctrl Pts',(-10.6080729180997,17.1750388395657,0.));
#14894=CARTESIAN_POINT('Ctrl Pts',(-10.6080729180997,17.1750388395657,21.));
#14895=CARTESIAN_POINT('Ctrl Pts',(-10.6476672831754,17.2045545572011,0.));
#14896=CARTESIAN_POINT('Ctrl Pts',(-10.6476672831754,17.2045545572011,21.));
#14897=CARTESIAN_POINT('Ctrl Pts',(-10.6875226650217,17.2338514174709,0.));
#14898=CARTESIAN_POINT('Ctrl Pts',(-10.6875226650217,17.2338514174709,21.));
#14899=CARTESIAN_POINT('Ctrl Pts',(-10.7276339231608,17.2629318816279,0.));
#14900=CARTESIAN_POINT('Ctrl Pts',(-10.7276339231608,17.2629318816279,21.));
#14901=CARTESIAN_POINT('Ctrl Pts',(-10.7679952591482,17.2917988998581,0.));
#14902=CARTESIAN_POINT('Ctrl Pts',(-10.7679952591482,17.2917988998581,21.));
#14903=CARTESIAN_POINT('Ctrl Pts',(-10.8086009632423,17.3204553814537,0.));
#14904=CARTESIAN_POINT('Ctrl Pts',(-10.8086009632423,17.3204553814537,21.));
#14905=CARTESIAN_POINT('Ctrl Pts',(-10.8494462423128,17.3489036079991,0.));
#14906=CARTESIAN_POINT('Ctrl Pts',(-10.8494462423128,17.3489036079991,21.));
#14907=CARTESIAN_POINT('Ctrl Pts',(-10.8905275295837,17.377145012528,0.));
#14908=CARTESIAN_POINT('Ctrl Pts',(-10.8905275295837,17.377145012528,21.));
#14909=CARTESIAN_POINT('Ctrl Pts',(-10.9318420203801,17.405180505413,0.));
#14910=CARTESIAN_POINT('Ctrl Pts',(-10.9318420203801,17.405180505413,21.));
#14911=CARTESIAN_POINT('Ctrl Pts',(-10.9733873885115,17.4330106728622,0.));
#14912=CARTESIAN_POINT('Ctrl Pts',(-10.9733873885115,17.4330106728622,21.));
#14913=CARTESIAN_POINT('Ctrl Pts',(-11.0151614525642,17.460636011184,0.));
#14914=CARTESIAN_POINT('Ctrl Pts',(-11.0151614525642,17.460636011184,21.));
#14915=CARTESIAN_POINT('Ctrl Pts',(-11.0571618040371,17.4880571878157,0.));
#14916=CARTESIAN_POINT('Ctrl Pts',(-11.0571618040371,17.4880571878157,21.));
#14917=CARTESIAN_POINT('Ctrl Pts',(-11.0993856581394,17.5152751467292,0.));
#14918=CARTESIAN_POINT('Ctrl Pts',(-11.0993856581394,17.5152751467292,21.));
#14919=CARTESIAN_POINT('Ctrl Pts',(-11.1418300507683,17.5422909714139,0.));
#14920=CARTESIAN_POINT('Ctrl Pts',(-11.1418300507683,17.5422909714139,21.));
#14921=CARTESIAN_POINT('Ctrl Pts',(-11.1844919535058,17.5691058058227,0.));
#14922=CARTESIAN_POINT('Ctrl Pts',(-11.1844919535058,17.5691058058227,21.));
#14923=CARTESIAN_POINT('Ctrl Pts',(-11.2273684103051,17.5957207597803,0.));
#14924=CARTESIAN_POINT('Ctrl Pts',(-11.2273684103051,17.5957207597803,21.));
#14925=CARTESIAN_POINT('Ctrl Pts',(-11.2704566868205,17.6221368072528,0.));
#14926=CARTESIAN_POINT('Ctrl Pts',(-11.2704566868205,17.6221368072528,21.));
#14927=CARTESIAN_POINT('Ctrl Pts',(-11.3137543310722,17.6483547422688,0.));
#14928=CARTESIAN_POINT('Ctrl Pts',(-11.3137543310722,17.6483547422688,21.));
#14929=CARTESIAN_POINT('Ctrl Pts',(-11.3572590796967,17.674375235974,0.));
#14930=CARTESIAN_POINT('Ctrl Pts',(-11.3572590796967,17.674375235974,21.));
#14931=CARTESIAN_POINT('Ctrl Pts',(-11.4009687970126,17.700198872213,0.));
#14932=CARTESIAN_POINT('Ctrl Pts',(-11.4009687970126,17.700198872213,21.));
#14933=CARTESIAN_POINT('Ctrl Pts',(-11.4448814046804,17.725826190457,0.));
#14934=CARTESIAN_POINT('Ctrl Pts',(-11.4448814046804,17.725826190457,21.));
#14935=CARTESIAN_POINT('Ctrl Pts',(-11.4889948016216,17.7512577332768,0.));
#14936=CARTESIAN_POINT('Ctrl Pts',(-11.4889948016216,17.7512577332768,21.));
#14937=CARTESIAN_POINT('Ctrl Pts',(-11.5333068279911,17.7764940721306,0.));
#14938=CARTESIAN_POINT('Ctrl Pts',(-11.5333068279911,17.7764940721306,21.));
#14939=CARTESIAN_POINT('Ctrl Pts',(-11.5778153222435,17.8015357852426,0.));
#14940=CARTESIAN_POINT('Ctrl Pts',(-11.5778153222435,17.8015357852426,21.));
#14941=CARTESIAN_POINT('Ctrl Pts',(-11.6225181583564,17.8263834470057,0.));
#14942=CARTESIAN_POINT('Ctrl Pts',(-11.6225181583564,17.8263834470057,21.));
#14943=CARTESIAN_POINT('Ctrl Pts',(-11.6674132861792,17.8510376144926,0.));
#14944=CARTESIAN_POINT('Ctrl Pts',(-11.6674132861792,17.8510376144926,21.));
#14945=CARTESIAN_POINT('Ctrl Pts',(-11.7124987772363,17.8754988158862,0.));
#14946=CARTESIAN_POINT('Ctrl Pts',(-11.7124987772363,17.8754988158862,21.));
#14947=CARTESIAN_POINT('Ctrl Pts',(-11.7577728408871,17.8997675418752,0.));
#14948=CARTESIAN_POINT('Ctrl Pts',(-11.7577728408871,17.8997675418752,21.));
#14949=CARTESIAN_POINT('Ctrl Pts',(-11.8032337607271,17.9238442458356,0.));
#14950=CARTESIAN_POINT('Ctrl Pts',(-11.8032337607271,17.9238442458356,21.));
#14951=CARTESIAN_POINT('Ctrl Pts',(-11.8488798430201,17.9477293432951,0.));
#14952=CARTESIAN_POINT('Ctrl Pts',(-11.8488798430201,17.9477293432951,21.));
#14953=CARTESIAN_POINT('Ctrl Pts',(-11.8947093631895,17.9714232133203,0.));
#14954=CARTESIAN_POINT('Ctrl Pts',(-11.8947093631895,17.9714232133203,21.));
#14955=CARTESIAN_POINT('Ctrl Pts',(-11.9407205019619,17.9949261997754,0.));
#14956=CARTESIAN_POINT('Ctrl Pts',(-11.9407205019619,17.9949261997754,21.));
#14957=CARTESIAN_POINT('Ctrl Pts',(-11.986911314246,18.0182386160553,0.));
#14958=CARTESIAN_POINT('Ctrl Pts',(-11.986911314246,18.0182386160553,21.));
#14959=CARTESIAN_POINT('Ctrl Pts',(-12.0332798395991,18.0413607600052,0.));
#14960=CARTESIAN_POINT('Ctrl Pts',(-12.0332798395991,18.0413607600052,21.));
#14961=CARTESIAN_POINT('Ctrl Pts',(-12.0798241915081,18.0642929289333,0.));
#14962=CARTESIAN_POINT('Ctrl Pts',(-12.0798241915081,18.0642929289333,21.));
#14963=CARTESIAN_POINT('Ctrl Pts',(-12.1265426519718,18.0870354350128,0.));
#14964=CARTESIAN_POINT('Ctrl Pts',(-12.1265426519718,18.0870354350128,21.));
#14965=CARTESIAN_POINT('Ctrl Pts',(-12.1734337668195,18.109588624154,0.));
#14966=CARTESIAN_POINT('Ctrl Pts',(-12.1734337668195,18.109588624154,21.));
#14967=CARTESIAN_POINT('Ctrl Pts',(-12.2204964278426,18.1319528884305,0.));
#14968=CARTESIAN_POINT('Ctrl Pts',(-12.2204964278426,18.1319528884305,21.));
#14969=CARTESIAN_POINT('Ctrl Pts',(-12.2677298318549,18.1541286139166,0.));
#14970=CARTESIAN_POINT('Ctrl Pts',(-12.2677298318549,18.1541286139166,21.));
#14971=CARTESIAN_POINT('Ctrl Pts',(-12.3056527265146,18.1717186310224,0.));
#14972=CARTESIAN_POINT('Ctrl Pts',(-12.3056527265146,18.1717186310224,21.));
#14973=CARTESIAN_POINT('Ctrl Pts',(-12.3341713636489,18.1848265584754,0.));
#14974=CARTESIAN_POINT('Ctrl Pts',(-12.3341713636489,18.1848265584754,21.));
#14975=CARTESIAN_POINT('Ctrl Pts',(-12.3532177620787,18.1935275957711,0.));
#14976=CARTESIAN_POINT('Ctrl Pts',(-12.3532177620787,18.1935275957711,21.));
#14977=CARTESIAN_POINT('Ctrl Pts',(-12.3627494547115,18.1978687191668,0.));
#14978=CARTESIAN_POINT('Ctrl Pts',(-12.3627494547115,18.1978687191668,21.));
#14979=CARTESIAN_POINT('Ctrl Pts',(-9.57984538049455,16.1689656784104,0.));
#14980=CARTESIAN_POINT('Ctrl Pts',(-9.58464985151482,16.1770747160769,0.));
#14981=CARTESIAN_POINT('Ctrl Pts',(-9.59446643316596,16.1931534965272,0.));
#14982=CARTESIAN_POINT('Ctrl Pts',(-9.60981421781524,16.2168537871666,0.));
#14983=CARTESIAN_POINT('Ctrl Pts',(-9.63146315443273,16.2476599387841,0.));
#14984=CARTESIAN_POINT('Ctrl Pts',(-9.66014786078746,16.2850845948324,0.));
#14985=CARTESIAN_POINT('Ctrl Pts',(-9.69000797146315,16.3217321000366,0.));
#14986=CARTESIAN_POINT('Ctrl Pts',(-9.72060002001012,16.3579039682519,0.));
#14987=CARTESIAN_POINT('Ctrl Pts',(-9.75159288382684,16.3938231282759,0.));
#14988=CARTESIAN_POINT('Ctrl Pts',(-9.78285689698057,16.4295725710378,0.));
#14989=CARTESIAN_POINT('Ctrl Pts',(-9.81439757053278,16.4651416449558,0.));
#14990=CARTESIAN_POINT('Ctrl Pts',(-9.84630229363521,16.5004633692332,0.));
#14991=CARTESIAN_POINT('Ctrl Pts',(-9.8786843754698,16.5354535643506,0.));
#14992=CARTESIAN_POINT('Ctrl Pts',(-9.91162317616648,16.5700527532381,0.));
#14993=CARTESIAN_POINT('Ctrl Pts',(-9.9451214271291,16.6042559779574,0.));
#14994=CARTESIAN_POINT('Ctrl Pts',(-9.97913546489641,16.6380914029057,0.));
#14995=CARTESIAN_POINT('Ctrl Pts',(-10.0135950379525,16.6716062376277,0.));
#14996=CARTESIAN_POINT('Ctrl Pts',(-10.0484259314257,16.7048506904207,0.));
#14997=CARTESIAN_POINT('Ctrl Pts',(-10.0835742491038,16.7378607357337,0.));
#14998=CARTESIAN_POINT('Ctrl Pts',(-10.1190207721353,16.7706479198888,0.));
#14999=CARTESIAN_POINT('Ctrl Pts',(-10.1547673397274,16.8032089941901,0.));
#15000=CARTESIAN_POINT('Ctrl Pts',(-10.1908283166713,16.8355319435838,0.));
#15001=CARTESIAN_POINT('Ctrl Pts',(-10.2272206796636,16.8676029947679,0.));
#15002=CARTESIAN_POINT('Ctrl Pts',(-10.2639532144219,16.8994142530447,0.));
#15003=CARTESIAN_POINT('Ctrl Pts',(-10.3010210756062,16.9309675442426,0.));
#15004=CARTESIAN_POINT('Ctrl Pts',(-10.3384116178624,16.9622702798438,0.));
#15005=CARTESIAN_POINT('Ctrl Pts',(-10.3761078860454,16.9933329788855,0.));
#15006=CARTESIAN_POINT('Ctrl Pts',(-10.4140927470882,17.0241663361802,0.));
#15007=CARTESIAN_POINT('Ctrl Pts',(-10.452353435089,17.0547779975888,0.));
#15008=CARTESIAN_POINT('Ctrl Pts',(-10.4908835057575,17.0851711712016,0.));
#15009=CARTESIAN_POINT('Ctrl Pts',(-10.5296803023445,17.1153464189932,0.));
#15010=CARTESIAN_POINT('Ctrl Pts',(-10.5687434234512,17.1453027387554,0.));
#15011=CARTESIAN_POINT('Ctrl Pts',(-10.6080729180997,17.1750388395657,0.));
#15012=CARTESIAN_POINT('Ctrl Pts',(-10.6476672831754,17.2045545572011,0.));
#15013=CARTESIAN_POINT('Ctrl Pts',(-10.6875226650217,17.2338514174709,0.));
#15014=CARTESIAN_POINT('Ctrl Pts',(-10.7276339231608,17.2629318816279,0.));
#15015=CARTESIAN_POINT('Ctrl Pts',(-10.7679952591482,17.2917988998581,0.));
#15016=CARTESIAN_POINT('Ctrl Pts',(-10.8086009632423,17.3204553814537,0.));
#15017=CARTESIAN_POINT('Ctrl Pts',(-10.8494462423128,17.3489036079991,0.));
#15018=CARTESIAN_POINT('Ctrl Pts',(-10.8905275295837,17.377145012528,0.));
#15019=CARTESIAN_POINT('Ctrl Pts',(-10.9318420203801,17.405180505413,0.));
#15020=CARTESIAN_POINT('Ctrl Pts',(-10.9733873885115,17.4330106728622,0.));
#15021=CARTESIAN_POINT('Ctrl Pts',(-11.0151614525642,17.460636011184,0.));
#15022=CARTESIAN_POINT('Ctrl Pts',(-11.0571618040371,17.4880571878157,0.));
#15023=CARTESIAN_POINT('Ctrl Pts',(-11.0993856581394,17.5152751467292,0.));
#15024=CARTESIAN_POINT('Ctrl Pts',(-11.1418300507683,17.5422909714139,0.));
#15025=CARTESIAN_POINT('Ctrl Pts',(-11.1844919535058,17.5691058058227,0.));
#15026=CARTESIAN_POINT('Ctrl Pts',(-11.2273684103051,17.5957207597803,0.));
#15027=CARTESIAN_POINT('Ctrl Pts',(-11.2704566868205,17.6221368072528,0.));
#15028=CARTESIAN_POINT('Ctrl Pts',(-11.3137543310722,17.6483547422688,0.));
#15029=CARTESIAN_POINT('Ctrl Pts',(-11.3572590796967,17.674375235974,0.));
#15030=CARTESIAN_POINT('Ctrl Pts',(-11.4009687970126,17.700198872213,0.));
#15031=CARTESIAN_POINT('Ctrl Pts',(-11.4448814046804,17.725826190457,0.));
#15032=CARTESIAN_POINT('Ctrl Pts',(-11.4889948016216,17.7512577332768,0.));
#15033=CARTESIAN_POINT('Ctrl Pts',(-11.5333068279911,17.7764940721306,0.));
#15034=CARTESIAN_POINT('Ctrl Pts',(-11.5778153222435,17.8015357852426,0.));
#15035=CARTESIAN_POINT('Ctrl Pts',(-11.6225181583564,17.8263834470057,0.));
#15036=CARTESIAN_POINT('Ctrl Pts',(-11.6674132861792,17.8510376144926,0.));
#15037=CARTESIAN_POINT('Ctrl Pts',(-11.7124987772363,17.8754988158862,0.));
#15038=CARTESIAN_POINT('Ctrl Pts',(-11.7577728408871,17.8997675418752,0.));
#15039=CARTESIAN_POINT('Ctrl Pts',(-11.8032337607271,17.9238442458356,0.));
#15040=CARTESIAN_POINT('Ctrl Pts',(-11.8488798430201,17.9477293432951,0.));
#15041=CARTESIAN_POINT('Ctrl Pts',(-11.8947093631895,17.9714232133203,0.));
#15042=CARTESIAN_POINT('Ctrl Pts',(-11.9407205019619,17.9949261997754,0.));
#15043=CARTESIAN_POINT('Ctrl Pts',(-11.986911314246,18.0182386160553,0.));
#15044=CARTESIAN_POINT('Ctrl Pts',(-12.0332798395991,18.0413607600052,0.));
#15045=CARTESIAN_POINT('Ctrl Pts',(-12.0798241915081,18.0642929289333,0.));
#15046=CARTESIAN_POINT('Ctrl Pts',(-12.1265426519718,18.0870354350128,0.));
#15047=CARTESIAN_POINT('Ctrl Pts',(-12.1734337668195,18.109588624154,0.));
#15048=CARTESIAN_POINT('Ctrl Pts',(-12.2299089600472,18.1364257412858,0.));
#15049=CARTESIAN_POINT('Ctrl Pts',(-12.2771850498068,18.1585543320743,0.));
#15050=CARTESIAN_POINT('Ctrl Pts',(-12.3151419520839,18.1761067306718,0.));
#15051=CARTESIAN_POINT('Ctrl Pts',(-12.3436860694314,18.1891864723772,0.));
#15052=CARTESIAN_POINT('Ctrl Pts',(-12.3627494547115,18.1978687191668,0.));
#15053=CARTESIAN_POINT('Ctrl Pts',(-9.57984538049455,16.1689656784104,13.));
#15054=CARTESIAN_POINT('Ctrl Pts',(-9.58794311444298,16.1826331205334,13.));
#15055=CARTESIAN_POINT('Ctrl Pts',(-9.59639855902712,16.1960605405031,13.));
#15056=CARTESIAN_POINT('Ctrl Pts',(-9.60518801711085,16.209264165571,13.));
#15057=CARTESIAN_POINT('Ctrl Pts',(-9.6154899193841,16.224739801703,13.));
#15058=CARTESIAN_POINT('Ctrl Pts',(-9.62624998107167,16.2399084848584,13.));
#15059=CARTESIAN_POINT('Ctrl Pts',(-9.63737105568732,16.254836637175,13.));
#15060=CARTESIAN_POINT('Ctrl Pts',(-9.65301893989002,16.2758412618972,13.));
#15061=CARTESIAN_POINT('Ctrl Pts',(-9.66937567449949,16.296373798599,13.));
#15062=CARTESIAN_POINT('Ctrl Pts',(-9.68610238201322,16.3166650331518,13.));
#15063=CARTESIAN_POINT('Ctrl Pts',(-9.69722828051063,16.3301619042985,13.));
#15064=CARTESIAN_POINT('Ctrl Pts',(-9.70851618070807,16.3435531467518,13.));
#15065=CARTESIAN_POINT('Ctrl Pts',(-9.7198910779208,16.3568892752788,13.));
#15066=CARTESIAN_POINT('Ctrl Pts',(-9.73186502184932,16.3709277366574,13.));
#15067=CARTESIAN_POINT('Ctrl Pts',(-9.74393463776872,16.3849056240572,13.));
#15068=CARTESIAN_POINT('Ctrl Pts',(-9.75606525513648,16.3988451548219,13.));
#15069=CARTESIAN_POINT('Ctrl Pts',(-9.76953696975778,16.414325766791,13.));
#15070=CARTESIAN_POINT('Ctrl Pts',(-9.78308498747417,16.4297583183324,13.));
#15071=CARTESIAN_POINT('Ctrl Pts',(-9.79671869019648,16.4451338763398,13.));
#15072=CARTESIAN_POINT('Ctrl Pts',(-9.8172721587789,16.4683132763075,13.));
#15073=CARTESIAN_POINT('Ctrl Pts',(-9.83802550134249,16.4913594464712,13.));
#15074=CARTESIAN_POINT('Ctrl Pts',(-9.85910360864921,16.5141788054336,13.));
#15075=CARTESIAN_POINT('Ctrl Pts',(-9.87441639279172,16.5307565708362,13.));
#15076=CARTESIAN_POINT('Ctrl Pts',(-9.88990330206224,16.5472127770975,13.));
#15077=CARTESIAN_POINT('Ctrl Pts',(-9.90558047214324,16.5635345032205,13.));
#15078=CARTESIAN_POINT('Ctrl Pts',(-9.92474447016175,16.5834864158081,13.));
#15079=CARTESIAN_POINT('Ctrl Pts',(-9.9441917311001,16.6032381063718,13.));
#15080=CARTESIAN_POINT('Ctrl Pts',(-9.96388214930656,16.6228156007807,13.));
#15081=CARTESIAN_POINT('Ctrl Pts',(-9.9851510689085,16.6439625439398,13.));
#15082=CARTESIAN_POINT('Ctrl Pts',(-10.006698815053,16.6649096998191,13.));
#15083=CARTESIAN_POINT('Ctrl Pts',(-10.0284493480904,16.6857083247995,13.));
#15084=CARTESIAN_POINT('Ctrl Pts',(-10.0485293380076,16.7049095176705,13.));
#15085=CARTESIAN_POINT('Ctrl Pts',(-10.0687801145851,16.7239855768682,13.));
#15086=CARTESIAN_POINT('Ctrl Pts',(-10.0891775910162,16.7429517500628,13.));
#15087=CARTESIAN_POINT('Ctrl Pts',(-10.1168886100216,16.7687182701337,13.));
#15088=CARTESIAN_POINT('Ctrl Pts',(-10.1448719871919,16.7942808297111,13.));
#15089=CARTESIAN_POINT('Ctrl Pts',(-10.1731502199822,16.8196194580034,13.));
#15090=CARTESIAN_POINT('Ctrl Pts',(-10.2004381038963,16.844070687064,13.));
#15091=CARTESIAN_POINT('Ctrl Pts',(-10.2280069309447,16.8683088890975,13.));
#15092=CARTESIAN_POINT('Ctrl Pts',(-10.2558682820918,16.8923226175541,13.));
#15093=CARTESIAN_POINT('Ctrl Pts',(-10.2937187080479,16.9249459403096,13.));
#15094=CARTESIAN_POINT('Ctrl Pts',(-10.3321063567812,16.9571568356211,13.));
#15095=CARTESIAN_POINT('Ctrl Pts',(-10.3709578724058,16.9889999235317,13.));
#15096=CARTESIAN_POINT('Ctrl Pts',(-10.4051075100498,17.0169893055707,13.));
#15097=CARTESIAN_POINT('Ctrl Pts',(-10.4396099589146,17.04469848632,13.));
#15098=CARTESIAN_POINT('Ctrl Pts',(-10.474436876203,17.0721430001642,13.));
#15099=CARTESIAN_POINT('Ctrl Pts',(-10.5257802081583,17.112602877017,13.));
#15100=CARTESIAN_POINT('Ctrl Pts',(-10.5778361036082,17.1524822680152,13.));
#15101=CARTESIAN_POINT('Ctrl Pts',(-10.6305946314222,17.1917748564523,13.));
#15102=CARTESIAN_POINT('Ctrl Pts',(-10.6971764080832,17.2413624862848,13.));
#15103=CARTESIAN_POINT('Ctrl Pts',(-10.7648729797973,17.2900185098528,13.));
#15104=CARTESIAN_POINT('Ctrl Pts',(-10.8335716334697,17.3377983051247,13.));
#15105=CARTESIAN_POINT('Ctrl Pts',(-10.9266292559136,17.4025197212104,13.));
#15106=CARTESIAN_POINT('Ctrl Pts',(-11.0215303643735,17.465629946501,13.));
#15107=CARTESIAN_POINT('Ctrl Pts',(-11.1181400554829,17.5271690583862,13.));
#15108=CARTESIAN_POINT('Ctrl Pts',(-11.2042701255893,17.5820327885162,13.));
#15109=CARTESIAN_POINT('Ctrl Pts',(-11.2917512652755,17.6356526662346,13.));
#15110=CARTESIAN_POINT('Ctrl Pts',(-11.3804891386083,17.6880597469658,13.));
#15111=CARTESIAN_POINT('Ctrl Pts',(-11.5062551071101,17.7623349917623,13.));
#15112=CARTESIAN_POINT('Ctrl Pts',(-11.6345494475067,17.8341701535583,13.));
#15113=CARTESIAN_POINT('Ctrl Pts',(-11.7651542350891,17.9036238122623,13.));
#15114=CARTESIAN_POINT('Ctrl Pts',(-11.8666049261148,17.9575737615728,13.));
#15115=CARTESIAN_POINT('Ctrl Pts',(-11.9694546915569,18.0100864746768,13.));
#15116=CARTESIAN_POINT('Ctrl Pts',(-12.0736101881878,18.0611784501095,13.));
#15117=CARTESIAN_POINT('Ctrl Pts',(-12.163712553743,18.1053768649439,13.));
#15118=CARTESIAN_POINT('Ctrl Pts',(-12.2547877895871,18.1485120955669,13.));
#15119=CARTESIAN_POINT('Ctrl Pts',(-12.346811245556,18.1905949538241,13.));
#15120=CARTESIAN_POINT('Ctrl Pts',(-12.3521208117116,18.1930230491134,13.));
#15121=CARTESIAN_POINT('Ctrl Pts',(-12.357433548157,18.1954476374973,13.));
#15122=CARTESIAN_POINT('Ctrl Pts',(-12.3627494547115,18.1978687191668,13.));
#15123=CARTESIAN_POINT('Ctrl Pts',(-7.45574324794401,20.698113262342,0.));
#15124=CARTESIAN_POINT('Ctrl Pts',(-7.45574324794401,20.698113262342,21.));
#15125=CARTESIAN_POINT('Ctrl Pts',(-7.45783379370107,20.6878503127065,0.));
#15126=CARTESIAN_POINT('Ctrl Pts',(-7.45783379370107,20.6878503127065,21.));
#15127=CARTESIAN_POINT('Ctrl Pts',(-7.46198969876653,20.6673271112931,0.));
#15128=CARTESIAN_POINT('Ctrl Pts',(-7.46198969876653,20.6673271112931,21.));
#15129=CARTESIAN_POINT('Ctrl Pts',(-7.46814799701905,20.6365504027501,0.));
#15130=CARTESIAN_POINT('Ctrl Pts',(-7.46814799701905,20.6365504027501,21.));
#15131=CARTESIAN_POINT('Ctrl Pts',(-7.47620789245427,20.5955309838521,0.));
#15132=CARTESIAN_POINT('Ctrl Pts',(-7.47620789245427,20.5955309838521,21.));
#15133=CARTESIAN_POINT('Ctrl Pts',(-7.48603045196744,20.5442837929044,0.));
#15134=CARTESIAN_POINT('Ctrl Pts',(-7.48603045196744,20.5442837929044,21.));
#15135=CARTESIAN_POINT('Ctrl Pts',(-7.49560012018405,20.4930639156161,0.));
#15136=CARTESIAN_POINT('Ctrl Pts',(-7.49560012018405,20.4930639156161,21.));
#15137=CARTESIAN_POINT('Ctrl Pts',(-7.50491611266253,20.4418717748497,0.));
#15138=CARTESIAN_POINT('Ctrl Pts',(-7.50491611266253,20.4418717748497,21.));
#15139=CARTESIAN_POINT('Ctrl Pts',(-7.51397746081993,20.3907080367098,0.));
#15140=CARTESIAN_POINT('Ctrl Pts',(-7.51397746081993,20.3907080367098,21.));
#15141=CARTESIAN_POINT('Ctrl Pts',(-7.52278303006887,20.3395736743243,0.));
#15142=CARTESIAN_POINT('Ctrl Pts',(-7.52278303006887,20.3395736743243,21.));
#15143=CARTESIAN_POINT('Ctrl Pts',(-7.53133155804007,20.2884698940944,0.));
#15144=CARTESIAN_POINT('Ctrl Pts',(-7.53133155804007,20.2884698940944,21.));
#15145=CARTESIAN_POINT('Ctrl Pts',(-7.53962169534166,20.2373980474879,0.));
#15146=CARTESIAN_POINT('Ctrl Pts',(-7.53962169534166,20.2373980474879,21.));
#15147=CARTESIAN_POINT('Ctrl Pts',(-7.54765204869254,20.1863595454674,0.));
#15148=CARTESIAN_POINT('Ctrl Pts',(-7.54765204869254,20.1863595454674,21.));
#15149=CARTESIAN_POINT('Ctrl Pts',(-7.55542122125494,20.1353557774357,0.));
#15150=CARTESIAN_POINT('Ctrl Pts',(-7.55542122125494,20.1353557774357,21.));
#15151=CARTESIAN_POINT('Ctrl Pts',(-7.5629278654946,20.0843880130978,0.));
#15152=CARTESIAN_POINT('Ctrl Pts',(-7.5629278654946,20.0843880130978,21.));
#15153=CARTESIAN_POINT('Ctrl Pts',(-7.57017066105973,20.0334574248556,0.));
#15154=CARTESIAN_POINT('Ctrl Pts',(-7.57017066105973,20.0334574248556,21.));
#15155=CARTESIAN_POINT('Ctrl Pts',(-7.57714827622806,19.9825651387294,0.));
#15156=CARTESIAN_POINT('Ctrl Pts',(-7.57714827622806,19.9825651387294,21.));
#15157=CARTESIAN_POINT('Ctrl Pts',(-7.58385933533351,19.931712276832,0.));
#15158=CARTESIAN_POINT('Ctrl Pts',(-7.58385933533351,19.931712276832,21.));
#15159=CARTESIAN_POINT('Ctrl Pts',(-7.59030238888852,19.8808999994024,0.));
#15160=CARTESIAN_POINT('Ctrl Pts',(-7.59030238888852,19.8808999994024,21.));
#15161=CARTESIAN_POINT('Ctrl Pts',(-7.59647587605448,19.830129556152,0.));
#15162=CARTESIAN_POINT('Ctrl Pts',(-7.59647587605448,19.830129556152,21.));
#15163=CARTESIAN_POINT('Ctrl Pts',(-7.60237814110186,19.7794022782484,0.));
#15164=CARTESIAN_POINT('Ctrl Pts',(-7.60237814110186,19.7794022782484,21.));
#15165=CARTESIAN_POINT('Ctrl Pts',(-7.60800746969261,19.7287195480601,0.));
#15166=CARTESIAN_POINT('Ctrl Pts',(-7.60800746969261,19.7287195480601,21.));
#15167=CARTESIAN_POINT('Ctrl Pts',(-7.61336212350879,19.6780827744426,0.));
#15168=CARTESIAN_POINT('Ctrl Pts',(-7.61336212350879,19.6780827744426,21.));
#15169=CARTESIAN_POINT('Ctrl Pts',(-7.6184403707059,19.6274933688524,0.));
#15170=CARTESIAN_POINT('Ctrl Pts',(-7.6184403707059,19.6274933688524,21.));
#15171=CARTESIAN_POINT('Ctrl Pts',(-7.62324053735219,19.5769527121826,0.));
#15172=CARTESIAN_POINT('Ctrl Pts',(-7.62324053735219,19.5769527121826,21.));
#15173=CARTESIAN_POINT('Ctrl Pts',(-7.62776096538882,19.5264621687521,0.));
#15174=CARTESIAN_POINT('Ctrl Pts',(-7.62776096538882,19.5264621687521,21.));
#15175=CARTESIAN_POINT('Ctrl Pts',(-7.63199992715365,19.4760231231881,0.));
#15176=CARTESIAN_POINT('Ctrl Pts',(-7.63199992715365,19.4760231231881,21.));
#15177=CARTESIAN_POINT('Ctrl Pts',(-7.63595554930654,19.4256370121006,0.));
#15178=CARTESIAN_POINT('Ctrl Pts',(-7.63595554930654,19.4256370121006,21.));
#15179=CARTESIAN_POINT('Ctrl Pts',(-7.6396257482276,19.3753053524647,0.));
#15180=CARTESIAN_POINT('Ctrl Pts',(-7.6396257482276,19.3753053524647,21.));
#15181=CARTESIAN_POINT('Ctrl Pts',(-7.64300812875338,19.3250297839295,0.));
#15182=CARTESIAN_POINT('Ctrl Pts',(-7.64300812875338,19.3250297839295,21.));
#15183=CARTESIAN_POINT('Ctrl Pts',(-7.64610005549613,19.2748120456486,0.));
#15184=CARTESIAN_POINT('Ctrl Pts',(-7.64610005549613,19.2748120456486,21.));
#15185=CARTESIAN_POINT('Ctrl Pts',(-7.64889882291923,19.224653915265,0.));
#15186=CARTESIAN_POINT('Ctrl Pts',(-7.64889882291923,19.224653915265,21.));
#15187=CARTESIAN_POINT('Ctrl Pts',(-7.65140181220525,19.1745571539291,0.));
#15188=CARTESIAN_POINT('Ctrl Pts',(-7.65140181220525,19.1745571539291,21.));
#15189=CARTESIAN_POINT('Ctrl Pts',(-7.65360662280609,19.1245234597312,0.));
#15190=CARTESIAN_POINT('Ctrl Pts',(-7.65360662280609,19.1245234597312,21.));
#15191=CARTESIAN_POINT('Ctrl Pts',(-7.65551129907201,19.0745543888799,0.));
#15192=CARTESIAN_POINT('Ctrl Pts',(-7.65551129907201,19.0745543888799,21.));
#15193=CARTESIAN_POINT('Ctrl Pts',(-7.65711415727855,19.0246514144531,0.));
#15194=CARTESIAN_POINT('Ctrl Pts',(-7.65711415727855,19.0246514144531,21.));
#15195=CARTESIAN_POINT('Ctrl Pts',(-7.65841335587266,18.974816073814,0.));
#15196=CARTESIAN_POINT('Ctrl Pts',(-7.65841335587266,18.974816073814,21.));
#15197=CARTESIAN_POINT('Ctrl Pts',(-7.65940650980098,18.9250501008887,0.));
#15198=CARTESIAN_POINT('Ctrl Pts',(-7.65940650980098,18.9250501008887,21.));
#15199=CARTESIAN_POINT('Ctrl Pts',(-7.66009036321663,18.8753555389435,0.));
#15200=CARTESIAN_POINT('Ctrl Pts',(-7.66009036321663,18.8753555389435,21.));
#15201=CARTESIAN_POINT('Ctrl Pts',(-7.66046025294774,18.8257349246207,0.));
#15202=CARTESIAN_POINT('Ctrl Pts',(-7.66046025294774,18.8257349246207,21.));
#15203=CARTESIAN_POINT('Ctrl Pts',(-7.6605104692254,18.7761911671591,0.));
#15204=CARTESIAN_POINT('Ctrl Pts',(-7.6605104692254,18.7761911671591,21.));
#15205=CARTESIAN_POINT('Ctrl Pts',(-7.66023521705904,18.7267272235231,0.));
#15206=CARTESIAN_POINT('Ctrl Pts',(-7.66023521705904,18.7267272235231,21.));
#15207=CARTESIAN_POINT('Ctrl Pts',(-7.65962948375621,18.6773458057584,0.));
#15208=CARTESIAN_POINT('Ctrl Pts',(-7.65962948375621,18.6773458057584,21.));
#15209=CARTESIAN_POINT('Ctrl Pts',(-7.65868976978872,18.6280491346907,0.));
#15210=CARTESIAN_POINT('Ctrl Pts',(-7.65868976978872,18.6280491346907,21.));
#15211=CARTESIAN_POINT('Ctrl Pts',(-7.65741532450727,18.5788385228928,0.));
#15212=CARTESIAN_POINT('Ctrl Pts',(-7.65741532450727,18.5788385228928,21.));
#15213=CARTESIAN_POINT('Ctrl Pts',(-7.65580722110436,18.5297146894905,0.));
#15214=CARTESIAN_POINT('Ctrl Pts',(-7.65580722110436,18.5297146894905,21.));
#15215=CARTESIAN_POINT('Ctrl Pts',(-7.65386603444742,18.4806785483052,0.));
#15216=CARTESIAN_POINT('Ctrl Pts',(-7.65386603444742,18.4806785483052,21.));
#15217=CARTESIAN_POINT('Ctrl Pts',(-7.65158974829126,18.4317319183719,0.));
#15218=CARTESIAN_POINT('Ctrl Pts',(-7.65158974829126,18.4317319183719,21.));
#15219=CARTESIAN_POINT('Ctrl Pts',(-7.6489719793775,18.3828781275628,0.));
#15220=CARTESIAN_POINT('Ctrl Pts',(-7.6489719793775,18.3828781275628,21.));
#15221=CARTESIAN_POINT('Ctrl Pts',(-7.64599903846601,18.3341230095852,0.));
#15222=CARTESIAN_POINT('Ctrl Pts',(-7.64599903846601,18.3341230095852,21.));
#15223=CARTESIAN_POINT('Ctrl Pts',(-7.6426522027076,18.2854741391282,0.));
#15224=CARTESIAN_POINT('Ctrl Pts',(-7.6426522027076,18.2854741391282,21.));
#15225=CARTESIAN_POINT('Ctrl Pts',(-7.63891299603826,18.2369390502576,0.));
#15226=CARTESIAN_POINT('Ctrl Pts',(-7.63891299603826,18.2369390502576,21.));
#15227=CARTESIAN_POINT('Ctrl Pts',(-7.63476798969016,18.1885236169197,0.));
#15228=CARTESIAN_POINT('Ctrl Pts',(-7.63476798969016,18.1885236169197,21.));
#15229=CARTESIAN_POINT('Ctrl Pts',(-7.63021285851761,18.1402306858819,0.));
#15230=CARTESIAN_POINT('Ctrl Pts',(-7.63021285851761,18.1402306858819,21.));
#15231=CARTESIAN_POINT('Ctrl Pts',(-7.62525915358073,18.0920577897363,0.));
#15232=CARTESIAN_POINT('Ctrl Pts',(-7.62525915358073,18.0920577897363,21.));
#15233=CARTESIAN_POINT('Ctrl Pts',(-7.61992799636654,18.0439992897906,0.));
#15234=CARTESIAN_POINT('Ctrl Pts',(-7.61992799636654,18.0439992897906,21.));
#15235=CARTESIAN_POINT('Ctrl Pts',(-7.61423755067037,17.9960506269561,0.));
#15236=CARTESIAN_POINT('Ctrl Pts',(-7.61423755067037,17.9960506269561,21.));
#15237=CARTESIAN_POINT('Ctrl Pts',(-7.60819152580111,17.9482122228183,0.));
#15238=CARTESIAN_POINT('Ctrl Pts',(-7.60819152580111,17.9482122228183,21.));
#15239=CARTESIAN_POINT('Ctrl Pts',(-7.60176928403058,17.900492838997,0.));
#15240=CARTESIAN_POINT('Ctrl Pts',(-7.60176928403058,17.900492838997,21.));
#15241=CARTESIAN_POINT('Ctrl Pts',(-7.59491004201955,17.8529149331931,0.));
#15242=CARTESIAN_POINT('Ctrl Pts',(-7.59491004201955,17.8529149331931,21.));
#15243=CARTESIAN_POINT('Ctrl Pts',(-7.58752955799499,17.8055090348024,0.));
#15244=CARTESIAN_POINT('Ctrl Pts',(-7.58752955799499,17.8055090348024,21.));
#15245=CARTESIAN_POINT('Ctrl Pts',(-7.57954834582803,17.7583042294209,0.));
#15246=CARTESIAN_POINT('Ctrl Pts',(-7.57954834582803,17.7583042294209,21.));
#15247=CARTESIAN_POINT('Ctrl Pts',(-7.57091795530423,17.7113192869136,0.));
#15248=CARTESIAN_POINT('Ctrl Pts',(-7.57091795530423,17.7113192869136,21.));
#15249=CARTESIAN_POINT('Ctrl Pts',(-7.56164400295862,17.6645549117314,0.));
#15250=CARTESIAN_POINT('Ctrl Pts',(-7.56164400295862,17.6645549117314,21.));
#15251=CARTESIAN_POINT('Ctrl Pts',(-7.55182125346563,17.6179818599248,0.));
#15252=CARTESIAN_POINT('Ctrl Pts',(-7.55182125346563,17.6179818599248,21.));
#15253=CARTESIAN_POINT('Ctrl Pts',(-7.54158441095317,17.5715579419204,0.));
#15254=CARTESIAN_POINT('Ctrl Pts',(-7.54158441095317,17.5715579419204,21.));
#15255=CARTESIAN_POINT('Ctrl Pts',(-7.53103903007863,17.5252518287336,0.));
#15256=CARTESIAN_POINT('Ctrl Pts',(-7.53103903007863,17.5252518287336,21.));
#15257=CARTESIAN_POINT('Ctrl Pts',(-7.52019696747328,17.4790653226646,0.));
#15258=CARTESIAN_POINT('Ctrl Pts',(-7.52019696747328,17.4790653226646,21.));
#15259=CARTESIAN_POINT('Ctrl Pts',(-7.50891486634214,17.4330545448126,0.));
#15260=CARTESIAN_POINT('Ctrl Pts',(-7.50891486634214,17.4330545448126,21.));
#15261=CARTESIAN_POINT('Ctrl Pts',(-7.4968177445175,17.3873563447297,0.));
#15262=CARTESIAN_POINT('Ctrl Pts',(-7.4968177445175,17.3873563447297,21.));
#15263=CARTESIAN_POINT('Ctrl Pts',(-7.48340100912745,17.3421522689127,0.));
#15264=CARTESIAN_POINT('Ctrl Pts',(-7.48340100912745,17.3421522689127,21.));
#15265=CARTESIAN_POINT('Ctrl Pts',(-7.47120323460919,17.3065305096784,0.));
#15266=CARTESIAN_POINT('Ctrl Pts',(-7.47120323460919,17.3065305096784,21.));
#15267=CARTESIAN_POINT('Ctrl Pts',(-7.4610504981825,17.2801832097582,0.));
#15268=CARTESIAN_POINT('Ctrl Pts',(-7.4610504981825,17.2801832097582,21.));
#15269=CARTESIAN_POINT('Ctrl Pts',(-7.45381253347183,17.2627905583523,0.));
#15270=CARTESIAN_POINT('Ctrl Pts',(-7.45381253347183,17.2627905583523,21.));
#15271=CARTESIAN_POINT('Ctrl Pts',(-7.45007618140238,17.2541372868972,0.));
#15272=CARTESIAN_POINT('Ctrl Pts',(-7.45007618140238,17.2541372868972,21.));
#15273=CARTESIAN_POINT('',(-7.45574324794407,20.698113262342,0.));
#15274=CARTESIAN_POINT('Ctrl Pts',(-7.45007618140238,17.2541372868972,0.));
#15275=CARTESIAN_POINT('Ctrl Pts',(-7.45381253347183,17.2627905583523,0.));
#15276=CARTESIAN_POINT('Ctrl Pts',(-7.4610504981825,17.2801832097582,0.));
#15277=CARTESIAN_POINT('Ctrl Pts',(-7.47120323460919,17.3065305096784,0.));
#15278=CARTESIAN_POINT('Ctrl Pts',(-7.48340100912745,17.3421522689127,0.));
#15279=CARTESIAN_POINT('Ctrl Pts',(-7.4968177445175,17.3873563447297,0.));
#15280=CARTESIAN_POINT('Ctrl Pts',(-7.50891486634214,17.4330545448126,0.));
#15281=CARTESIAN_POINT('Ctrl Pts',(-7.52019696747328,17.4790653226646,0.));
#15282=CARTESIAN_POINT('Ctrl Pts',(-7.53103903007863,17.5252518287336,0.));
#15283=CARTESIAN_POINT('Ctrl Pts',(-7.54158441095317,17.5715579419204,0.));
#15284=CARTESIAN_POINT('Ctrl Pts',(-7.55182125346563,17.6179818599248,0.));
#15285=CARTESIAN_POINT('Ctrl Pts',(-7.56164400295862,17.6645549117314,0.));
#15286=CARTESIAN_POINT('Ctrl Pts',(-7.57091795530423,17.7113192869136,0.));
#15287=CARTESIAN_POINT('Ctrl Pts',(-7.57954834582803,17.7583042294209,0.));
#15288=CARTESIAN_POINT('Ctrl Pts',(-7.58752955799499,17.8055090348024,0.));
#15289=CARTESIAN_POINT('Ctrl Pts',(-7.59491004201955,17.8529149331931,0.));
#15290=CARTESIAN_POINT('Ctrl Pts',(-7.60176928403058,17.900492838997,0.));
#15291=CARTESIAN_POINT('Ctrl Pts',(-7.60819152580111,17.9482122228183,0.));
#15292=CARTESIAN_POINT('Ctrl Pts',(-7.61423755067037,17.9960506269561,0.));
#15293=CARTESIAN_POINT('Ctrl Pts',(-7.61992799636654,18.0439992897906,0.));
#15294=CARTESIAN_POINT('Ctrl Pts',(-7.62525915358073,18.0920577897363,0.));
#15295=CARTESIAN_POINT('Ctrl Pts',(-7.63021285851761,18.1402306858819,0.));
#15296=CARTESIAN_POINT('Ctrl Pts',(-7.63476798969016,18.1885236169197,0.));
#15297=CARTESIAN_POINT('Ctrl Pts',(-7.63891299603826,18.2369390502576,0.));
#15298=CARTESIAN_POINT('Ctrl Pts',(-7.6426522027076,18.2854741391282,0.));
#15299=CARTESIAN_POINT('Ctrl Pts',(-7.64599903846601,18.3341230095852,0.));
#15300=CARTESIAN_POINT('Ctrl Pts',(-7.6489719793775,18.3828781275628,0.));
#15301=CARTESIAN_POINT('Ctrl Pts',(-7.65158974829126,18.4317319183719,0.));
#15302=CARTESIAN_POINT('Ctrl Pts',(-7.65386603444742,18.4806785483052,0.));
#15303=CARTESIAN_POINT('Ctrl Pts',(-7.65580722110436,18.5297146894905,0.));
#15304=CARTESIAN_POINT('Ctrl Pts',(-7.65741532450727,18.5788385228928,0.));
#15305=CARTESIAN_POINT('Ctrl Pts',(-7.65868976978872,18.6280491346907,0.));
#15306=CARTESIAN_POINT('Ctrl Pts',(-7.65962948375621,18.6773458057584,0.));
#15307=CARTESIAN_POINT('Ctrl Pts',(-7.66023521705904,18.7267272235231,0.));
#15308=CARTESIAN_POINT('Ctrl Pts',(-7.6605104692254,18.7761911671591,0.));
#15309=CARTESIAN_POINT('Ctrl Pts',(-7.66046025294774,18.8257349246207,0.));
#15310=CARTESIAN_POINT('Ctrl Pts',(-7.66009036321663,18.8753555389435,0.));
#15311=CARTESIAN_POINT('Ctrl Pts',(-7.65940650980098,18.9250501008887,0.));
#15312=CARTESIAN_POINT('Ctrl Pts',(-7.65841335587266,18.974816073814,0.));
#15313=CARTESIAN_POINT('Ctrl Pts',(-7.65711415727855,19.0246514144531,0.));
#15314=CARTESIAN_POINT('Ctrl Pts',(-7.65551129907201,19.0745543888799,0.));
#15315=CARTESIAN_POINT('Ctrl Pts',(-7.65360662280609,19.1245234597312,0.));
#15316=CARTESIAN_POINT('Ctrl Pts',(-7.65140181220525,19.1745571539291,0.));
#15317=CARTESIAN_POINT('Ctrl Pts',(-7.64889882291923,19.224653915265,0.));
#15318=CARTESIAN_POINT('Ctrl Pts',(-7.64610005549613,19.2748120456486,0.));
#15319=CARTESIAN_POINT('Ctrl Pts',(-7.64300812875338,19.3250297839295,0.));
#15320=CARTESIAN_POINT('Ctrl Pts',(-7.6396257482276,19.3753053524647,0.));
#15321=CARTESIAN_POINT('Ctrl Pts',(-7.63595554930654,19.4256370121006,0.));
#15322=CARTESIAN_POINT('Ctrl Pts',(-7.63199992715365,19.4760231231881,0.));
#15323=CARTESIAN_POINT('Ctrl Pts',(-7.62776096538882,19.5264621687521,0.));
#15324=CARTESIAN_POINT('Ctrl Pts',(-7.62324053735219,19.5769527121826,0.));
#15325=CARTESIAN_POINT('Ctrl Pts',(-7.6184403707059,19.6274933688524,0.));
#15326=CARTESIAN_POINT('Ctrl Pts',(-7.61336212350879,19.6780827744426,0.));
#15327=CARTESIAN_POINT('Ctrl Pts',(-7.60800746969261,19.7287195480601,0.));
#15328=CARTESIAN_POINT('Ctrl Pts',(-7.60237814110186,19.7794022782484,0.));
#15329=CARTESIAN_POINT('Ctrl Pts',(-7.59647587605448,19.830129556152,0.));
#15330=CARTESIAN_POINT('Ctrl Pts',(-7.59030238888852,19.8808999994024,0.));
#15331=CARTESIAN_POINT('Ctrl Pts',(-7.58385933533351,19.931712276832,0.));
#15332=CARTESIAN_POINT('Ctrl Pts',(-7.57714827622806,19.9825651387294,0.));
#15333=CARTESIAN_POINT('Ctrl Pts',(-7.57017066105973,20.0334574248556,0.));
#15334=CARTESIAN_POINT('Ctrl Pts',(-7.5629278654946,20.0843880130978,0.));
#15335=CARTESIAN_POINT('Ctrl Pts',(-7.55542122125494,20.1353557774357,0.));
#15336=CARTESIAN_POINT('Ctrl Pts',(-7.54765204869254,20.1863595454674,0.));
#15337=CARTESIAN_POINT('Ctrl Pts',(-7.53962169534166,20.2373980474879,0.));
#15338=CARTESIAN_POINT('Ctrl Pts',(-7.53133155804007,20.2884698940944,0.));
#15339=CARTESIAN_POINT('Ctrl Pts',(-7.52278303006887,20.3395736743243,0.));
#15340=CARTESIAN_POINT('Ctrl Pts',(-7.51397746081993,20.3907080367098,0.));
#15341=CARTESIAN_POINT('Ctrl Pts',(-7.50491611266253,20.4418717748497,0.));
#15342=CARTESIAN_POINT('Ctrl Pts',(-7.49560012018405,20.4930639156161,0.));
#15343=CARTESIAN_POINT('Ctrl Pts',(-7.48411651832412,20.5545277683621,0.));
#15344=CARTESIAN_POINT('Ctrl Pts',(-7.47423073598681,20.6057817877246,0.));
#15345=CARTESIAN_POINT('Ctrl Pts',(-7.46612041736313,20.6468066077586,0.));
#15346=CARTESIAN_POINT('Ctrl Pts',(-7.45992433946823,20.6775873630604,0.));
#15347=CARTESIAN_POINT('Ctrl Pts',(-7.45574324794401,20.698113262342,0.));
#15348=CARTESIAN_POINT('',(-7.45574324794407,20.698113262342,13.));
#15349=CARTESIAN_POINT('Ctrl Pts',(-7.45574324794401,20.698113262342,13.));
#15350=CARTESIAN_POINT('Ctrl Pts',(-7.47632490128082,20.5970733922996,13.));
#15351=CARTESIAN_POINT('Ctrl Pts',(-7.49544541996018,20.4961877827456,13.));
#15352=CARTESIAN_POINT('Ctrl Pts',(-7.51308219880446,20.3954689810171,13.));
#15353=CARTESIAN_POINT('Ctrl Pts',(-7.54230710697449,20.2285735542786,13.));
#15354=CARTESIAN_POINT('Ctrl Pts',(-7.56745095717373,20.062147728883,13.));
#15355=CARTESIAN_POINT('Ctrl Pts',(-7.58830059932795,19.8963869101261,13.));
#15356=CARTESIAN_POINT('Ctrl Pts',(-7.60432685704092,19.7689734235799,13.));
#15357=CARTESIAN_POINT('Ctrl Pts',(-7.61781485448689,19.6419503916105,13.));
#15358=CARTESIAN_POINT('Ctrl Pts',(-7.62864367953763,19.5154161616707,13.));
#15359=CARTESIAN_POINT('Ctrl Pts',(-7.6403006489712,19.3792051097978,13.));
#15360=CARTESIAN_POINT('Ctrl Pts',(-7.64888186442765,19.2435576430979,13.));
#15361=CARTESIAN_POINT('Ctrl Pts',(-7.65417053744727,19.1086228829228,13.));
#15362=CARTESIAN_POINT('Ctrl Pts',(-7.6570984904302,19.0339193359104,13.));
#15363=CARTESIAN_POINT('Ctrl Pts',(-7.65902218172414,18.9594327317773,13.));
#15364=CARTESIAN_POINT('Ctrl Pts',(-7.65990167998771,18.8851905412181,13.));
#15365=CARTESIAN_POINT('Ctrl Pts',(-7.66074919903711,18.813647852193,13.));
#15366=CARTESIAN_POINT('Ctrl Pts',(-7.66062065571968,18.742334282715,13.));
#15367=CARTESIAN_POINT('Ctrl Pts',(-7.65944821270105,18.6712863090353,13.));
#15368=CARTESIAN_POINT('Ctrl Pts',(-7.65843486239238,18.6098790722535,13.));
#15369=CARTESIAN_POINT('Ctrl Pts',(-7.65664478982501,18.5486691992234,13.));
#15370=CARTESIAN_POINT('Ctrl Pts',(-7.65407864070033,18.4876659850186,13.));
#15371=CARTESIAN_POINT('Ctrl Pts',(-7.6522370315783,18.4438867382584,13.));
#15372=CARTESIAN_POINT('Ctrl Pts',(-7.64999840197637,18.4002130327903,13.));
#15373=CARTESIAN_POINT('Ctrl Pts',(-7.64732656562888,18.3566609384397,13.));
#15374=CARTESIAN_POINT('Ctrl Pts',(-7.64469823681671,18.3138180358347,13.));
#15375=CARTESIAN_POINT('Ctrl Pts',(-7.64164464440333,18.2710948573601,13.));
#15376=CARTESIAN_POINT('Ctrl Pts',(-7.63811742044703,18.2285117408546,13.));
#15377=CARTESIAN_POINT('Ctrl Pts',(-7.63505911004952,18.1915896770503,13.));
#15378=CARTESIAN_POINT('Ctrl Pts',(-7.63164238136491,18.154773706468,13.));
#15379=CARTESIAN_POINT('Ctrl Pts',(-7.62788266166224,18.1180614604547,13.));
#15380=CARTESIAN_POINT('Ctrl Pts',(-7.62447721821964,18.0848085886088,13.));
#15381=CARTESIAN_POINT('Ctrl Pts',(-7.6207956490075,18.0516390296698,13.));
#15382=CARTESIAN_POINT('Ctrl Pts',(-7.61686093607981,18.0185473585012,13.));
#15383=CARTESIAN_POINT('Ctrl Pts',(-7.61354654175259,17.9906726827078,13.));
#15384=CARTESIAN_POINT('Ctrl Pts',(-7.6100541756254,17.9628527174308,13.));
#15385=CARTESIAN_POINT('Ctrl Pts',(-7.60636550501162,17.9350952313316,13.));
#15386=CARTESIAN_POINT('Ctrl Pts',(-7.60102759729446,17.8949271288438,13.));
#15387=CARTESIAN_POINT('Ctrl Pts',(-7.59527782596713,17.8548900767291,13.));
#15388=CARTESIAN_POINT('Ctrl Pts',(-7.58891067825601,17.8150590779502,13.));
#15389=CARTESIAN_POINT('Ctrl Pts',(-7.58506340059149,17.7909916432194,13.));
#15390=CARTESIAN_POINT('Ctrl Pts',(-7.58098742039303,17.7670005717874,13.));
#15391=CARTESIAN_POINT('Ctrl Pts',(-7.5766581762109,17.7430955913527,13.));
#15392=CARTESIAN_POINT('Ctrl Pts',(-7.57266539518276,17.7210484745022,13.));
#15393=CARTESIAN_POINT('Ctrl Pts',(-7.56845593268005,17.6990750118723,13.));
#15394=CARTESIAN_POINT('Ctrl Pts',(-7.56405390354134,17.677168309438,13.));
#15395=CARTESIAN_POINT('Ctrl Pts',(-7.5579984663457,17.6470334201461,13.));
#15396=CARTESIAN_POINT('Ctrl Pts',(-7.5515855270709,17.617022406593,13.));
#15397=CARTESIAN_POINT('Ctrl Pts',(-7.54495919885966,17.5870909089508,13.));
#15398=CARTESIAN_POINT('Ctrl Pts',(-7.54075533804246,17.5681018329307,13.));
#15399=CARTESIAN_POINT('Ctrl Pts',(-7.53646718585994,17.5491442491042,13.));
#15400=CARTESIAN_POINT('Ctrl Pts',(-7.53210330803509,17.5302169633315,13.));
#15401=CARTESIAN_POINT('Ctrl Pts',(-7.52818693080709,17.5132306053344,13.));
#15402=CARTESIAN_POINT('Ctrl Pts',(-7.5242102522165,17.4962684161094,13.));
#15403=CARTESIAN_POINT('Ctrl Pts',(-7.52014106530733,17.4793429835295,13.));
#15404=CARTESIAN_POINT('Ctrl Pts',(-7.51586353943748,17.4615509829812,13.));
#15405=CARTESIAN_POINT('Ctrl Pts',(-7.51148394209978,17.4437995539472,13.));
#15406=CARTESIAN_POINT('Ctrl Pts',(-7.50690601561094,17.4261238143268,13.));
#15407=CARTESIAN_POINT('Ctrl Pts',(-7.4993020898442,17.3967644499347,13.));
#15408=CARTESIAN_POINT('Ctrl Pts',(-7.49114308214025,17.3676168188904,13.));
#15409=CARTESIAN_POINT('Ctrl Pts',(-7.4818397562212,17.3388922514977,13.));
#15410=CARTESIAN_POINT('Ctrl Pts',(-7.47670957121237,17.3230525027557,13.));
#15411=CARTESIAN_POINT('Ctrl Pts',(-7.47123011545034,17.3073418194582,13.));
#15412=CARTESIAN_POINT('Ctrl Pts',(-7.46532888197675,17.2917860605643,13.));
#15413=CARTESIAN_POINT('Ctrl Pts',(-7.46052853290803,17.279132253008,13.));
#15414=CARTESIAN_POINT('Ctrl Pts',(-7.45544915949044,17.2665809316753,13.));
#15415=CARTESIAN_POINT('Ctrl Pts',(-7.45007618140238,17.2541372868972,13.));
#15416=CARTESIAN_POINT('',(-7.45574324794407,20.698113262342,0.));
#15417=CARTESIAN_POINT('Origin',(-1.75106900012182E-12,5.38923623413286E-12,
0.));
#15418=CARTESIAN_POINT('',(-6.1342227326009,21.1275013067528,0.));
#15419=CARTESIAN_POINT('Origin',(-1.75106900012182E-12,5.38923623413286E-12,
0.));
#15420=CARTESIAN_POINT('',(-6.1342227326009,21.1275013067528,13.));
#15421=CARTESIAN_POINT('Origin',(-1.75106900012182E-12,5.38923623413286E-12,
13.));
#15422=CARTESIAN_POINT('',(-6.1342227326009,21.1275013067528,0.));
#15423=CARTESIAN_POINT('Ctrl Pts',(-4.1144891981253,18.337935196262,0.));
#15424=CARTESIAN_POINT('Ctrl Pts',(-4.1144891981253,18.337935196262,21.));
#15425=CARTESIAN_POINT('Ctrl Pts',(-4.11655269114951,18.3471320125699,0.));
#15426=CARTESIAN_POINT('Ctrl Pts',(-4.11655269114951,18.3471320125699,21.));
#15427=CARTESIAN_POINT('Ctrl Pts',(-4.12092019868859,18.3654573320481,0.));
#15428=CARTESIAN_POINT('Ctrl Pts',(-4.12092019868859,18.3654573320481,21.));
#15429=CARTESIAN_POINT('Ctrl Pts',(-4.12819301671078,18.3927403741815,0.));
#15430=CARTESIAN_POINT('Ctrl Pts',(-4.12819301671078,18.3927403741815,21.));
#15431=CARTESIAN_POINT('Ctrl Pts',(-4.13926275457062,18.4287286547442,0.));
#15432=CARTESIAN_POINT('Ctrl Pts',(-4.13926275457062,18.4287286547442,21.));
#15433=CARTESIAN_POINT('Ctrl Pts',(-4.15497867673974,18.4731856794913,0.));
#15434=CARTESIAN_POINT('Ctrl Pts',(-4.15497867673974,18.4731856794913,21.));
#15435=CARTESIAN_POINT('Ctrl Pts',(-4.17205262766561,18.5172668097744,0.));
#15436=CARTESIAN_POINT('Ctrl Pts',(-4.17205262766561,18.5172668097744,21.));
#15437=CARTESIAN_POINT('Ctrl Pts',(-4.1899696727862,18.5611217636409,0.));
#15438=CARTESIAN_POINT('Ctrl Pts',(-4.1899696727862,18.5611217636409,21.));
#15439=CARTESIAN_POINT('Ctrl Pts',(-4.20834600700664,18.6048602364653,0.));
#15440=CARTESIAN_POINT('Ctrl Pts',(-4.20834600700664,18.6048602364653,21.));
#15441=CARTESIAN_POINT('Ctrl Pts',(-4.22703266508918,18.6485210883348,0.));
#15442=CARTESIAN_POINT('Ctrl Pts',(-4.22703266508918,18.6485210883348,21.));
#15443=CARTESIAN_POINT('Ctrl Pts',(-4.24603817988452,18.6920958920047,0.));
#15444=CARTESIAN_POINT('Ctrl Pts',(-4.24603817988452,18.6920958920047,21.));
#15445=CARTESIAN_POINT('Ctrl Pts',(-4.26546636161932,18.735547949685,0.));
#15446=CARTESIAN_POINT('Ctrl Pts',(-4.26546636161932,18.735547949685,21.));
#15447=CARTESIAN_POINT('Ctrl Pts',(-4.28545098663153,18.778832216358,0.));
#15448=CARTESIAN_POINT('Ctrl Pts',(-4.28545098663153,18.778832216358,21.));
#15449=CARTESIAN_POINT('Ctrl Pts',(-4.30608591031525,18.8219166495975,0.));
#15450=CARTESIAN_POINT('Ctrl Pts',(-4.30608591031525,18.8219166495975,21.));
#15451=CARTESIAN_POINT('Ctrl Pts',(-4.32737526247704,18.8647973781745,0.));
#15452=CARTESIAN_POINT('Ctrl Pts',(-4.32737526247704,18.8647973781745,21.));
#15453=CARTESIAN_POINT('Ctrl Pts',(-4.34926881342021,18.9074876952706,0.));
#15454=CARTESIAN_POINT('Ctrl Pts',(-4.34926881342021,18.9074876952706,21.));
#15455=CARTESIAN_POINT('Ctrl Pts',(-4.37168516143122,18.9500107909187,0.));
#15456=CARTESIAN_POINT('Ctrl Pts',(-4.37168516143122,18.9500107909187,21.));
#15457=CARTESIAN_POINT('Ctrl Pts',(-4.39453820875554,18.9923914823906,0.));
#15458=CARTESIAN_POINT('Ctrl Pts',(-4.39453820875554,18.9923914823906,21.));
#15459=CARTESIAN_POINT('Ctrl Pts',(-4.41776558033331,19.034647328575,0.));
#15460=CARTESIAN_POINT('Ctrl Pts',(-4.41776558033331,19.034647328575,21.));
#15461=CARTESIAN_POINT('Ctrl Pts',(-4.44134542994081,19.0767833717249,0.));
#15462=CARTESIAN_POINT('Ctrl Pts',(-4.44134542994081,19.0767833717249,21.));
#15463=CARTESIAN_POINT('Ctrl Pts',(-4.46528051067021,19.1187970904932,0.));
#15464=CARTESIAN_POINT('Ctrl Pts',(-4.46528051067021,19.1187970904932,21.));
#15465=CARTESIAN_POINT('Ctrl Pts',(-4.48958819710576,19.1606814968494,0.));
#15466=CARTESIAN_POINT('Ctrl Pts',(-4.48958819710576,19.1606814968494,21.));
#15467=CARTESIAN_POINT('Ctrl Pts',(-4.51428889122954,19.2024287376926,0.));
#15468=CARTESIAN_POINT('Ctrl Pts',(-4.51428889122954,19.2024287376926,21.));
#15469=CARTESIAN_POINT('Ctrl Pts',(-4.53939338835151,19.2440340196551,0.));
#15470=CARTESIAN_POINT('Ctrl Pts',(-4.53939338835151,19.2440340196551,21.));
#15471=CARTESIAN_POINT('Ctrl Pts',(-4.5648965160674,19.2854975819105,0.));
#15472=CARTESIAN_POINT('Ctrl Pts',(-4.5648965160674,19.2854975819105,21.));
#15473=CARTESIAN_POINT('Ctrl Pts',(-4.59078395765677,19.3268225655679,0.));
#15474=CARTESIAN_POINT('Ctrl Pts',(-4.59078395765677,19.3268225655679,21.));
#15475=CARTESIAN_POINT('Ctrl Pts',(-4.61703633725712,19.3680137353983,0.));
#15476=CARTESIAN_POINT('Ctrl Pts',(-4.61703633725712,19.3680137353983,21.));
#15477=CARTESIAN_POINT('Ctrl Pts',(-4.64363405547472,19.4090759683639,0.));
#15478=CARTESIAN_POINT('Ctrl Pts',(-4.64363405547472,19.4090759683639,21.));
#15479=CARTESIAN_POINT('Ctrl Pts',(-4.67056260851453,19.4500125912299,0.));
#15480=CARTESIAN_POINT('Ctrl Pts',(-4.67056260851453,19.4500125912299,21.));
#15481=CARTESIAN_POINT('Ctrl Pts',(-4.69781487613784,19.4908246636763,0.));
#15482=CARTESIAN_POINT('Ctrl Pts',(-4.69781487613784,19.4908246636763,21.));
#15483=CARTESIAN_POINT('Ctrl Pts',(-4.72538815796615,19.531511899192,0.));
#15484=CARTESIAN_POINT('Ctrl Pts',(-4.72538815796615,19.531511899192,21.));
#15485=CARTESIAN_POINT('Ctrl Pts',(-4.7532823819461,19.5720732205813,0.));
#15486=CARTESIAN_POINT('Ctrl Pts',(-4.7532823819461,19.5720732205813,21.));
#15487=CARTESIAN_POINT('Ctrl Pts',(-4.7814979936173,19.6125074152527,0.));
#15488=CARTESIAN_POINT('Ctrl Pts',(-4.7814979936173,19.6125074152527,21.));
#15489=CARTESIAN_POINT('Ctrl Pts',(-4.8100336141806,19.6528138625329,0.));
#15490=CARTESIAN_POINT('Ctrl Pts',(-4.8100336141806,19.6528138625329,21.));
#15491=CARTESIAN_POINT('Ctrl Pts',(-4.83888510708974,19.6929928227072,0.));
#15492=CARTESIAN_POINT('Ctrl Pts',(-4.83888510708974,19.6929928227072,21.));
#15493=CARTESIAN_POINT('Ctrl Pts',(-4.86804682289086,19.7330450480715,0.));
#15494=CARTESIAN_POINT('Ctrl Pts',(-4.86804682289086,19.7330450480715,21.));
#15495=CARTESIAN_POINT('Ctrl Pts',(-4.89751233527804,19.772971552601,0.));
#15496=CARTESIAN_POINT('Ctrl Pts',(-4.89751233527804,19.772971552601,21.));
#15497=CARTESIAN_POINT('Ctrl Pts',(-4.92727531494346,19.8127733387903,0.));
#15498=CARTESIAN_POINT('Ctrl Pts',(-4.92727531494346,19.8127733387903,21.));
#15499=CARTESIAN_POINT('Ctrl Pts',(-4.95733049830096,19.8524510953961,0.));
#15500=CARTESIAN_POINT('Ctrl Pts',(-4.95733049830096,19.8524510953961,21.));
#15501=CARTESIAN_POINT('Ctrl Pts',(-4.98767405031333,19.8920050831202,0.));
#15502=CARTESIAN_POINT('Ctrl Pts',(-4.98767405031333,19.8920050831202,21.));
#15503=CARTESIAN_POINT('Ctrl Pts',(-5.01830302225557,19.931435301086,0.));
#15504=CARTESIAN_POINT('Ctrl Pts',(-5.01830302225557,19.931435301086,21.));
#15505=CARTESIAN_POINT('Ctrl Pts',(-5.04921502064063,19.9707415879783,0.));
#15506=CARTESIAN_POINT('Ctrl Pts',(-5.04921502064063,19.9707415879783,21.));
#15507=CARTESIAN_POINT('Ctrl Pts',(-5.08040781745336,20.0099237417205,0.));
#15508=CARTESIAN_POINT('Ctrl Pts',(-5.08040781745336,20.0099237417205,21.));
#15509=CARTESIAN_POINT('Ctrl Pts',(-5.11187891582334,20.0489816528155,0.));
#15510=CARTESIAN_POINT('Ctrl Pts',(-5.11187891582334,20.0489816528155,21.));
#15511=CARTESIAN_POINT('Ctrl Pts',(-5.14362537555397,20.087915358486,0.));
#15512=CARTESIAN_POINT('Ctrl Pts',(-5.14362537555397,20.087915358486,21.));
#15513=CARTESIAN_POINT('Ctrl Pts',(-5.17564404279921,20.1267249732337,0.));
#15514=CARTESIAN_POINT('Ctrl Pts',(-5.17564404279921,20.1267249732337,21.));
#15515=CARTESIAN_POINT('Ctrl Pts',(-5.20793168386163,20.1654106491899,0.));
#15516=CARTESIAN_POINT('Ctrl Pts',(-5.20793168386163,20.1654106491899,21.));
#15517=CARTESIAN_POINT('Ctrl Pts',(-5.2404851444189,20.2039725283917,0.));
#15518=CARTESIAN_POINT('Ctrl Pts',(-5.2404851444189,20.2039725283917,21.));
#15519=CARTESIAN_POINT('Ctrl Pts',(-5.2733015229815,20.2424106921768,0.));
#15520=CARTESIAN_POINT('Ctrl Pts',(-5.2733015229815,20.2424106921768,21.));
#15521=CARTESIAN_POINT('Ctrl Pts',(-5.30637824220997,20.2807251380077,0.));
#15522=CARTESIAN_POINT('Ctrl Pts',(-5.30637824220997,20.2807251380077,21.));
#15523=CARTESIAN_POINT('Ctrl Pts',(-5.33971294212213,20.3189158047642,0.));
#15524=CARTESIAN_POINT('Ctrl Pts',(-5.33971294212213,20.3189158047642,21.));
#15525=CARTESIAN_POINT('Ctrl Pts',(-5.37330341114649,20.3569825877537,0.));
#15526=CARTESIAN_POINT('Ctrl Pts',(-5.37330341114649,20.3569825877537,21.));
#15527=CARTESIAN_POINT('Ctrl Pts',(-5.40714750595875,20.3949253578015,0.));
#15528=CARTESIAN_POINT('Ctrl Pts',(-5.40714750595875,20.3949253578015,21.));
#15529=CARTESIAN_POINT('Ctrl Pts',(-5.44124306065111,20.4327439816542,0.));
#15530=CARTESIAN_POINT('Ctrl Pts',(-5.44124306065111,20.4327439816542,21.));
#15531=CARTESIAN_POINT('Ctrl Pts',(-5.4755878444985,20.4704383353718,0.));
#15532=CARTESIAN_POINT('Ctrl Pts',(-5.4755878444985,20.4704383353718,21.));
#15533=CARTESIAN_POINT('Ctrl Pts',(-5.51017962306782,20.5080083009242,0.));
#15534=CARTESIAN_POINT('Ctrl Pts',(-5.51017962306782,20.5080083009242,21.));
#15535=CARTESIAN_POINT('Ctrl Pts',(-5.5450161968946,20.5454537676144,0.));
#15536=CARTESIAN_POINT('Ctrl Pts',(-5.5450161968946,20.5454537676144,21.));
#15537=CARTESIAN_POINT('Ctrl Pts',(-5.58009544402475,20.5827746317185,0.));
#15538=CARTESIAN_POINT('Ctrl Pts',(-5.58009544402475,20.5827746317185,21.));
#15539=CARTESIAN_POINT('Ctrl Pts',(-5.61541536715149,20.6199707996366,0.));
#15540=CARTESIAN_POINT('Ctrl Pts',(-5.61541536715149,20.6199707996366,21.));
#15541=CARTESIAN_POINT('Ctrl Pts',(-5.65097411164334,20.6570421847033,0.));
#15542=CARTESIAN_POINT('Ctrl Pts',(-5.65097411164334,20.6570421847033,21.));
#15543=CARTESIAN_POINT('Ctrl Pts',(-5.68676990500163,20.6939886877061,0.));
#15544=CARTESIAN_POINT('Ctrl Pts',(-5.68676990500163,20.6939886877061,21.));
#15545=CARTESIAN_POINT('Ctrl Pts',(-5.72280100798241,20.7308101804425,0.));
#15546=CARTESIAN_POINT('Ctrl Pts',(-5.72280100798241,20.7308101804425,21.));
#15547=CARTESIAN_POINT('Ctrl Pts',(-5.75906566327796,20.7675064905026,0.));
#15548=CARTESIAN_POINT('Ctrl Pts',(-5.75906566327796,20.7675064905026,21.));
#15549=CARTESIAN_POINT('Ctrl Pts',(-5.79556203439644,20.8040773827343,0.));
#15550=CARTESIAN_POINT('Ctrl Pts',(-5.79556203439644,20.8040773827343,21.));
#15551=CARTESIAN_POINT('Ctrl Pts',(-5.83228817460177,20.8405225541277,0.));
#15552=CARTESIAN_POINT('Ctrl Pts',(-5.83228817460177,20.8405225541277,21.));
#15553=CARTESIAN_POINT('Ctrl Pts',(-5.86924212736287,20.8768416821402,0.));
#15554=CARTESIAN_POINT('Ctrl Pts',(-5.86924212736287,20.8768416821402,21.));
#15555=CARTESIAN_POINT('Ctrl Pts',(-5.90642200662599,20.9130344665641,0.));
#15556=CARTESIAN_POINT('Ctrl Pts',(-5.90642200662599,20.9130344665641,21.));
#15557=CARTESIAN_POINT('Ctrl Pts',(-5.94382608200804,20.9491006734021,0.));
#15558=CARTESIAN_POINT('Ctrl Pts',(-5.94382608200804,20.9491006734021,21.));
#15559=CARTESIAN_POINT('Ctrl Pts',(-5.98145286361836,20.9850401822713,0.));
#15560=CARTESIAN_POINT('Ctrl Pts',(-5.98145286361836,20.9850401822713,21.));
#15561=CARTESIAN_POINT('Ctrl Pts',(-6.01930117633044,21.0208530236003,0.));
#15562=CARTESIAN_POINT('Ctrl Pts',(-6.01930117633044,21.0208530236003,21.));
#15563=CARTESIAN_POINT('Ctrl Pts',(-6.05737013696532,21.0565393163693,0.));
#15564=CARTESIAN_POINT('Ctrl Pts',(-6.05737013696532,21.0565393163693,21.));
#15565=CARTESIAN_POINT('Ctrl Pts',(-6.08800133883114,21.0849872356853,0.));
#15566=CARTESIAN_POINT('Ctrl Pts',(-6.08800133883114,21.0849872356853,21.));
#15567=CARTESIAN_POINT('Ctrl Pts',(-6.11107360216958,21.1062663590356,0.));
#15568=CARTESIAN_POINT('Ctrl Pts',(-6.11107360216958,21.1062663590356,21.));
#15569=CARTESIAN_POINT('Ctrl Pts',(-6.12649903511517,21.1204271980506,0.));
#15570=CARTESIAN_POINT('Ctrl Pts',(-6.12649903511517,21.1204271980506,21.));
#15571=CARTESIAN_POINT('Ctrl Pts',(-6.1342227326009,21.1275013067528,0.));
#15572=CARTESIAN_POINT('Ctrl Pts',(-6.1342227326009,21.1275013067528,21.));
#15573=CARTESIAN_POINT('Ctrl Pts',(-4.1144891981253,18.337935196262,0.));
#15574=CARTESIAN_POINT('Ctrl Pts',(-4.11655269114951,18.3471320125699,0.));
#15575=CARTESIAN_POINT('Ctrl Pts',(-4.12092019868859,18.3654573320481,0.));
#15576=CARTESIAN_POINT('Ctrl Pts',(-4.12819301671078,18.3927403741815,0.));
#15577=CARTESIAN_POINT('Ctrl Pts',(-4.13926275457062,18.4287286547442,0.));
#15578=CARTESIAN_POINT('Ctrl Pts',(-4.15497867673974,18.4731856794913,0.));
#15579=CARTESIAN_POINT('Ctrl Pts',(-4.17205262766561,18.5172668097744,0.));
#15580=CARTESIAN_POINT('Ctrl Pts',(-4.1899696727862,18.5611217636409,0.));
#15581=CARTESIAN_POINT('Ctrl Pts',(-4.20834600700664,18.6048602364653,0.));
#15582=CARTESIAN_POINT('Ctrl Pts',(-4.22703266508918,18.6485210883348,0.));
#15583=CARTESIAN_POINT('Ctrl Pts',(-4.24603817988452,18.6920958920047,0.));
#15584=CARTESIAN_POINT('Ctrl Pts',(-4.26546636161932,18.735547949685,0.));
#15585=CARTESIAN_POINT('Ctrl Pts',(-4.28545098663153,18.778832216358,0.));
#15586=CARTESIAN_POINT('Ctrl Pts',(-4.30608591031525,18.8219166495975,0.));
#15587=CARTESIAN_POINT('Ctrl Pts',(-4.32737526247704,18.8647973781745,0.));
#15588=CARTESIAN_POINT('Ctrl Pts',(-4.34926881342021,18.9074876952706,0.));
#15589=CARTESIAN_POINT('Ctrl Pts',(-4.37168516143122,18.9500107909187,0.));
#15590=CARTESIAN_POINT('Ctrl Pts',(-4.39453820875554,18.9923914823906,0.));
#15591=CARTESIAN_POINT('Ctrl Pts',(-4.41776558033331,19.034647328575,0.));
#15592=CARTESIAN_POINT('Ctrl Pts',(-4.44134542994081,19.0767833717249,0.));
#15593=CARTESIAN_POINT('Ctrl Pts',(-4.46528051067021,19.1187970904932,0.));
#15594=CARTESIAN_POINT('Ctrl Pts',(-4.48958819710576,19.1606814968494,0.));
#15595=CARTESIAN_POINT('Ctrl Pts',(-4.51428889122954,19.2024287376926,0.));
#15596=CARTESIAN_POINT('Ctrl Pts',(-4.53939338835151,19.2440340196551,0.));
#15597=CARTESIAN_POINT('Ctrl Pts',(-4.5648965160674,19.2854975819105,0.));
#15598=CARTESIAN_POINT('Ctrl Pts',(-4.59078395765677,19.3268225655679,0.));
#15599=CARTESIAN_POINT('Ctrl Pts',(-4.61703633725712,19.3680137353983,0.));
#15600=CARTESIAN_POINT('Ctrl Pts',(-4.64363405547472,19.4090759683639,0.));
#15601=CARTESIAN_POINT('Ctrl Pts',(-4.67056260851453,19.4500125912299,0.));
#15602=CARTESIAN_POINT('Ctrl Pts',(-4.69781487613784,19.4908246636763,0.));
#15603=CARTESIAN_POINT('Ctrl Pts',(-4.72538815796615,19.531511899192,0.));
#15604=CARTESIAN_POINT('Ctrl Pts',(-4.7532823819461,19.5720732205813,0.));
#15605=CARTESIAN_POINT('Ctrl Pts',(-4.7814979936173,19.6125074152527,0.));
#15606=CARTESIAN_POINT('Ctrl Pts',(-4.8100336141806,19.6528138625329,0.));
#15607=CARTESIAN_POINT('Ctrl Pts',(-4.83888510708974,19.6929928227072,0.));
#15608=CARTESIAN_POINT('Ctrl Pts',(-4.86804682289086,19.7330450480715,0.));
#15609=CARTESIAN_POINT('Ctrl Pts',(-4.89751233527804,19.772971552601,0.));
#15610=CARTESIAN_POINT('Ctrl Pts',(-4.92727531494346,19.8127733387903,0.));
#15611=CARTESIAN_POINT('Ctrl Pts',(-4.95733049830096,19.8524510953961,0.));
#15612=CARTESIAN_POINT('Ctrl Pts',(-4.98767405031333,19.8920050831202,0.));
#15613=CARTESIAN_POINT('Ctrl Pts',(-5.01830302225557,19.931435301086,0.));
#15614=CARTESIAN_POINT('Ctrl Pts',(-5.04921502064063,19.9707415879783,0.));
#15615=CARTESIAN_POINT('Ctrl Pts',(-5.08040781745336,20.0099237417205,0.));
#15616=CARTESIAN_POINT('Ctrl Pts',(-5.11187891582334,20.0489816528155,0.));
#15617=CARTESIAN_POINT('Ctrl Pts',(-5.14362537555397,20.087915358486,0.));
#15618=CARTESIAN_POINT('Ctrl Pts',(-5.17564404279921,20.1267249732337,0.));
#15619=CARTESIAN_POINT('Ctrl Pts',(-5.20793168386163,20.1654106491899,0.));
#15620=CARTESIAN_POINT('Ctrl Pts',(-5.2404851444189,20.2039725283917,0.));
#15621=CARTESIAN_POINT('Ctrl Pts',(-5.2733015229815,20.2424106921768,0.));
#15622=CARTESIAN_POINT('Ctrl Pts',(-5.30637824220997,20.2807251380077,0.));
#15623=CARTESIAN_POINT('Ctrl Pts',(-5.33971294212213,20.3189158047642,0.));
#15624=CARTESIAN_POINT('Ctrl Pts',(-5.37330341114649,20.3569825877537,0.));
#15625=CARTESIAN_POINT('Ctrl Pts',(-5.40714750595875,20.3949253578015,0.));
#15626=CARTESIAN_POINT('Ctrl Pts',(-5.44124306065111,20.4327439816542,0.));
#15627=CARTESIAN_POINT('Ctrl Pts',(-5.4755878444985,20.4704383353718,0.));
#15628=CARTESIAN_POINT('Ctrl Pts',(-5.51017962306782,20.5080083009242,0.));
#15629=CARTESIAN_POINT('Ctrl Pts',(-5.5450161968946,20.5454537676144,0.));
#15630=CARTESIAN_POINT('Ctrl Pts',(-5.58009544402475,20.5827746317185,0.));
#15631=CARTESIAN_POINT('Ctrl Pts',(-5.61541536715149,20.6199707996366,0.));
#15632=CARTESIAN_POINT('Ctrl Pts',(-5.65097411164334,20.6570421847033,0.));
#15633=CARTESIAN_POINT('Ctrl Pts',(-5.68676990500163,20.6939886877061,0.));
#15634=CARTESIAN_POINT('Ctrl Pts',(-5.72280100798241,20.7308101804425,0.));
#15635=CARTESIAN_POINT('Ctrl Pts',(-5.75906566327796,20.7675064905026,0.));
#15636=CARTESIAN_POINT('Ctrl Pts',(-5.79556203439644,20.8040773827343,0.));
#15637=CARTESIAN_POINT('Ctrl Pts',(-5.83228817460177,20.8405225541277,0.));
#15638=CARTESIAN_POINT('Ctrl Pts',(-5.86924212736287,20.8768416821402,0.));
#15639=CARTESIAN_POINT('Ctrl Pts',(-5.90642200662599,20.9130344665641,0.));
#15640=CARTESIAN_POINT('Ctrl Pts',(-5.94382608200804,20.9491006734021,0.));
#15641=CARTESIAN_POINT('Ctrl Pts',(-5.98145286361836,20.9850401822713,0.));
#15642=CARTESIAN_POINT('Ctrl Pts',(-6.02687083887286,21.0280155918661,0.));
#15643=CARTESIAN_POINT('Ctrl Pts',(-6.06499496148844,21.0636702474951,0.));
#15644=CARTESIAN_POINT('Ctrl Pts',(-6.09567013127871,21.0920928984154,0.));
#15645=CARTESIAN_POINT('Ctrl Pts',(-6.11877533761502,21.1133530893457,0.));
#15646=CARTESIAN_POINT('Ctrl Pts',(-6.1342227326009,21.1275013067528,0.));
#15647=CARTESIAN_POINT('Ctrl Pts',(-4.1144891981253,18.337935196262,13.));
#15648=CARTESIAN_POINT('Ctrl Pts',(-4.11796712887951,18.3534360435645,13.));
#15649=CARTESIAN_POINT('Ctrl Pts',(-4.12185943358937,18.3688191548995,13.));
#15650=CARTESIAN_POINT('Ctrl Pts',(-4.12613856044267,18.3840926404824,13.));
#15651=CARTESIAN_POINT('Ctrl Pts',(-4.13115401716693,18.4019943079477,13.));
#15652=CARTESIAN_POINT('Ctrl Pts',(-4.13670006307401,18.4197456248295,13.));
#15653=CARTESIAN_POINT('Ctrl Pts',(-4.1426637807957,18.4373797424196,13.));
#15654=CARTESIAN_POINT('Ctrl Pts',(-4.15105501703309,18.4621917897769,13.));
#15655=CARTESIAN_POINT('Ctrl Pts',(-4.16026629328986,18.4867739015683,13.));
#15656=CARTESIAN_POINT('Ctrl Pts',(-4.16990400115281,18.5112408492934,13.));
#15657=CARTESIAN_POINT('Ctrl Pts',(-4.17631459686345,18.5275152282609,13.));
#15658=CARTESIAN_POINT('Ctrl Pts',(-4.18291190640786,18.5437392096496,13.));
#15659=CARTESIAN_POINT('Ctrl Pts',(-4.18960898617042,18.5599376581358,13.));
#15660=CARTESIAN_POINT('Ctrl Pts',(-4.19665876042785,18.5769891804703,13.));
#15661=CARTESIAN_POINT('Ctrl Pts',(-4.20381824254442,18.5940126577989,13.));
#15662=CARTESIAN_POINT('Ctrl Pts',(-4.21104759333806,18.6110185062838,13.));
#15663=CARTESIAN_POINT('Ctrl Pts',(-4.21907618313382,18.6299044319376,13.));
#15664=CARTESIAN_POINT('Ctrl Pts',(-4.22719219297435,18.6487682283615,13.));
#15665=CARTESIAN_POINT('Ctrl Pts',(-4.23540730606871,18.6676042988365,13.));
#15666=CARTESIAN_POINT('Ctrl Pts',(-4.24779198778706,18.6960005893047,13.));
#15667=CARTESIAN_POINT('Ctrl Pts',(-4.26040793123126,18.7243319351566,13.));
#15668=CARTESIAN_POINT('Ctrl Pts',(-4.27340283281641,18.7525479285623,13.));
#15669=CARTESIAN_POINT('Ctrl Pts',(-4.28284334471974,18.7730462309053,13.));
#15670=CARTESIAN_POINT('Ctrl Pts',(-4.29248702330122,18.7934827312586,13.));
#15671=CARTESIAN_POINT('Ctrl Pts',(-4.30235320731447,18.8138501272238,13.));
#15672=CARTESIAN_POINT('Ctrl Pts',(-4.31441377244466,18.8387475247628,13.));
#15673=CARTESIAN_POINT('Ctrl Pts',(-4.32680560862846,18.8635420328974,13.));
#15674=CARTESIAN_POINT('Ctrl Pts',(-4.33948253068855,18.888246010372,13.));
#15675=CARTESIAN_POINT('Ctrl Pts',(-4.35317571045463,18.9149304060711,13.));
#15676=CARTESIAN_POINT('Ctrl Pts',(-4.36719580768566,18.9415109549159,13.));
#15677=CARTESIAN_POINT('Ctrl Pts',(-4.3814546652845,18.9680129070776,13.));
#15678=CARTESIAN_POINT('Ctrl Pts',(-4.39461837563789,18.9924793848188,13.));
#15679=CARTESIAN_POINT('Ctrl Pts',(-4.40798318218919,19.0168796293449,13.));
#15680=CARTESIAN_POINT('Ctrl Pts',(-4.42152146523478,19.0412206988196,13.));
#15681=CARTESIAN_POINT('Ctrl Pts',(-4.43991391787386,19.0742892914905,13.));
#15682=CARTESIAN_POINT('Ctrl Pts',(-4.45862842578007,19.1072480695063,13.));
#15683=CARTESIAN_POINT('Ctrl Pts',(-4.47769255661886,19.1400849916113,13.));
#15684=CARTESIAN_POINT('Ctrl Pts',(-4.49608903112579,19.1717719122214,13.));
#15685=CARTESIAN_POINT('Ctrl Pts',(-4.51481852740326,19.2033430482922,13.));
#15686=CARTESIAN_POINT('Ctrl Pts',(-4.53389559678128,19.2347910922226,13.));
#15687=CARTESIAN_POINT('Ctrl Pts',(-4.55981233004855,19.2775141410396,13.));
#15688=CARTESIAN_POINT('Ctrl Pts',(-4.58636743963562,19.3200109590135,13.));
#15689=CARTESIAN_POINT('Ctrl Pts',(-4.61347737159604,19.3623013141123,13.));
#15690=CARTESIAN_POINT('Ctrl Pts',(-4.63730641242961,19.3994736168679,13.));
#15691=CARTESIAN_POINT('Ctrl Pts',(-4.66155758363823,19.4364884570226,13.));
#15692=CARTESIAN_POINT('Ctrl Pts',(-4.68619912923096,19.4733518502478,13.));
#15693=CARTESIAN_POINT('Ctrl Pts',(-4.72252674998903,19.527697441676,13.));
#15694=CARTESIAN_POINT('Ctrl Pts',(-4.75971143888908,19.5817111524814,13.));
#15695=CARTESIAN_POINT('Ctrl Pts',(-4.79774570283441,19.6353839062314,13.));
#15696=CARTESIAN_POINT('Ctrl Pts',(-4.84574531506025,19.7031194451863,13.));
#15697=CARTESIAN_POINT('Ctrl Pts',(-4.895093042552,19.7703134645498,13.));
#15698=CARTESIAN_POINT('Ctrl Pts',(-4.94566457605319,19.836983801638,13.));
#15699=CARTESIAN_POINT('Ctrl Pts',(-5.01416761715498,19.9272939133872,13.));
#15700=CARTESIAN_POINT('Ctrl Pts',(-5.08492180300406,20.01664136013,13.));
#15701=CARTESIAN_POINT('Ctrl Pts',(-5.15778644827778,20.105022570296,13.));
#15702=CARTESIAN_POINT('Ctrl Pts',(-5.22274718768723,20.1838167336481,13.));
#15703=CARTESIAN_POINT('Ctrl Pts',(-5.28937724215395,20.2618454265211,13.));
#15704=CARTESIAN_POINT('Ctrl Pts',(-5.35757729622096,20.3391090329722,13.));
#15705=CARTESIAN_POINT('Ctrl Pts',(-5.454235527518,20.4486128104304,13.));
#15706=CARTESIAN_POINT('Ctrl Pts',(-5.55405241051352,20.5565772409248,13.));
#15707=CARTESIAN_POINT('Ctrl Pts',(-5.65680258430444,20.6629906948204,13.));
#15708=CARTESIAN_POINT('Ctrl Pts',(-5.73661648166364,20.7456501412575,13.));
#15709=CARTESIAN_POINT('Ctrl Pts',(-5.81820510861819,20.8273750324251,13.));
#15710=CARTESIAN_POINT('Ctrl Pts',(-5.90147459212854,20.908152214715,13.));
#15711=CARTESIAN_POINT('Ctrl Pts',(-5.97350898952772,20.9780305831708,13.));
#15712=CARTESIAN_POINT('Ctrl Pts',(-6.04679718411003,21.0471984364812,13.));
#15713=CARTESIAN_POINT('Ctrl Pts',(-6.12131239112586,21.1156584400056,13.));
#15714=CARTESIAN_POINT('Ctrl Pts',(-6.12561173959338,21.1196084177756,13.));
#15715=CARTESIAN_POINT('Ctrl Pts',(-6.12991518682867,21.1235560399827,13.));
#15716=CARTESIAN_POINT('Ctrl Pts',(-6.1342227326009,21.1275013067528,13.));
#15717=CARTESIAN_POINT('Ctrl Pts',(-0.69476445021958,21.9890268624765,0.));
#15718=CARTESIAN_POINT('Ctrl Pts',(-0.69476445021958,21.9890268624765,21.));
#15719=CARTESIAN_POINT('Ctrl Pts',(-0.699924103234222,21.9799122315157,
0.));
#15720=CARTESIAN_POINT('Ctrl Pts',(-0.699924103234222,21.9799122315157,
21.));
#15721=CARTESIAN_POINT('Ctrl Pts',(-0.710218621843556,21.9616777523685,
0.));
#15722=CARTESIAN_POINT('Ctrl Pts',(-0.710218621843556,21.9616777523685,
21.));
#15723=CARTESIAN_POINT('Ctrl Pts',(-0.725586037496635,21.9343103819749,
0.));
#15724=CARTESIAN_POINT('Ctrl Pts',(-0.725586037496635,21.9343103819749,
21.));
#15725=CARTESIAN_POINT('Ctrl Pts',(-0.745927151109821,21.8977892409997,
0.));
#15726=CARTESIAN_POINT('Ctrl Pts',(-0.745927151109821,21.8977892409997,
21.));
#15727=CARTESIAN_POINT('Ctrl Pts',(-0.77110521325833,21.8520856039249,0.));
#15728=CARTESIAN_POINT('Ctrl Pts',(-0.77110521325833,21.8520856039249,21.));
#15729=CARTESIAN_POINT('Ctrl Pts',(-0.796034321106412,21.8063297959755,
0.));
#15730=CARTESIAN_POINT('Ctrl Pts',(-0.796034321106412,21.8063297959755,
21.));
#15731=CARTESIAN_POINT('Ctrl Pts',(-0.820713597934077,21.7605219769118,
0.));
#15732=CARTESIAN_POINT('Ctrl Pts',(-0.820713597934077,21.7605219769118,
21.));
#15733=CARTESIAN_POINT('Ctrl Pts',(-0.845141916726557,21.7146624809285,
0.));
#15734=CARTESIAN_POINT('Ctrl Pts',(-0.845141916726557,21.7146624809285,
21.));
#15735=CARTESIAN_POINT('Ctrl Pts',(-0.869317897714099,21.6687518829182,
0.));
#15736=CARTESIAN_POINT('Ctrl Pts',(-0.869317897714099,21.6687518829182,
21.));
#15737=CARTESIAN_POINT('Ctrl Pts',(-0.893239967513673,21.6227909401433,
0.));
#15738=CARTESIAN_POINT('Ctrl Pts',(-0.893239967513673,21.6227909401433,
21.));
#15739=CARTESIAN_POINT('Ctrl Pts',(-0.916906425150853,21.5767805209408,
0.));
#15740=CARTESIAN_POINT('Ctrl Pts',(-0.916906425150853,21.5767805209408,
21.));
#15741=CARTESIAN_POINT('Ctrl Pts',(-0.940315509525149,21.5307215366685,
0.));
#15742=CARTESIAN_POINT('Ctrl Pts',(-0.940315509525149,21.5307215366685,
21.));
#15743=CARTESIAN_POINT('Ctrl Pts',(-0.963465462815771,21.4846148770804,
0.));
#15744=CARTESIAN_POINT('Ctrl Pts',(-0.963465462815771,21.4846148770804,
21.));
#15745=CARTESIAN_POINT('Ctrl Pts',(-0.986354611081133,21.4384613333266,
0.));
#15746=CARTESIAN_POINT('Ctrl Pts',(-0.986354611081133,21.4384613333266,
21.));
#15747=CARTESIAN_POINT('Ctrl Pts',(-1.00898133629988,21.3922616124166,0.));
#15748=CARTESIAN_POINT('Ctrl Pts',(-1.00898133629988,21.3922616124166,21.));
#15749=CARTESIAN_POINT('Ctrl Pts',(-1.03134402396953,21.3460163737343,0.));
#15750=CARTESIAN_POINT('Ctrl Pts',(-1.03134402396953,21.3460163737343,21.));
#15751=CARTESIAN_POINT('Ctrl Pts',(-1.05344101900192,21.2997262593683,0.));
#15752=CARTESIAN_POINT('Ctrl Pts',(-1.05344101900192,21.2997262593683,21.));
#15753=CARTESIAN_POINT('Ctrl Pts',(-1.07527058431887,21.2533919248553,0.));
#15754=CARTESIAN_POINT('Ctrl Pts',(-1.07527058431887,21.2533919248553,21.));
#15755=CARTESIAN_POINT('Ctrl Pts',(-1.09683084929266,21.2070140764156,0.));
#15756=CARTESIAN_POINT('Ctrl Pts',(-1.09683084929266,21.2070140764156,21.));
#15757=CARTESIAN_POINT('Ctrl Pts',(-1.11811982787746,21.1605934684164,0.));
#15758=CARTESIAN_POINT('Ctrl Pts',(-1.11811982787746,21.1605934684164,21.));
#15759=CARTESIAN_POINT('Ctrl Pts',(-1.13913546246555,21.1141308858087,0.));
#15760=CARTESIAN_POINT('Ctrl Pts',(-1.13913546246555,21.1141308858087,21.));
#15761=CARTESIAN_POINT('Ctrl Pts',(-1.15987566445807,21.0676271313238,0.));
#15762=CARTESIAN_POINT('Ctrl Pts',(-1.15987566445807,21.0676271313238,21.));
#15763=CARTESIAN_POINT('Ctrl Pts',(-1.18033835060894,21.0210830121673,0.));
#15764=CARTESIAN_POINT('Ctrl Pts',(-1.18033835060894,21.0210830121673,21.));
#15765=CARTESIAN_POINT('Ctrl Pts',(-1.20052150219503,20.9744993243732,0.));
#15766=CARTESIAN_POINT('Ctrl Pts',(-1.20052150219503,20.9744993243732,21.));
#15767=CARTESIAN_POINT('Ctrl Pts',(-1.22042312071096,20.9278768531175,0.));
#15768=CARTESIAN_POINT('Ctrl Pts',(-1.22042312071096,20.9278768531175,21.));
#15769=CARTESIAN_POINT('Ctrl Pts',(-1.24004113517905,20.881216381382,0.));
#15770=CARTESIAN_POINT('Ctrl Pts',(-1.24004113517905,20.881216381382,21.));
#15771=CARTESIAN_POINT('Ctrl Pts',(-1.25937332001005,20.83451869657,0.));
#15772=CARTESIAN_POINT('Ctrl Pts',(-1.25937332001005,20.83451869657,21.));
#15773=CARTESIAN_POINT('Ctrl Pts',(-1.27841722479262,20.7877845975367,0.));
#15774=CARTESIAN_POINT('Ctrl Pts',(-1.27841722479262,20.7877845975367,21.));
#15775=CARTESIAN_POINT('Ctrl Pts',(-1.29717006491149,20.7410149035348,0.));
#15776=CARTESIAN_POINT('Ctrl Pts',(-1.29717006491149,20.7410149035348,21.));
#15777=CARTESIAN_POINT('Ctrl Pts',(-1.31562879653596,20.694210454218,0.));
#15778=CARTESIAN_POINT('Ctrl Pts',(-1.31562879653596,20.694210454218,21.));
#15779=CARTESIAN_POINT('Ctrl Pts',(-1.3337902972259,20.6473721041685,0.));
#15780=CARTESIAN_POINT('Ctrl Pts',(-1.3337902972259,20.6473721041685,21.));
#15781=CARTESIAN_POINT('Ctrl Pts',(-1.35165153211253,20.6005007190809,0.));
#15782=CARTESIAN_POINT('Ctrl Pts',(-1.35165153211253,20.6005007190809,21.));
#15783=CARTESIAN_POINT('Ctrl Pts',(-1.36920969340018,20.5535971721246,0.));
#15784=CARTESIAN_POINT('Ctrl Pts',(-1.36920969340018,20.5535971721246,21.));
#15785=CARTESIAN_POINT('Ctrl Pts',(-1.38646244026049,20.5066623390132,0.));
#15786=CARTESIAN_POINT('Ctrl Pts',(-1.38646244026049,20.5066623390132,21.));
#15787=CARTESIAN_POINT('Ctrl Pts',(-1.40340771617024,20.4596971004275,0.));
#15788=CARTESIAN_POINT('Ctrl Pts',(-1.40340771617024,20.4596971004275,21.));
#15789=CARTESIAN_POINT('Ctrl Pts',(-1.4200432946371,20.4127023494155,0.));
#15790=CARTESIAN_POINT('Ctrl Pts',(-1.4200432946371,20.4127023494155,21.));
#15791=CARTESIAN_POINT('Ctrl Pts',(-1.43636637152782,20.3656789980171,0.));
#15792=CARTESIAN_POINT('Ctrl Pts',(-1.43636637152782,20.3656789980171,21.));
#15793=CARTESIAN_POINT('Ctrl Pts',(-1.45237321894403,20.3186279833818,0.));
#15794=CARTESIAN_POINT('Ctrl Pts',(-1.45237321894403,20.3186279833818,21.));
#15795=CARTESIAN_POINT('Ctrl Pts',(-1.46805861808021,20.2715502770004,0.));
#15796=CARTESIAN_POINT('Ctrl Pts',(-1.46805861808021,20.2715502770004,21.));
#15797=CARTESIAN_POINT('Ctrl Pts',(-1.48341623961913,20.224446881308,0.));
#15798=CARTESIAN_POINT('Ctrl Pts',(-1.48341623961913,20.224446881308,21.));
#15799=CARTESIAN_POINT('Ctrl Pts',(-1.49843965844502,20.1773188177942,0.));
#15800=CARTESIAN_POINT('Ctrl Pts',(-1.49843965844502,20.1773188177942,21.));
#15801=CARTESIAN_POINT('Ctrl Pts',(-1.51312326913583,20.1301671167606,0.));
#15802=CARTESIAN_POINT('Ctrl Pts',(-1.51312326913583,20.1301671167606,21.));
#15803=CARTESIAN_POINT('Ctrl Pts',(-1.52746305716964,20.0829928089241,0.));
#15804=CARTESIAN_POINT('Ctrl Pts',(-1.52746305716964,20.0829928089241,21.));
#15805=CARTESIAN_POINT('Ctrl Pts',(-1.54145790302917,20.0357969106526,0.));
#15806=CARTESIAN_POINT('Ctrl Pts',(-1.54145790302917,20.0357969106526,21.));
#15807=CARTESIAN_POINT('Ctrl Pts',(-1.55510860515913,19.9885804375097,0.));
#15808=CARTESIAN_POINT('Ctrl Pts',(-1.55510860515913,19.9885804375097,21.));
#15809=CARTESIAN_POINT('Ctrl Pts',(-1.56841542790452,19.9413444362352,0.));
#15810=CARTESIAN_POINT('Ctrl Pts',(-1.56841542790452,19.9413444362352,21.));
#15811=CARTESIAN_POINT('Ctrl Pts',(-1.58137589158952,19.8940900137801,0.));
#15812=CARTESIAN_POINT('Ctrl Pts',(-1.58137589158952,19.8940900137801,21.));
#15813=CARTESIAN_POINT('Ctrl Pts',(-1.59398289700559,19.8468183626037,0.));
#15814=CARTESIAN_POINT('Ctrl Pts',(-1.59398289700559,19.8468183626037,21.));
#15815=CARTESIAN_POINT('Ctrl Pts',(-1.60622162219699,19.7995308006834,0.));
#15816=CARTESIAN_POINT('Ctrl Pts',(-1.60622162219699,19.7995308006834,21.));
#15817=CARTESIAN_POINT('Ctrl Pts',(-1.61807191996834,19.7522287462982,0.));
#15818=CARTESIAN_POINT('Ctrl Pts',(-1.61807191996834,19.7522287462982,21.));
#15819=CARTESIAN_POINT('Ctrl Pts',(-1.62951389038421,19.7049136553525,0.));
#15820=CARTESIAN_POINT('Ctrl Pts',(-1.62951389038421,19.7049136553525,21.));
#15821=CARTESIAN_POINT('Ctrl Pts',(-1.64053294677821,19.6575869645839,0.));
#15822=CARTESIAN_POINT('Ctrl Pts',(-1.64053294677821,19.6575869645839,21.));
#15823=CARTESIAN_POINT('Ctrl Pts',(-1.65112409599283,19.6102500448855,0.));
#15824=CARTESIAN_POINT('Ctrl Pts',(-1.65112409599283,19.6102500448855,21.));
#15825=CARTESIAN_POINT('Ctrl Pts',(-1.66129908621006,19.5629041190868,0.));
#15826=CARTESIAN_POINT('Ctrl Pts',(-1.66129908621006,19.5629041190868,21.));
#15827=CARTESIAN_POINT('Ctrl Pts',(-1.67107974760949,19.5155503513712,0.));
#15828=CARTESIAN_POINT('Ctrl Pts',(-1.67107974760949,19.5155503513712,21.));
#15829=CARTESIAN_POINT('Ctrl Pts',(-1.68048476382294,19.4681900187091,0.));
#15830=CARTESIAN_POINT('Ctrl Pts',(-1.68048476382294,19.4681900187091,21.));
#15831=CARTESIAN_POINT('Ctrl Pts',(-1.68951753233571,19.4208246682917,0.));
#15832=CARTESIAN_POINT('Ctrl Pts',(-1.68951753233571,19.4208246682917,21.));
#15833=CARTESIAN_POINT('Ctrl Pts',(-1.69815571801252,19.3734562555057,0.));
#15834=CARTESIAN_POINT('Ctrl Pts',(-1.69815571801252,19.3734562555057,21.));
#15835=CARTESIAN_POINT('Ctrl Pts',(-1.70633457265124,19.3260873558094,0.));
#15836=CARTESIAN_POINT('Ctrl Pts',(-1.70633457265124,19.3260873558094,21.));
#15837=CARTESIAN_POINT('Ctrl Pts',(-1.71396454346262,19.2787209722437,0.));
#15838=CARTESIAN_POINT('Ctrl Pts',(-1.71396454346262,19.2787209722437,21.));
#15839=CARTESIAN_POINT('Ctrl Pts',(-1.72096104670234,19.2313602042899,0.));
#15840=CARTESIAN_POINT('Ctrl Pts',(-1.72096104670234,19.2313602042899,21.));
#15841=CARTESIAN_POINT('Ctrl Pts',(-1.72727220327098,19.1840079312107,0.));
#15842=CARTESIAN_POINT('Ctrl Pts',(-1.72727220327098,19.1840079312107,21.));
#15843=CARTESIAN_POINT('Ctrl Pts',(-1.73290313712353,19.1366665585833,0.));
#15844=CARTESIAN_POINT('Ctrl Pts',(-1.73290313712353,19.1366665585833,21.));
#15845=CARTESIAN_POINT('Ctrl Pts',(-1.7379530116984,19.0893375576541,0.));
#15846=CARTESIAN_POINT('Ctrl Pts',(-1.7379530116984,19.0893375576541,21.));
#15847=CARTESIAN_POINT('Ctrl Pts',(-1.74256297552949,19.0420224296189,0.));
#15848=CARTESIAN_POINT('Ctrl Pts',(-1.74256297552949,19.0420224296189,21.));
#15849=CARTESIAN_POINT('Ctrl Pts',(-1.74684309825012,18.9947239970259,0.));
#15850=CARTESIAN_POINT('Ctrl Pts',(-1.74684309825012,18.9947239970259,21.));
#15851=CARTESIAN_POINT('Ctrl Pts',(-1.75080409924533,18.947447637865,0.));
#15852=CARTESIAN_POINT('Ctrl Pts',(-1.75080409924533,18.947447637865,21.));
#15853=CARTESIAN_POINT('Ctrl Pts',(-1.75429229572775,18.9002024267872,0.));
#15854=CARTESIAN_POINT('Ctrl Pts',(-1.75429229572775,18.9002024267872,21.));
#15855=CARTESIAN_POINT('Ctrl Pts',(-1.75690876962597,18.8530026395886,0.));
#15856=CARTESIAN_POINT('Ctrl Pts',(-1.75690876962597,18.8530026395886,21.));
#15857=CARTESIAN_POINT('Ctrl Pts',(-1.7581175236483,18.8058650094753,0.));
#15858=CARTESIAN_POINT('Ctrl Pts',(-1.7581175236483,18.8058650094753,21.));
#15859=CARTESIAN_POINT('Ctrl Pts',(-1.75752447968136,18.7682173836138,0.));
#15860=CARTESIAN_POINT('Ctrl Pts',(-1.75752447968136,18.7682173836138,21.));
#15861=CARTESIAN_POINT('Ctrl Pts',(-1.75601041697575,18.7400222442427,0.));
#15862=CARTESIAN_POINT('Ctrl Pts',(-1.75601041697575,18.7400222442427,21.));
#15863=CARTESIAN_POINT('Ctrl Pts',(-1.75450132833464,18.7212441956871,0.));
#15864=CARTESIAN_POINT('Ctrl Pts',(-1.75450132833464,18.7212441956871,21.));
#15865=CARTESIAN_POINT('Ctrl Pts',(-1.75362185428836,18.7118598491961,0.));
#15866=CARTESIAN_POINT('Ctrl Pts',(-1.75362185428836,18.7118598491961,21.));
#15867=CARTESIAN_POINT('',(-0.694764450219644,21.9890268624765,0.));
#15868=CARTESIAN_POINT('Ctrl Pts',(-1.75362185428836,18.7118598491961,0.));
#15869=CARTESIAN_POINT('Ctrl Pts',(-1.75450132833464,18.7212441956871,0.));
#15870=CARTESIAN_POINT('Ctrl Pts',(-1.75601041697575,18.7400222442427,0.));
#15871=CARTESIAN_POINT('Ctrl Pts',(-1.75752447968136,18.7682173836138,0.));
#15872=CARTESIAN_POINT('Ctrl Pts',(-1.7581175236483,18.8058650094753,0.));
#15873=CARTESIAN_POINT('Ctrl Pts',(-1.75690876962597,18.8530026395886,0.));
#15874=CARTESIAN_POINT('Ctrl Pts',(-1.75429229572775,18.9002024267872,0.));
#15875=CARTESIAN_POINT('Ctrl Pts',(-1.75080409924533,18.947447637865,0.));
#15876=CARTESIAN_POINT('Ctrl Pts',(-1.74684309825012,18.9947239970259,0.));
#15877=CARTESIAN_POINT('Ctrl Pts',(-1.74256297552949,19.0420224296189,0.));
#15878=CARTESIAN_POINT('Ctrl Pts',(-1.7379530116984,19.0893375576541,0.));
#15879=CARTESIAN_POINT('Ctrl Pts',(-1.73290313712353,19.1366665585833,0.));
#15880=CARTESIAN_POINT('Ctrl Pts',(-1.72727220327098,19.1840079312107,0.));
#15881=CARTESIAN_POINT('Ctrl Pts',(-1.72096104670234,19.2313602042899,0.));
#15882=CARTESIAN_POINT('Ctrl Pts',(-1.71396454346262,19.2787209722437,0.));
#15883=CARTESIAN_POINT('Ctrl Pts',(-1.70633457265124,19.3260873558094,0.));
#15884=CARTESIAN_POINT('Ctrl Pts',(-1.69815571801252,19.3734562555057,0.));
#15885=CARTESIAN_POINT('Ctrl Pts',(-1.68951753233571,19.4208246682917,0.));
#15886=CARTESIAN_POINT('Ctrl Pts',(-1.68048476382294,19.4681900187091,0.));
#15887=CARTESIAN_POINT('Ctrl Pts',(-1.67107974760949,19.5155503513712,0.));
#15888=CARTESIAN_POINT('Ctrl Pts',(-1.66129908621006,19.5629041190868,0.));
#15889=CARTESIAN_POINT('Ctrl Pts',(-1.65112409599283,19.6102500448855,0.));
#15890=CARTESIAN_POINT('Ctrl Pts',(-1.64053294677821,19.6575869645839,0.));
#15891=CARTESIAN_POINT('Ctrl Pts',(-1.62951389038421,19.7049136553525,0.));
#15892=CARTESIAN_POINT('Ctrl Pts',(-1.61807191996834,19.7522287462982,0.));
#15893=CARTESIAN_POINT('Ctrl Pts',(-1.60622162219699,19.7995308006834,0.));
#15894=CARTESIAN_POINT('Ctrl Pts',(-1.59398289700559,19.8468183626037,0.));
#15895=CARTESIAN_POINT('Ctrl Pts',(-1.58137589158952,19.8940900137801,0.));
#15896=CARTESIAN_POINT('Ctrl Pts',(-1.56841542790452,19.9413444362352,0.));
#15897=CARTESIAN_POINT('Ctrl Pts',(-1.55510860515913,19.9885804375097,0.));
#15898=CARTESIAN_POINT('Ctrl Pts',(-1.54145790302917,20.0357969106526,0.));
#15899=CARTESIAN_POINT('Ctrl Pts',(-1.52746305716964,20.0829928089241,0.));
#15900=CARTESIAN_POINT('Ctrl Pts',(-1.51312326913583,20.1301671167606,0.));
#15901=CARTESIAN_POINT('Ctrl Pts',(-1.49843965844502,20.1773188177942,0.));
#15902=CARTESIAN_POINT('Ctrl Pts',(-1.48341623961913,20.224446881308,0.));
#15903=CARTESIAN_POINT('Ctrl Pts',(-1.46805861808021,20.2715502770004,0.));
#15904=CARTESIAN_POINT('Ctrl Pts',(-1.45237321894403,20.3186279833818,0.));
#15905=CARTESIAN_POINT('Ctrl Pts',(-1.43636637152782,20.3656789980171,0.));
#15906=CARTESIAN_POINT('Ctrl Pts',(-1.4200432946371,20.4127023494155,0.));
#15907=CARTESIAN_POINT('Ctrl Pts',(-1.40340771617024,20.4596971004275,0.));
#15908=CARTESIAN_POINT('Ctrl Pts',(-1.38646244026049,20.5066623390132,0.));
#15909=CARTESIAN_POINT('Ctrl Pts',(-1.36920969340018,20.5535971721246,0.));
#15910=CARTESIAN_POINT('Ctrl Pts',(-1.35165153211253,20.6005007190809,0.));
#15911=CARTESIAN_POINT('Ctrl Pts',(-1.3337902972259,20.6473721041685,0.));
#15912=CARTESIAN_POINT('Ctrl Pts',(-1.31562879653596,20.694210454218,0.));
#15913=CARTESIAN_POINT('Ctrl Pts',(-1.29717006491149,20.7410149035348,0.));
#15914=CARTESIAN_POINT('Ctrl Pts',(-1.27841722479262,20.7877845975367,0.));
#15915=CARTESIAN_POINT('Ctrl Pts',(-1.25937332001005,20.83451869657,0.));
#15916=CARTESIAN_POINT('Ctrl Pts',(-1.24004113517905,20.881216381382,0.));
#15917=CARTESIAN_POINT('Ctrl Pts',(-1.22042312071096,20.9278768531175,0.));
#15918=CARTESIAN_POINT('Ctrl Pts',(-1.20052150219503,20.9744993243732,0.));
#15919=CARTESIAN_POINT('Ctrl Pts',(-1.18033835060894,21.0210830121673,0.));
#15920=CARTESIAN_POINT('Ctrl Pts',(-1.15987566445807,21.0676271313238,0.));
#15921=CARTESIAN_POINT('Ctrl Pts',(-1.13913546246555,21.1141308858087,0.));
#15922=CARTESIAN_POINT('Ctrl Pts',(-1.11811982787746,21.1605934684164,0.));
#15923=CARTESIAN_POINT('Ctrl Pts',(-1.09683084929266,21.2070140764156,0.));
#15924=CARTESIAN_POINT('Ctrl Pts',(-1.07527058431887,21.2533919248553,0.));
#15925=CARTESIAN_POINT('Ctrl Pts',(-1.05344101900192,21.2997262593683,0.));
#15926=CARTESIAN_POINT('Ctrl Pts',(-1.03134402396953,21.3460163737343,0.));
#15927=CARTESIAN_POINT('Ctrl Pts',(-1.00898133629988,21.3922616124166,0.));
#15928=CARTESIAN_POINT('Ctrl Pts',(-0.986354611081133,21.4384613333266,
0.));
#15929=CARTESIAN_POINT('Ctrl Pts',(-0.963465462815771,21.4846148770804,
0.));
#15930=CARTESIAN_POINT('Ctrl Pts',(-0.940315509525149,21.5307215366685,
0.));
#15931=CARTESIAN_POINT('Ctrl Pts',(-0.916906425150853,21.5767805209408,
0.));
#15932=CARTESIAN_POINT('Ctrl Pts',(-0.893239967513673,21.6227909401433,
0.));
#15933=CARTESIAN_POINT('Ctrl Pts',(-0.869317897714099,21.6687518829182,
0.));
#15934=CARTESIAN_POINT('Ctrl Pts',(-0.845141916726557,21.7146624809285,
0.));
#15935=CARTESIAN_POINT('Ctrl Pts',(-0.820713597934077,21.7605219769118,
0.));
#15936=CARTESIAN_POINT('Ctrl Pts',(-0.796034321106412,21.8063297959755,
0.));
#15937=CARTESIAN_POINT('Ctrl Pts',(-0.766119391688713,21.8612367655148,
0.));
#15938=CARTESIAN_POINT('Ctrl Pts',(-0.740879090965097,21.9069273598709,
0.));
#15939=CARTESIAN_POINT('Ctrl Pts',(-0.720488353007147,21.9434380560096,
0.));
#15940=CARTESIAN_POINT('Ctrl Pts',(-0.70508375626176,21.970797600548,0.));
#15941=CARTESIAN_POINT('Ctrl Pts',(-0.69476445021958,21.9890268624765,0.));
#15942=CARTESIAN_POINT('',(-0.694764450219644,21.9890268624765,13.));
#15943=CARTESIAN_POINT('Ctrl Pts',(-0.69476445021958,21.9890268624765,13.));
#15944=CARTESIAN_POINT('Ctrl Pts',(-0.745561803283239,21.8992923152799,
13.));
#15945=CARTESIAN_POINT('Ctrl Pts',(-0.794921865564174,21.8092529630784,
13.));
#15946=CARTESIAN_POINT('Ctrl Pts',(-0.842819260919079,21.7189137537155,
13.));
#15947=CARTESIAN_POINT('Ctrl Pts',(-0.922187323998701,21.5692177626466,
13.));
#15948=CARTESIAN_POINT('Ctrl Pts',(-0.997528955439908,21.4187072727147,
13.));
#15949=CARTESIAN_POINT('Ctrl Pts',(-1.06858105391185,21.2675022584072,13.));
#15950=CARTESIAN_POINT('Ctrl Pts',(-1.12319586329668,21.1512772177393,13.));
#15951=CARTESIAN_POINT('Ctrl Pts',(-1.17527598661216,21.0346391558834,13.));
#15952=CARTESIAN_POINT('Ctrl Pts',(-1.22467603855632,20.917644242923,13.));
#15953=CARTESIAN_POINT('Ctrl Pts',(-1.27785400417095,20.7917020381349,13.));
#15954=CARTESIAN_POINT('Ctrl Pts',(-1.32793259662342,20.6653453744634,13.));
#15955=CARTESIAN_POINT('Ctrl Pts',(-1.37465955681607,20.5386490834201,13.));
#15956=CARTESIAN_POINT('Ctrl Pts',(-1.40052887118435,20.4685065753523,13.));
#15957=CARTESIAN_POINT('Ctrl Pts',(-1.42537603688911,20.3982600582948,13.));
#15958=CARTESIAN_POINT('Ctrl Pts',(-1.44915458805604,20.3279233189672,13.));
#15959=CARTESIAN_POINT('Ctrl Pts',(-1.47206853306895,20.2601440768247,13.));
#15960=CARTESIAN_POINT('Ctrl Pts',(-1.49398338579287,20.1922811204633,13.));
#15961=CARTESIAN_POINT('Ctrl Pts',(-1.51482335730943,20.1243481779698,13.));
#15962=CARTESIAN_POINT('Ctrl Pts',(-1.53283548365772,20.0656332827775,13.));
#15963=CARTESIAN_POINT('Ctrl Pts',(-1.55004791448615,20.0068660712896,13.));
#15964=CARTESIAN_POINT('Ctrl Pts',(-1.5664583915576,19.9480555831788,13.));
#15965=CARTESIAN_POINT('Ctrl Pts',(-1.57823544845321,19.9058499567655,13.));
#15966=CARTESIAN_POINT('Ctrl Pts',(-1.58960230238178,19.8636220200104,13.));
#15967=CARTESIAN_POINT('Ctrl Pts',(-1.60051957231072,19.8213758740547,13.));
#15968=CARTESIAN_POINT('Ctrl Pts',(-1.61125906811029,19.7798176539142,13.));
#15969=CARTESIAN_POINT('Ctrl Pts',(-1.62155711739663,19.7382418845082,13.));
#15970=CARTESIAN_POINT('Ctrl Pts',(-1.631361434785,19.6966529617546,13.));
#15971=CARTESIAN_POINT('Ctrl Pts',(-1.63986235395436,19.6605929224204,13.));
#15972=CARTESIAN_POINT('Ctrl Pts',(-1.64798961246616,19.6245230263946,13.));
#15973=CARTESIAN_POINT('Ctrl Pts',(-1.6557586144792,19.5884457882424,13.));
#15974=CARTESIAN_POINT('Ctrl Pts',(-1.66279554781242,19.5557680879024,13.));
#15975=CARTESIAN_POINT('Ctrl Pts',(-1.66954412482931,19.5230842952898,13.));
#15976=CARTESIAN_POINT('Ctrl Pts',(-1.67602787922142,19.4903963526387,13.));
#15977=CARTESIAN_POINT('Ctrl Pts',(-1.68148945143256,19.4628617564117,13.));
#15978=CARTESIAN_POINT('Ctrl Pts',(-1.68676485592428,19.435324196667,13.));
#15979=CARTESIAN_POINT('Ctrl Pts',(-1.69183425662716,19.4077853967291,13.));
#15980=CARTESIAN_POINT('Ctrl Pts',(-1.69917023102265,19.3679337568473,13.));
#15981=CARTESIAN_POINT('Ctrl Pts',(-1.70607400305428,19.3280794804219,13.));
#15982=CARTESIAN_POINT('Ctrl Pts',(-1.71232694126836,19.2882303925697,13.));
#15983=CARTESIAN_POINT('Ctrl Pts',(-1.71610520911737,19.2641520277611,13.));
#15984=CARTESIAN_POINT('Ctrl Pts',(-1.71964237037416,19.2400756157958,13.));
#15985=CARTESIAN_POINT('Ctrl Pts',(-1.72291205968776,19.2160028183594,13.));
#15986=CARTESIAN_POINT('Ctrl Pts',(-1.7259276330568,19.193800927016,13.));
#15987=CARTESIAN_POINT('Ctrl Pts',(-1.72871436969152,19.171602126741,13.));
#15988=CARTESIAN_POINT('Ctrl Pts',(-1.73129733453724,19.1494073128219,13.));
#15989=CARTESIAN_POINT('Ctrl Pts',(-1.73485046444234,19.1188760970354,13.));
#15990=CARTESIAN_POINT('Ctrl Pts',(-1.73802530995816,19.0883522198594,13.));
#15991=CARTESIAN_POINT('Ctrl Pts',(-1.7409726387683,19.0578380260009,13.));
#15992=CARTESIAN_POINT('Ctrl Pts',(-1.74284247674286,19.0384792770743,13.));
#15993=CARTESIAN_POINT('Ctrl Pts',(-1.74462241724203,19.0191244315393,13.));
#15994=CARTESIAN_POINT('Ctrl Pts',(-1.74632097576209,18.9997750006553,13.));
#15995=CARTESIAN_POINT('Ctrl Pts',(-1.74784535297286,18.9824097870743,13.));
#15996=CARTESIAN_POINT('Ctrl Pts',(-1.74930491161852,18.9650489252156,13.));
#15997=CARTESIAN_POINT('Ctrl Pts',(-1.75066513119703,18.9476944343612,13.));
#15998=CARTESIAN_POINT('Ctrl Pts',(-1.75209499287824,18.9294514081162,13.));
#15999=CARTESIAN_POINT('Ctrl Pts',(-1.75341524153751,18.9112154258559,13.));
#16000=CARTESIAN_POINT('Ctrl Pts',(-1.7545234786503,18.8929901414275,13.));
#16001=CARTESIAN_POINT('Ctrl Pts',(-1.7563642580427,18.8627179843144,13.));
#16002=CARTESIAN_POINT('Ctrl Pts',(-1.75761169393889,18.8324756678297,13.));
#16003=CARTESIAN_POINT('Ctrl Pts',(-1.75764008468139,18.8022820950122,13.));
#16004=CARTESIAN_POINT('Ctrl Pts',(-1.75765574034722,18.7856322843864,13.));
#16005=CARTESIAN_POINT('Ctrl Pts',(-1.75729933637085,18.7689972916942,13.));
#16006=CARTESIAN_POINT('Ctrl Pts',(-1.75649392367898,18.752379304385,13.));
#16007=CARTESIAN_POINT('Ctrl Pts',(-1.75583876199516,18.7388614288199,13.));
#16008=CARTESIAN_POINT('Ctrl Pts',(-1.75488656240175,18.7253548001799,13.));
#16009=CARTESIAN_POINT('Ctrl Pts',(-1.75362185428836,18.7118598491961,13.));
#16010=CARTESIAN_POINT('',(-0.694764450219644,21.9890268624765,0.));
#16011=CARTESIAN_POINT('Origin',(0.,5.6665783176868E-12,0.));
#16012=CARTESIAN_POINT('',(0.694764450219583,21.9890268624765,0.));
#16013=CARTESIAN_POINT('Origin',(0.,5.6665783176868E-12,0.));
#16014=CARTESIAN_POINT('',(0.694764450219583,21.9890268624765,13.));
#16015=CARTESIAN_POINT('Origin',(0.,5.6665783176868E-12,13.));
#16016=CARTESIAN_POINT('',(0.694764450219583,21.9890268624765,0.));
#16017=CARTESIAN_POINT('Ctrl Pts',(1.75362185428837,18.7118598491961,0.));
#16018=CARTESIAN_POINT('Ctrl Pts',(1.75362185428837,18.7118598491961,21.));
#16019=CARTESIAN_POINT('Ctrl Pts',(1.75450132833464,18.7212441956871,0.));
#16020=CARTESIAN_POINT('Ctrl Pts',(1.75450132833464,18.7212441956871,21.));
#16021=CARTESIAN_POINT('Ctrl Pts',(1.75601041697575,18.7400222442427,0.));
#16022=CARTESIAN_POINT('Ctrl Pts',(1.75601041697575,18.7400222442427,21.));
#16023=CARTESIAN_POINT('Ctrl Pts',(1.75752447968136,18.7682173836138,0.));
#16024=CARTESIAN_POINT('Ctrl Pts',(1.75752447968136,18.7682173836138,21.));
#16025=CARTESIAN_POINT('Ctrl Pts',(1.7581175236483,18.8058650094753,0.));
#16026=CARTESIAN_POINT('Ctrl Pts',(1.7581175236483,18.8058650094753,21.));
#16027=CARTESIAN_POINT('Ctrl Pts',(1.75690876962597,18.8530026395886,0.));
#16028=CARTESIAN_POINT('Ctrl Pts',(1.75690876962597,18.8530026395886,21.));
#16029=CARTESIAN_POINT('Ctrl Pts',(1.75429229572775,18.9002024267872,0.));
#16030=CARTESIAN_POINT('Ctrl Pts',(1.75429229572775,18.9002024267872,21.));
#16031=CARTESIAN_POINT('Ctrl Pts',(1.75080409924533,18.947447637865,0.));
#16032=CARTESIAN_POINT('Ctrl Pts',(1.75080409924533,18.947447637865,21.));
#16033=CARTESIAN_POINT('Ctrl Pts',(1.74684309825012,18.9947239970259,0.));
#16034=CARTESIAN_POINT('Ctrl Pts',(1.74684309825012,18.9947239970259,21.));
#16035=CARTESIAN_POINT('Ctrl Pts',(1.74256297552949,19.0420224296189,0.));
#16036=CARTESIAN_POINT('Ctrl Pts',(1.74256297552949,19.0420224296189,21.));
#16037=CARTESIAN_POINT('Ctrl Pts',(1.73795301169841,19.0893375576541,0.));
#16038=CARTESIAN_POINT('Ctrl Pts',(1.73795301169841,19.0893375576541,21.));
#16039=CARTESIAN_POINT('Ctrl Pts',(1.73290313712353,19.1366665585833,0.));
#16040=CARTESIAN_POINT('Ctrl Pts',(1.73290313712353,19.1366665585833,21.));
#16041=CARTESIAN_POINT('Ctrl Pts',(1.72727220327098,19.1840079312107,0.));
#16042=CARTESIAN_POINT('Ctrl Pts',(1.72727220327098,19.1840079312107,21.));
#16043=CARTESIAN_POINT('Ctrl Pts',(1.72096104670234,19.2313602042899,0.));
#16044=CARTESIAN_POINT('Ctrl Pts',(1.72096104670234,19.2313602042899,21.));
#16045=CARTESIAN_POINT('Ctrl Pts',(1.71396454346262,19.2787209722437,0.));
#16046=CARTESIAN_POINT('Ctrl Pts',(1.71396454346262,19.2787209722437,21.));
#16047=CARTESIAN_POINT('Ctrl Pts',(1.70633457265124,19.3260873558094,0.));
#16048=CARTESIAN_POINT('Ctrl Pts',(1.70633457265124,19.3260873558094,21.));
#16049=CARTESIAN_POINT('Ctrl Pts',(1.69815571801252,19.3734562555057,0.));
#16050=CARTESIAN_POINT('Ctrl Pts',(1.69815571801252,19.3734562555057,21.));
#16051=CARTESIAN_POINT('Ctrl Pts',(1.68951753233571,19.4208246682917,0.));
#16052=CARTESIAN_POINT('Ctrl Pts',(1.68951753233571,19.4208246682917,21.));
#16053=CARTESIAN_POINT('Ctrl Pts',(1.68048476382294,19.4681900187091,0.));
#16054=CARTESIAN_POINT('Ctrl Pts',(1.68048476382294,19.4681900187091,21.));
#16055=CARTESIAN_POINT('Ctrl Pts',(1.67107974760949,19.5155503513712,0.));
#16056=CARTESIAN_POINT('Ctrl Pts',(1.67107974760949,19.5155503513712,21.));
#16057=CARTESIAN_POINT('Ctrl Pts',(1.66129908621006,19.5629041190868,0.));
#16058=CARTESIAN_POINT('Ctrl Pts',(1.66129908621006,19.5629041190868,21.));
#16059=CARTESIAN_POINT('Ctrl Pts',(1.65112409599283,19.6102500448855,0.));
#16060=CARTESIAN_POINT('Ctrl Pts',(1.65112409599283,19.6102500448855,21.));
#16061=CARTESIAN_POINT('Ctrl Pts',(1.64053294677821,19.6575869645839,0.));
#16062=CARTESIAN_POINT('Ctrl Pts',(1.64053294677821,19.6575869645839,21.));
#16063=CARTESIAN_POINT('Ctrl Pts',(1.62951389038422,19.7049136553525,0.));
#16064=CARTESIAN_POINT('Ctrl Pts',(1.62951389038422,19.7049136553525,21.));
#16065=CARTESIAN_POINT('Ctrl Pts',(1.61807191996834,19.7522287462982,0.));
#16066=CARTESIAN_POINT('Ctrl Pts',(1.61807191996834,19.7522287462982,21.));
#16067=CARTESIAN_POINT('Ctrl Pts',(1.60622162219699,19.7995308006834,0.));
#16068=CARTESIAN_POINT('Ctrl Pts',(1.60622162219699,19.7995308006834,21.));
#16069=CARTESIAN_POINT('Ctrl Pts',(1.59398289700559,19.8468183626037,0.));
#16070=CARTESIAN_POINT('Ctrl Pts',(1.59398289700559,19.8468183626037,21.));
#16071=CARTESIAN_POINT('Ctrl Pts',(1.58137589158952,19.8940900137801,0.));
#16072=CARTESIAN_POINT('Ctrl Pts',(1.58137589158952,19.8940900137801,21.));
#16073=CARTESIAN_POINT('Ctrl Pts',(1.56841542790452,19.9413444362352,0.));
#16074=CARTESIAN_POINT('Ctrl Pts',(1.56841542790452,19.9413444362352,21.));
#16075=CARTESIAN_POINT('Ctrl Pts',(1.55510860515914,19.9885804375097,0.));
#16076=CARTESIAN_POINT('Ctrl Pts',(1.55510860515914,19.9885804375097,21.));
#16077=CARTESIAN_POINT('Ctrl Pts',(1.54145790302918,20.0357969106526,0.));
#16078=CARTESIAN_POINT('Ctrl Pts',(1.54145790302918,20.0357969106526,21.));
#16079=CARTESIAN_POINT('Ctrl Pts',(1.52746305716964,20.0829928089241,0.));
#16080=CARTESIAN_POINT('Ctrl Pts',(1.52746305716964,20.0829928089241,21.));
#16081=CARTESIAN_POINT('Ctrl Pts',(1.51312326913583,20.1301671167606,0.));
#16082=CARTESIAN_POINT('Ctrl Pts',(1.51312326913583,20.1301671167606,21.));
#16083=CARTESIAN_POINT('Ctrl Pts',(1.49843965844502,20.1773188177942,0.));
#16084=CARTESIAN_POINT('Ctrl Pts',(1.49843965844502,20.1773188177942,21.));
#16085=CARTESIAN_POINT('Ctrl Pts',(1.48341623961914,20.224446881308,0.));
#16086=CARTESIAN_POINT('Ctrl Pts',(1.48341623961914,20.224446881308,21.));
#16087=CARTESIAN_POINT('Ctrl Pts',(1.46805861808021,20.2715502770004,0.));
#16088=CARTESIAN_POINT('Ctrl Pts',(1.46805861808021,20.2715502770004,21.));
#16089=CARTESIAN_POINT('Ctrl Pts',(1.45237321894404,20.3186279833818,0.));
#16090=CARTESIAN_POINT('Ctrl Pts',(1.45237321894404,20.3186279833818,21.));
#16091=CARTESIAN_POINT('Ctrl Pts',(1.43636637152782,20.3656789980171,0.));
#16092=CARTESIAN_POINT('Ctrl Pts',(1.43636637152782,20.3656789980171,21.));
#16093=CARTESIAN_POINT('Ctrl Pts',(1.4200432946371,20.4127023494155,0.));
#16094=CARTESIAN_POINT('Ctrl Pts',(1.4200432946371,20.4127023494155,21.));
#16095=CARTESIAN_POINT('Ctrl Pts',(1.40340771617025,20.4596971004275,0.));
#16096=CARTESIAN_POINT('Ctrl Pts',(1.40340771617025,20.4596971004275,21.));
#16097=CARTESIAN_POINT('Ctrl Pts',(1.38646244026049,20.5066623390132,0.));
#16098=CARTESIAN_POINT('Ctrl Pts',(1.38646244026049,20.5066623390132,21.));
#16099=CARTESIAN_POINT('Ctrl Pts',(1.36920969340018,20.5535971721246,0.));
#16100=CARTESIAN_POINT('Ctrl Pts',(1.36920969340018,20.5535971721246,21.));
#16101=CARTESIAN_POINT('Ctrl Pts',(1.35165153211253,20.6005007190809,0.));
#16102=CARTESIAN_POINT('Ctrl Pts',(1.35165153211253,20.6005007190809,21.));
#16103=CARTESIAN_POINT('Ctrl Pts',(1.3337902972259,20.6473721041685,0.));
#16104=CARTESIAN_POINT('Ctrl Pts',(1.3337902972259,20.6473721041685,21.));
#16105=CARTESIAN_POINT('Ctrl Pts',(1.31562879653596,20.694210454218,0.));
#16106=CARTESIAN_POINT('Ctrl Pts',(1.31562879653596,20.694210454218,21.));
#16107=CARTESIAN_POINT('Ctrl Pts',(1.2971700649115,20.7410149035348,0.));
#16108=CARTESIAN_POINT('Ctrl Pts',(1.2971700649115,20.7410149035348,21.));
#16109=CARTESIAN_POINT('Ctrl Pts',(1.27841722479262,20.7877845975367,0.));
#16110=CARTESIAN_POINT('Ctrl Pts',(1.27841722479262,20.7877845975367,21.));
#16111=CARTESIAN_POINT('Ctrl Pts',(1.25937332001005,20.83451869657,0.));
#16112=CARTESIAN_POINT('Ctrl Pts',(1.25937332001005,20.83451869657,21.));
#16113=CARTESIAN_POINT('Ctrl Pts',(1.24004113517905,20.881216381382,0.));
#16114=CARTESIAN_POINT('Ctrl Pts',(1.24004113517905,20.881216381382,21.));
#16115=CARTESIAN_POINT('Ctrl Pts',(1.22042312071096,20.9278768531175,0.));
#16116=CARTESIAN_POINT('Ctrl Pts',(1.22042312071096,20.9278768531175,21.));
#16117=CARTESIAN_POINT('Ctrl Pts',(1.20052150219503,20.9744993243732,0.));
#16118=CARTESIAN_POINT('Ctrl Pts',(1.20052150219503,20.9744993243732,21.));
#16119=CARTESIAN_POINT('Ctrl Pts',(1.18033835060894,21.0210830121673,0.));
#16120=CARTESIAN_POINT('Ctrl Pts',(1.18033835060894,21.0210830121673,21.));
#16121=CARTESIAN_POINT('Ctrl Pts',(1.15987566445807,21.0676271313238,0.));
#16122=CARTESIAN_POINT('Ctrl Pts',(1.15987566445807,21.0676271313238,21.));
#16123=CARTESIAN_POINT('Ctrl Pts',(1.13913546246555,21.1141308858087,0.));
#16124=CARTESIAN_POINT('Ctrl Pts',(1.13913546246555,21.1141308858087,21.));
#16125=CARTESIAN_POINT('Ctrl Pts',(1.11811982787747,21.1605934684164,0.));
#16126=CARTESIAN_POINT('Ctrl Pts',(1.11811982787747,21.1605934684164,21.));
#16127=CARTESIAN_POINT('Ctrl Pts',(1.09683084929266,21.2070140764156,0.));
#16128=CARTESIAN_POINT('Ctrl Pts',(1.09683084929266,21.2070140764156,21.));
#16129=CARTESIAN_POINT('Ctrl Pts',(1.07527058431887,21.2533919248553,0.));
#16130=CARTESIAN_POINT('Ctrl Pts',(1.07527058431887,21.2533919248553,21.));
#16131=CARTESIAN_POINT('Ctrl Pts',(1.05344101900192,21.2997262593683,0.));
#16132=CARTESIAN_POINT('Ctrl Pts',(1.05344101900192,21.2997262593683,21.));
#16133=CARTESIAN_POINT('Ctrl Pts',(1.03134402396953,21.3460163737343,0.));
#16134=CARTESIAN_POINT('Ctrl Pts',(1.03134402396953,21.3460163737343,21.));
#16135=CARTESIAN_POINT('Ctrl Pts',(1.00898133629988,21.3922616124166,0.));
#16136=CARTESIAN_POINT('Ctrl Pts',(1.00898133629988,21.3922616124166,21.));
#16137=CARTESIAN_POINT('Ctrl Pts',(0.986354611081136,21.4384613333266,0.));
#16138=CARTESIAN_POINT('Ctrl Pts',(0.986354611081136,21.4384613333266,21.));
#16139=CARTESIAN_POINT('Ctrl Pts',(0.963465462815772,21.4846148770804,0.));
#16140=CARTESIAN_POINT('Ctrl Pts',(0.963465462815772,21.4846148770804,21.));
#16141=CARTESIAN_POINT('Ctrl Pts',(0.940315509525153,21.5307215366685,0.));
#16142=CARTESIAN_POINT('Ctrl Pts',(0.940315509525153,21.5307215366685,21.));
#16143=CARTESIAN_POINT('Ctrl Pts',(0.916906425150855,21.5767805209408,0.));
#16144=CARTESIAN_POINT('Ctrl Pts',(0.916906425150855,21.5767805209408,21.));
#16145=CARTESIAN_POINT('Ctrl Pts',(0.893239967513676,21.6227909401433,0.));
#16146=CARTESIAN_POINT('Ctrl Pts',(0.893239967513676,21.6227909401433,21.));
#16147=CARTESIAN_POINT('Ctrl Pts',(0.8693178977141,21.6687518829182,0.));
#16148=CARTESIAN_POINT('Ctrl Pts',(0.8693178977141,21.6687518829182,21.));
#16149=CARTESIAN_POINT('Ctrl Pts',(0.845141916726561,21.7146624809285,0.));
#16150=CARTESIAN_POINT('Ctrl Pts',(0.845141916726561,21.7146624809285,21.));
#16151=CARTESIAN_POINT('Ctrl Pts',(0.820713597934078,21.7605219769118,0.));
#16152=CARTESIAN_POINT('Ctrl Pts',(0.820713597934078,21.7605219769118,21.));
#16153=CARTESIAN_POINT('Ctrl Pts',(0.796034321106414,21.8063297959755,0.));
#16154=CARTESIAN_POINT('Ctrl Pts',(0.796034321106414,21.8063297959755,21.));
#16155=CARTESIAN_POINT('Ctrl Pts',(0.771105213258333,21.8520856039249,0.));
#16156=CARTESIAN_POINT('Ctrl Pts',(0.771105213258333,21.8520856039249,21.));
#16157=CARTESIAN_POINT('Ctrl Pts',(0.745927151109822,21.8977892409997,0.));
#16158=CARTESIAN_POINT('Ctrl Pts',(0.745927151109822,21.8977892409997,21.));
#16159=CARTESIAN_POINT('Ctrl Pts',(0.725586037496637,21.9343103819749,0.));
#16160=CARTESIAN_POINT('Ctrl Pts',(0.725586037496637,21.9343103819749,21.));
#16161=CARTESIAN_POINT('Ctrl Pts',(0.710218621843558,21.9616777523685,0.));
#16162=CARTESIAN_POINT('Ctrl Pts',(0.710218621843558,21.9616777523685,21.));
#16163=CARTESIAN_POINT('Ctrl Pts',(0.699924103234224,21.9799122315157,0.));
#16164=CARTESIAN_POINT('Ctrl Pts',(0.699924103234224,21.9799122315157,21.));
#16165=CARTESIAN_POINT('Ctrl Pts',(0.694764450219582,21.9890268624765,0.));
#16166=CARTESIAN_POINT('Ctrl Pts',(0.694764450219582,21.9890268624765,21.));
#16167=CARTESIAN_POINT('Ctrl Pts',(1.75362185428837,18.7118598491961,0.));
#16168=CARTESIAN_POINT('Ctrl Pts',(1.75450132833464,18.7212441956871,0.));
#16169=CARTESIAN_POINT('Ctrl Pts',(1.75601041697575,18.7400222442427,0.));
#16170=CARTESIAN_POINT('Ctrl Pts',(1.75752447968136,18.7682173836138,0.));
#16171=CARTESIAN_POINT('Ctrl Pts',(1.7581175236483,18.8058650094753,0.));
#16172=CARTESIAN_POINT('Ctrl Pts',(1.75690876962597,18.8530026395886,0.));
#16173=CARTESIAN_POINT('Ctrl Pts',(1.75429229572775,18.9002024267872,0.));
#16174=CARTESIAN_POINT('Ctrl Pts',(1.75080409924533,18.947447637865,0.));
#16175=CARTESIAN_POINT('Ctrl Pts',(1.74684309825012,18.9947239970259,0.));
#16176=CARTESIAN_POINT('Ctrl Pts',(1.74256297552949,19.0420224296189,0.));
#16177=CARTESIAN_POINT('Ctrl Pts',(1.73795301169841,19.0893375576541,0.));
#16178=CARTESIAN_POINT('Ctrl Pts',(1.73290313712353,19.1366665585833,0.));
#16179=CARTESIAN_POINT('Ctrl Pts',(1.72727220327098,19.1840079312107,0.));
#16180=CARTESIAN_POINT('Ctrl Pts',(1.72096104670234,19.2313602042899,0.));
#16181=CARTESIAN_POINT('Ctrl Pts',(1.71396454346262,19.2787209722437,0.));
#16182=CARTESIAN_POINT('Ctrl Pts',(1.70633457265124,19.3260873558094,0.));
#16183=CARTESIAN_POINT('Ctrl Pts',(1.69815571801252,19.3734562555057,0.));
#16184=CARTESIAN_POINT('Ctrl Pts',(1.68951753233571,19.4208246682917,0.));
#16185=CARTESIAN_POINT('Ctrl Pts',(1.68048476382294,19.4681900187091,0.));
#16186=CARTESIAN_POINT('Ctrl Pts',(1.67107974760949,19.5155503513712,0.));
#16187=CARTESIAN_POINT('Ctrl Pts',(1.66129908621006,19.5629041190868,0.));
#16188=CARTESIAN_POINT('Ctrl Pts',(1.65112409599283,19.6102500448855,0.));
#16189=CARTESIAN_POINT('Ctrl Pts',(1.64053294677821,19.6575869645839,0.));
#16190=CARTESIAN_POINT('Ctrl Pts',(1.62951389038422,19.7049136553525,0.));
#16191=CARTESIAN_POINT('Ctrl Pts',(1.61807191996834,19.7522287462982,0.));
#16192=CARTESIAN_POINT('Ctrl Pts',(1.60622162219699,19.7995308006834,0.));
#16193=CARTESIAN_POINT('Ctrl Pts',(1.59398289700559,19.8468183626037,0.));
#16194=CARTESIAN_POINT('Ctrl Pts',(1.58137589158952,19.8940900137801,0.));
#16195=CARTESIAN_POINT('Ctrl Pts',(1.56841542790452,19.9413444362352,0.));
#16196=CARTESIAN_POINT('Ctrl Pts',(1.55510860515914,19.9885804375097,0.));
#16197=CARTESIAN_POINT('Ctrl Pts',(1.54145790302918,20.0357969106526,0.));
#16198=CARTESIAN_POINT('Ctrl Pts',(1.52746305716964,20.0829928089241,0.));
#16199=CARTESIAN_POINT('Ctrl Pts',(1.51312326913583,20.1301671167606,0.));
#16200=CARTESIAN_POINT('Ctrl Pts',(1.49843965844502,20.1773188177942,0.));
#16201=CARTESIAN_POINT('Ctrl Pts',(1.48341623961914,20.224446881308,0.));
#16202=CARTESIAN_POINT('Ctrl Pts',(1.46805861808021,20.2715502770004,0.));
#16203=CARTESIAN_POINT('Ctrl Pts',(1.45237321894404,20.3186279833818,0.));
#16204=CARTESIAN_POINT('Ctrl Pts',(1.43636637152782,20.3656789980171,0.));
#16205=CARTESIAN_POINT('Ctrl Pts',(1.4200432946371,20.4127023494155,0.));
#16206=CARTESIAN_POINT('Ctrl Pts',(1.40340771617025,20.4596971004275,0.));
#16207=CARTESIAN_POINT('Ctrl Pts',(1.38646244026049,20.5066623390132,0.));
#16208=CARTESIAN_POINT('Ctrl Pts',(1.36920969340018,20.5535971721246,0.));
#16209=CARTESIAN_POINT('Ctrl Pts',(1.35165153211253,20.6005007190809,0.));
#16210=CARTESIAN_POINT('Ctrl Pts',(1.3337902972259,20.6473721041685,0.));
#16211=CARTESIAN_POINT('Ctrl Pts',(1.31562879653596,20.694210454218,0.));
#16212=CARTESIAN_POINT('Ctrl Pts',(1.2971700649115,20.7410149035348,0.));
#16213=CARTESIAN_POINT('Ctrl Pts',(1.27841722479262,20.7877845975367,0.));
#16214=CARTESIAN_POINT('Ctrl Pts',(1.25937332001005,20.83451869657,0.));
#16215=CARTESIAN_POINT('Ctrl Pts',(1.24004113517905,20.881216381382,0.));
#16216=CARTESIAN_POINT('Ctrl Pts',(1.22042312071096,20.9278768531175,0.));
#16217=CARTESIAN_POINT('Ctrl Pts',(1.20052150219503,20.9744993243732,0.));
#16218=CARTESIAN_POINT('Ctrl Pts',(1.18033835060894,21.0210830121673,0.));
#16219=CARTESIAN_POINT('Ctrl Pts',(1.15987566445807,21.0676271313238,0.));
#16220=CARTESIAN_POINT('Ctrl Pts',(1.13913546246555,21.1141308858087,0.));
#16221=CARTESIAN_POINT('Ctrl Pts',(1.11811982787747,21.1605934684164,0.));
#16222=CARTESIAN_POINT('Ctrl Pts',(1.09683084929266,21.2070140764156,0.));
#16223=CARTESIAN_POINT('Ctrl Pts',(1.07527058431887,21.2533919248553,0.));
#16224=CARTESIAN_POINT('Ctrl Pts',(1.05344101900192,21.2997262593683,0.));
#16225=CARTESIAN_POINT('Ctrl Pts',(1.03134402396953,21.3460163737343,0.));
#16226=CARTESIAN_POINT('Ctrl Pts',(1.00898133629988,21.3922616124166,0.));
#16227=CARTESIAN_POINT('Ctrl Pts',(0.986354611081136,21.4384613333266,0.));
#16228=CARTESIAN_POINT('Ctrl Pts',(0.963465462815772,21.4846148770804,0.));
#16229=CARTESIAN_POINT('Ctrl Pts',(0.940315509525153,21.5307215366685,0.));
#16230=CARTESIAN_POINT('Ctrl Pts',(0.916906425150855,21.5767805209408,0.));
#16231=CARTESIAN_POINT('Ctrl Pts',(0.893239967513676,21.6227909401433,0.));
#16232=CARTESIAN_POINT('Ctrl Pts',(0.8693178977141,21.6687518829182,0.));
#16233=CARTESIAN_POINT('Ctrl Pts',(0.845141916726561,21.7146624809285,0.));
#16234=CARTESIAN_POINT('Ctrl Pts',(0.820713597934078,21.7605219769118,0.));
#16235=CARTESIAN_POINT('Ctrl Pts',(0.796034321106414,21.8063297959755,0.));
#16236=CARTESIAN_POINT('Ctrl Pts',(0.766119391688716,21.8612367655148,0.));
#16237=CARTESIAN_POINT('Ctrl Pts',(0.740879090965098,21.9069273598709,0.));
#16238=CARTESIAN_POINT('Ctrl Pts',(0.72048835300715,21.9434380560096,0.));
#16239=CARTESIAN_POINT('Ctrl Pts',(0.705083756261762,21.970797600548,0.));
#16240=CARTESIAN_POINT('Ctrl Pts',(0.694764450219582,21.9890268624765,0.));
#16241=CARTESIAN_POINT('Ctrl Pts',(1.75362185428837,18.7118598491961,13.));
#16242=CARTESIAN_POINT('Ctrl Pts',(1.75510417082368,18.7276767707252,13.));
#16243=CARTESIAN_POINT('Ctrl Pts',(1.75615601189427,18.7435097672895,13.));
#16244=CARTESIAN_POINT('Ctrl Pts',(1.75680608702498,18.7593580381841,13.));
#16245=CARTESIAN_POINT('Ctrl Pts',(1.75756802370039,18.7779333970402,13.));
#16246=CARTESIAN_POINT('Ctrl Pts',(1.75777887919059,18.7965297250687,13.));
#16247=CARTESIAN_POINT('Ctrl Pts',(1.75755628860693,18.8151436576359,13.));
#16248=CARTESIAN_POINT('Ctrl Pts',(1.75724309300303,18.8413343515796,13.));
#16249=CARTESIAN_POINT('Ctrl Pts',(1.756078938996,18.8675597701072,13.));
#16250=CARTESIAN_POINT('Ctrl Pts',(1.75447363677689,18.8938074357123,13.));
#16251=CARTESIAN_POINT('Ctrl Pts',(1.7534058576267,18.9112662728963,13.));
#16252=CARTESIAN_POINT('Ctrl Pts',(1.75214492935998,18.9287348768824,13.));
#16253=CARTESIAN_POINT('Ctrl Pts',(1.75078122387634,18.946210028328,13.));
#16254=CARTESIAN_POINT('Ctrl Pts',(1.74934570031147,18.9646054898119,13.));
#16255=CARTESIAN_POINT('Ctrl Pts',(1.74779717198878,18.983008180503,13.));
#16256=CARTESIAN_POINT('Ctrl Pts',(1.74617674699319,19.0014156957761,13.));
#16257=CARTESIAN_POINT('Ctrl Pts',(1.7443771763328,19.0218582491225,13.));
#16258=CARTESIAN_POINT('Ctrl Pts',(1.74248762596105,19.0423067706001,13.));
#16259=CARTESIAN_POINT('Ctrl Pts',(1.74049525500457,19.0627595477229,13.));
#16260=CARTESIAN_POINT('Ctrl Pts',(1.73749165908592,19.0935931019321,13.));
#16261=CARTESIAN_POINT('Ctrl Pts',(1.73424805120572,19.1244363539441,13.));
#16262=CARTESIAN_POINT('Ctrl Pts',(1.73060838684995,19.1552870037662,13.));
#16263=CARTESIAN_POINT('Ctrl Pts',(1.72796425026689,19.177699326396,13.));
#16264=CARTESIAN_POINT('Ctrl Pts',(1.72510779282552,19.2001156537969,13.));
#16265=CARTESIAN_POINT('Ctrl Pts',(1.72201836571307,19.2225350169791,13.));
#16266=CARTESIAN_POINT('Ctrl Pts',(1.7182418056105,19.2499407687372,13.));
#16267=CARTESIAN_POINT('Ctrl Pts',(1.71411839343916,19.2773510352421,13.));
#16268=CARTESIAN_POINT('Ctrl Pts',(1.70969587297501,19.3047632983536,13.));
#16269=CARTESIAN_POINT('Ctrl Pts',(1.7049188168855,19.3343730920189,13.));
#16270=CARTESIAN_POINT('Ctrl Pts',(1.69979875336796,19.3639851445093,13.));
#16271=CARTESIAN_POINT('Ctrl Pts',(1.69442732753607,19.3935962281232,13.));
#16272=CARTESIAN_POINT('Ctrl Pts',(1.68946845243963,19.4209330414214,13.));
#16273=CARTESIAN_POINT('Ctrl Pts',(1.68429785630468,19.4482690053315,13.));
#16274=CARTESIAN_POINT('Ctrl Pts',(1.67894398812285,19.4756022976083,13.));
#16275=CARTESIAN_POINT('Ctrl Pts',(1.6716704833028,19.5127359785976,13.));
#16276=CARTESIAN_POINT('Ctrl Pts',(1.66405675112745,19.5498647401943,13.));
#16277=CARTESIAN_POINT('Ctrl Pts',(1.65607285223626,19.5869856493607,13.));
#16278=CARTESIAN_POINT('Ctrl Pts',(1.64836856224328,19.6228065249654,13.));
#16279=CARTESIAN_POINT('Ctrl Pts',(1.64031177033463,19.658620192316,13.));
#16280=CARTESIAN_POINT('Ctrl Pts',(1.6318863792002,19.6944241980793,13.));
#16281=CARTESIAN_POINT('Ctrl Pts',(1.62044024926504,19.743064943135,13.));
#16282=CARTESIAN_POINT('Ctrl Pts',(1.60831707819419,19.7916877990049,13.));
#16283=CARTESIAN_POINT('Ctrl Pts',(1.59560243915133,19.8402857465542,13.));
#16284=CARTESIAN_POINT('Ctrl Pts',(1.58442654784796,19.8830022859342,13.));
#16285=CARTESIAN_POINT('Ctrl Pts',(1.57280052808028,19.9256995149414,13.));
#16286=CARTESIAN_POINT('Ctrl Pts',(1.56075644053507,19.9683733416781,13.));
#16287=CARTESIAN_POINT('Ctrl Pts',(1.5430005314399,20.0312849226041,13.));
#16288=CARTESIAN_POINT('Ctrl Pts',(1.52432694535417,20.0941457149226,13.));
#16289=CARTESIAN_POINT('Ctrl Pts',(1.50474000386434,20.1569447709389,13.));
#16290=CARTESIAN_POINT('Ctrl Pts',(1.48002109253598,20.2361977925492,13.));
#16291=CARTESIAN_POINT('Ctrl Pts',(1.45385270864268,20.3153523889509,13.));
#16292=CARTESIAN_POINT('Ctrl Pts',(1.42635858934674,20.3943871107668,13.));
#16293=CARTESIAN_POINT('Ctrl Pts',(1.38911568504378,20.5014457348136,13.));
#16294=CARTESIAN_POINT('Ctrl Pts',(1.34943433501682,20.6082844520171,13.));
#16295=CARTESIAN_POINT('Ctrl Pts',(1.30744723528262,20.7148563914567,13.));
#16296=CARTESIAN_POINT('Ctrl Pts',(1.27001463638626,20.8098680661832,13.));
#16297=CARTESIAN_POINT('Ctrl Pts',(1.23075788114852,20.9046675819449,13.));
#16298=CARTESIAN_POINT('Ctrl Pts',(1.18977154286166,20.9992246138384,13.));
#16299=CARTESIAN_POINT('Ctrl Pts',(1.13168263040835,21.1332379308873,13.));
#16300=CARTESIAN_POINT('Ctrl Pts',(1.07011397731129,21.2667633190311,13.));
#16301=CARTESIAN_POINT('Ctrl Pts',(1.00527632077043,21.399720077481,13.));
#16302=CARTESIAN_POINT('Ctrl Pts',(0.954911969009935,21.5029977298323,13.));
#16303=CARTESIAN_POINT('Ctrl Pts',(0.902570955775857,21.6059349889335,13.));
#16304=CARTESIAN_POINT('Ctrl Pts',(0.848338494937178,21.7084903365992,13.));
#16305=CARTESIAN_POINT('Ctrl Pts',(0.801423318189067,21.7972084620133,13.));
#16306=CARTESIAN_POINT('Ctrl Pts',(0.753096148369746,21.8856382920406,13.));
#16307=CARTESIAN_POINT('Ctrl Pts',(0.703383282930066,21.9737740846455,13.));
#16308=CARTESIAN_POINT('Ctrl Pts',(0.700514964692425,21.9788593175944,13.));
#16309=CARTESIAN_POINT('Ctrl Pts',(0.697642020369455,21.9839435768553,13.));
#16310=CARTESIAN_POINT('Ctrl Pts',(0.694764450219583,21.9890268624765,13.));
#16311=CARTESIAN_POINT('Ctrl Pts',(6.13422273260091,21.1275013067528,0.));
#16312=CARTESIAN_POINT('Ctrl Pts',(6.13422273260091,21.1275013067528,21.));
#16313=CARTESIAN_POINT('Ctrl Pts',(6.12649903511518,21.1204271980506,0.));
#16314=CARTESIAN_POINT('Ctrl Pts',(6.12649903511518,21.1204271980506,21.));
#16315=CARTESIAN_POINT('Ctrl Pts',(6.11107360216958,21.1062663590356,0.));
#16316=CARTESIAN_POINT('Ctrl Pts',(6.11107360216958,21.1062663590356,21.));
#16317=CARTESIAN_POINT('Ctrl Pts',(6.08800133883115,21.0849872356853,0.));
#16318=CARTESIAN_POINT('Ctrl Pts',(6.08800133883115,21.0849872356853,21.));
#16319=CARTESIAN_POINT('Ctrl Pts',(6.05737013696533,21.0565393163693,0.));
#16320=CARTESIAN_POINT('Ctrl Pts',(6.05737013696533,21.0565393163693,21.));
#16321=CARTESIAN_POINT('Ctrl Pts',(6.01930117633045,21.0208530236003,0.));
#16322=CARTESIAN_POINT('Ctrl Pts',(6.01930117633045,21.0208530236003,21.));
#16323=CARTESIAN_POINT('Ctrl Pts',(5.98145286361837,20.9850401822713,0.));
#16324=CARTESIAN_POINT('Ctrl Pts',(5.98145286361837,20.9850401822713,21.));
#16325=CARTESIAN_POINT('Ctrl Pts',(5.94382608200804,20.9491006734021,0.));
#16326=CARTESIAN_POINT('Ctrl Pts',(5.94382608200804,20.9491006734021,21.));
#16327=CARTESIAN_POINT('Ctrl Pts',(5.906422006626,20.9130344665641,0.));
#16328=CARTESIAN_POINT('Ctrl Pts',(5.906422006626,20.9130344665641,21.));
#16329=CARTESIAN_POINT('Ctrl Pts',(5.86924212736288,20.8768416821402,0.));
#16330=CARTESIAN_POINT('Ctrl Pts',(5.86924212736288,20.8768416821402,21.));
#16331=CARTESIAN_POINT('Ctrl Pts',(5.83228817460178,20.8405225541277,0.));
#16332=CARTESIAN_POINT('Ctrl Pts',(5.83228817460178,20.8405225541277,21.));
#16333=CARTESIAN_POINT('Ctrl Pts',(5.79556203439644,20.8040773827343,0.));
#16334=CARTESIAN_POINT('Ctrl Pts',(5.79556203439644,20.8040773827343,21.));
#16335=CARTESIAN_POINT('Ctrl Pts',(5.75906566327796,20.7675064905026,0.));
#16336=CARTESIAN_POINT('Ctrl Pts',(5.75906566327796,20.7675064905026,21.));
#16337=CARTESIAN_POINT('Ctrl Pts',(5.72280100798241,20.7308101804425,0.));
#16338=CARTESIAN_POINT('Ctrl Pts',(5.72280100798241,20.7308101804425,21.));
#16339=CARTESIAN_POINT('Ctrl Pts',(5.68676990500163,20.6939886877061,0.));
#16340=CARTESIAN_POINT('Ctrl Pts',(5.68676990500163,20.6939886877061,21.));
#16341=CARTESIAN_POINT('Ctrl Pts',(5.65097411164335,20.6570421847033,0.));
#16342=CARTESIAN_POINT('Ctrl Pts',(5.65097411164335,20.6570421847033,21.));
#16343=CARTESIAN_POINT('Ctrl Pts',(5.61541536715149,20.6199707996366,0.));
#16344=CARTESIAN_POINT('Ctrl Pts',(5.61541536715149,20.6199707996366,21.));
#16345=CARTESIAN_POINT('Ctrl Pts',(5.58009544402475,20.5827746317185,0.));
#16346=CARTESIAN_POINT('Ctrl Pts',(5.58009544402475,20.5827746317185,21.));
#16347=CARTESIAN_POINT('Ctrl Pts',(5.5450161968946,20.5454537676144,0.));
#16348=CARTESIAN_POINT('Ctrl Pts',(5.5450161968946,20.5454537676144,21.));
#16349=CARTESIAN_POINT('Ctrl Pts',(5.51017962306782,20.5080083009242,0.));
#16350=CARTESIAN_POINT('Ctrl Pts',(5.51017962306782,20.5080083009242,21.));
#16351=CARTESIAN_POINT('Ctrl Pts',(5.47558784449851,20.4704383353718,0.));
#16352=CARTESIAN_POINT('Ctrl Pts',(5.47558784449851,20.4704383353718,21.));
#16353=CARTESIAN_POINT('Ctrl Pts',(5.44124306065111,20.4327439816542,0.));
#16354=CARTESIAN_POINT('Ctrl Pts',(5.44124306065111,20.4327439816542,21.));
#16355=CARTESIAN_POINT('Ctrl Pts',(5.40714750595875,20.3949253578015,0.));
#16356=CARTESIAN_POINT('Ctrl Pts',(5.40714750595875,20.3949253578015,21.));
#16357=CARTESIAN_POINT('Ctrl Pts',(5.37330341114649,20.3569825877537,0.));
#16358=CARTESIAN_POINT('Ctrl Pts',(5.37330341114649,20.3569825877537,21.));
#16359=CARTESIAN_POINT('Ctrl Pts',(5.33971294212214,20.3189158047642,0.));
#16360=CARTESIAN_POINT('Ctrl Pts',(5.33971294212214,20.3189158047642,21.));
#16361=CARTESIAN_POINT('Ctrl Pts',(5.30637824220998,20.2807251380077,0.));
#16362=CARTESIAN_POINT('Ctrl Pts',(5.30637824220998,20.2807251380077,21.));
#16363=CARTESIAN_POINT('Ctrl Pts',(5.2733015229815,20.2424106921768,0.));
#16364=CARTESIAN_POINT('Ctrl Pts',(5.2733015229815,20.2424106921768,21.));
#16365=CARTESIAN_POINT('Ctrl Pts',(5.24048514441891,20.2039725283917,0.));
#16366=CARTESIAN_POINT('Ctrl Pts',(5.24048514441891,20.2039725283917,21.));
#16367=CARTESIAN_POINT('Ctrl Pts',(5.20793168386164,20.1654106491899,0.));
#16368=CARTESIAN_POINT('Ctrl Pts',(5.20793168386164,20.1654106491899,21.));
#16369=CARTESIAN_POINT('Ctrl Pts',(5.17564404279922,20.1267249732337,0.));
#16370=CARTESIAN_POINT('Ctrl Pts',(5.17564404279922,20.1267249732337,21.));
#16371=CARTESIAN_POINT('Ctrl Pts',(5.14362537555398,20.087915358486,0.));
#16372=CARTESIAN_POINT('Ctrl Pts',(5.14362537555398,20.087915358486,21.));
#16373=CARTESIAN_POINT('Ctrl Pts',(5.11187891582335,20.0489816528155,0.));
#16374=CARTESIAN_POINT('Ctrl Pts',(5.11187891582335,20.0489816528155,21.));
#16375=CARTESIAN_POINT('Ctrl Pts',(5.08040781745337,20.0099237417206,0.));
#16376=CARTESIAN_POINT('Ctrl Pts',(5.08040781745337,20.0099237417206,21.));
#16377=CARTESIAN_POINT('Ctrl Pts',(5.04921502064063,19.9707415879783,0.));
#16378=CARTESIAN_POINT('Ctrl Pts',(5.04921502064063,19.9707415879783,21.));
#16379=CARTESIAN_POINT('Ctrl Pts',(5.01830302225557,19.931435301086,0.));
#16380=CARTESIAN_POINT('Ctrl Pts',(5.01830302225557,19.931435301086,21.));
#16381=CARTESIAN_POINT('Ctrl Pts',(4.98767405031333,19.8920050831202,0.));
#16382=CARTESIAN_POINT('Ctrl Pts',(4.98767405031333,19.8920050831202,21.));
#16383=CARTESIAN_POINT('Ctrl Pts',(4.95733049830096,19.8524510953961,0.));
#16384=CARTESIAN_POINT('Ctrl Pts',(4.95733049830096,19.8524510953961,21.));
#16385=CARTESIAN_POINT('Ctrl Pts',(4.92727531494347,19.8127733387903,0.));
#16386=CARTESIAN_POINT('Ctrl Pts',(4.92727531494347,19.8127733387903,21.));
#16387=CARTESIAN_POINT('Ctrl Pts',(4.89751233527805,19.772971552601,0.));
#16388=CARTESIAN_POINT('Ctrl Pts',(4.89751233527805,19.772971552601,21.));
#16389=CARTESIAN_POINT('Ctrl Pts',(4.86804682289087,19.7330450480715,0.));
#16390=CARTESIAN_POINT('Ctrl Pts',(4.86804682289087,19.7330450480715,21.));
#16391=CARTESIAN_POINT('Ctrl Pts',(4.83888510708974,19.6929928227072,0.));
#16392=CARTESIAN_POINT('Ctrl Pts',(4.83888510708974,19.6929928227072,21.));
#16393=CARTESIAN_POINT('Ctrl Pts',(4.81003361418061,19.6528138625329,0.));
#16394=CARTESIAN_POINT('Ctrl Pts',(4.81003361418061,19.6528138625329,21.));
#16395=CARTESIAN_POINT('Ctrl Pts',(4.7814979936173,19.6125074152527,0.));
#16396=CARTESIAN_POINT('Ctrl Pts',(4.7814979936173,19.6125074152527,21.));
#16397=CARTESIAN_POINT('Ctrl Pts',(4.75328238194611,19.5720732205813,0.));
#16398=CARTESIAN_POINT('Ctrl Pts',(4.75328238194611,19.5720732205813,21.));
#16399=CARTESIAN_POINT('Ctrl Pts',(4.72538815796616,19.531511899192,0.));
#16400=CARTESIAN_POINT('Ctrl Pts',(4.72538815796616,19.531511899192,21.));
#16401=CARTESIAN_POINT('Ctrl Pts',(4.69781487613784,19.4908246636763,0.));
#16402=CARTESIAN_POINT('Ctrl Pts',(4.69781487613784,19.4908246636763,21.));
#16403=CARTESIAN_POINT('Ctrl Pts',(4.67056260851453,19.4500125912299,0.));
#16404=CARTESIAN_POINT('Ctrl Pts',(4.67056260851453,19.4500125912299,21.));
#16405=CARTESIAN_POINT('Ctrl Pts',(4.64363405547472,19.4090759683639,0.));
#16406=CARTESIAN_POINT('Ctrl Pts',(4.64363405547472,19.4090759683639,21.));
#16407=CARTESIAN_POINT('Ctrl Pts',(4.61703633725712,19.3680137353983,0.));
#16408=CARTESIAN_POINT('Ctrl Pts',(4.61703633725712,19.3680137353983,21.));
#16409=CARTESIAN_POINT('Ctrl Pts',(4.59078395765677,19.3268225655679,0.));
#16410=CARTESIAN_POINT('Ctrl Pts',(4.59078395765677,19.3268225655679,21.));
#16411=CARTESIAN_POINT('Ctrl Pts',(4.56489651606741,19.2854975819105,0.));
#16412=CARTESIAN_POINT('Ctrl Pts',(4.56489651606741,19.2854975819105,21.));
#16413=CARTESIAN_POINT('Ctrl Pts',(4.53939338835152,19.2440340196551,0.));
#16414=CARTESIAN_POINT('Ctrl Pts',(4.53939338835152,19.2440340196551,21.));
#16415=CARTESIAN_POINT('Ctrl Pts',(4.51428889122955,19.2024287376926,0.));
#16416=CARTESIAN_POINT('Ctrl Pts',(4.51428889122955,19.2024287376926,21.));
#16417=CARTESIAN_POINT('Ctrl Pts',(4.48958819710577,19.1606814968494,0.));
#16418=CARTESIAN_POINT('Ctrl Pts',(4.48958819710577,19.1606814968494,21.));
#16419=CARTESIAN_POINT('Ctrl Pts',(4.46528051067021,19.1187970904933,0.));
#16420=CARTESIAN_POINT('Ctrl Pts',(4.46528051067021,19.1187970904933,21.));
#16421=CARTESIAN_POINT('Ctrl Pts',(4.44134542994082,19.0767833717249,0.));
#16422=CARTESIAN_POINT('Ctrl Pts',(4.44134542994082,19.0767833717249,21.));
#16423=CARTESIAN_POINT('Ctrl Pts',(4.41776558033332,19.034647328575,0.));
#16424=CARTESIAN_POINT('Ctrl Pts',(4.41776558033332,19.034647328575,21.));
#16425=CARTESIAN_POINT('Ctrl Pts',(4.39453820875555,18.9923914823906,0.));
#16426=CARTESIAN_POINT('Ctrl Pts',(4.39453820875555,18.9923914823906,21.));
#16427=CARTESIAN_POINT('Ctrl Pts',(4.37168516143123,18.9500107909187,0.));
#16428=CARTESIAN_POINT('Ctrl Pts',(4.37168516143123,18.9500107909187,21.));
#16429=CARTESIAN_POINT('Ctrl Pts',(4.34926881342022,18.9074876952706,0.));
#16430=CARTESIAN_POINT('Ctrl Pts',(4.34926881342022,18.9074876952706,21.));
#16431=CARTESIAN_POINT('Ctrl Pts',(4.32737526247704,18.8647973781745,0.));
#16432=CARTESIAN_POINT('Ctrl Pts',(4.32737526247704,18.8647973781745,21.));
#16433=CARTESIAN_POINT('Ctrl Pts',(4.30608591031526,18.8219166495975,0.));
#16434=CARTESIAN_POINT('Ctrl Pts',(4.30608591031526,18.8219166495975,21.));
#16435=CARTESIAN_POINT('Ctrl Pts',(4.28545098663153,18.778832216358,0.));
#16436=CARTESIAN_POINT('Ctrl Pts',(4.28545098663153,18.778832216358,21.));
#16437=CARTESIAN_POINT('Ctrl Pts',(4.26546636161933,18.735547949685,0.));
#16438=CARTESIAN_POINT('Ctrl Pts',(4.26546636161933,18.735547949685,21.));
#16439=CARTESIAN_POINT('Ctrl Pts',(4.24603817988452,18.6920958920047,0.));
#16440=CARTESIAN_POINT('Ctrl Pts',(4.24603817988452,18.6920958920047,21.));
#16441=CARTESIAN_POINT('Ctrl Pts',(4.22703266508919,18.6485210883348,0.));
#16442=CARTESIAN_POINT('Ctrl Pts',(4.22703266508919,18.6485210883348,21.));
#16443=CARTESIAN_POINT('Ctrl Pts',(4.20834600700665,18.6048602364653,0.));
#16444=CARTESIAN_POINT('Ctrl Pts',(4.20834600700665,18.6048602364653,21.));
#16445=CARTESIAN_POINT('Ctrl Pts',(4.18996967278621,18.5611217636409,0.));
#16446=CARTESIAN_POINT('Ctrl Pts',(4.18996967278621,18.5611217636409,21.));
#16447=CARTESIAN_POINT('Ctrl Pts',(4.17205262766562,18.5172668097744,0.));
#16448=CARTESIAN_POINT('Ctrl Pts',(4.17205262766562,18.5172668097744,21.));
#16449=CARTESIAN_POINT('Ctrl Pts',(4.15497867673974,18.4731856794913,0.));
#16450=CARTESIAN_POINT('Ctrl Pts',(4.15497867673974,18.4731856794913,21.));
#16451=CARTESIAN_POINT('Ctrl Pts',(4.13926275457062,18.4287286547442,0.));
#16452=CARTESIAN_POINT('Ctrl Pts',(4.13926275457062,18.4287286547442,21.));
#16453=CARTESIAN_POINT('Ctrl Pts',(4.12819301671079,18.3927403741815,0.));
#16454=CARTESIAN_POINT('Ctrl Pts',(4.12819301671079,18.3927403741815,21.));
#16455=CARTESIAN_POINT('Ctrl Pts',(4.1209201986886,18.3654573320481,0.));
#16456=CARTESIAN_POINT('Ctrl Pts',(4.1209201986886,18.3654573320481,21.));
#16457=CARTESIAN_POINT('Ctrl Pts',(4.11655269114951,18.3471320125699,0.));
#16458=CARTESIAN_POINT('Ctrl Pts',(4.11655269114951,18.3471320125699,21.));
#16459=CARTESIAN_POINT('Ctrl Pts',(4.11448919812531,18.337935196262,0.));
#16460=CARTESIAN_POINT('Ctrl Pts',(4.11448919812531,18.337935196262,21.));
#16461=CARTESIAN_POINT('',(6.13422273260085,21.1275013067529,0.));
#16462=CARTESIAN_POINT('Ctrl Pts',(4.11448919812531,18.337935196262,0.));
#16463=CARTESIAN_POINT('Ctrl Pts',(4.11655269114951,18.3471320125699,0.));
#16464=CARTESIAN_POINT('Ctrl Pts',(4.1209201986886,18.3654573320481,0.));
#16465=CARTESIAN_POINT('Ctrl Pts',(4.12819301671079,18.3927403741815,0.));
#16466=CARTESIAN_POINT('Ctrl Pts',(4.13926275457062,18.4287286547442,0.));
#16467=CARTESIAN_POINT('Ctrl Pts',(4.15497867673974,18.4731856794913,0.));
#16468=CARTESIAN_POINT('Ctrl Pts',(4.17205262766562,18.5172668097744,0.));
#16469=CARTESIAN_POINT('Ctrl Pts',(4.18996967278621,18.5611217636409,0.));
#16470=CARTESIAN_POINT('Ctrl Pts',(4.20834600700665,18.6048602364653,0.));
#16471=CARTESIAN_POINT('Ctrl Pts',(4.22703266508919,18.6485210883348,0.));
#16472=CARTESIAN_POINT('Ctrl Pts',(4.24603817988452,18.6920958920047,0.));
#16473=CARTESIAN_POINT('Ctrl Pts',(4.26546636161933,18.735547949685,0.));
#16474=CARTESIAN_POINT('Ctrl Pts',(4.28545098663153,18.778832216358,0.));
#16475=CARTESIAN_POINT('Ctrl Pts',(4.30608591031526,18.8219166495975,0.));
#16476=CARTESIAN_POINT('Ctrl Pts',(4.32737526247704,18.8647973781745,0.));
#16477=CARTESIAN_POINT('Ctrl Pts',(4.34926881342022,18.9074876952706,0.));
#16478=CARTESIAN_POINT('Ctrl Pts',(4.37168516143123,18.9500107909187,0.));
#16479=CARTESIAN_POINT('Ctrl Pts',(4.39453820875555,18.9923914823906,0.));
#16480=CARTESIAN_POINT('Ctrl Pts',(4.41776558033332,19.034647328575,0.));
#16481=CARTESIAN_POINT('Ctrl Pts',(4.44134542994082,19.0767833717249,0.));
#16482=CARTESIAN_POINT('Ctrl Pts',(4.46528051067021,19.1187970904933,0.));
#16483=CARTESIAN_POINT('Ctrl Pts',(4.48958819710577,19.1606814968494,0.));
#16484=CARTESIAN_POINT('Ctrl Pts',(4.51428889122955,19.2024287376926,0.));
#16485=CARTESIAN_POINT('Ctrl Pts',(4.53939338835152,19.2440340196551,0.));
#16486=CARTESIAN_POINT('Ctrl Pts',(4.56489651606741,19.2854975819105,0.));
#16487=CARTESIAN_POINT('Ctrl Pts',(4.59078395765677,19.3268225655679,0.));
#16488=CARTESIAN_POINT('Ctrl Pts',(4.61703633725712,19.3680137353983,0.));
#16489=CARTESIAN_POINT('Ctrl Pts',(4.64363405547472,19.4090759683639,0.));
#16490=CARTESIAN_POINT('Ctrl Pts',(4.67056260851453,19.4500125912299,0.));
#16491=CARTESIAN_POINT('Ctrl Pts',(4.69781487613784,19.4908246636763,0.));
#16492=CARTESIAN_POINT('Ctrl Pts',(4.72538815796616,19.531511899192,0.));
#16493=CARTESIAN_POINT('Ctrl Pts',(4.75328238194611,19.5720732205813,0.));
#16494=CARTESIAN_POINT('Ctrl Pts',(4.7814979936173,19.6125074152527,0.));
#16495=CARTESIAN_POINT('Ctrl Pts',(4.81003361418061,19.6528138625329,0.));
#16496=CARTESIAN_POINT('Ctrl Pts',(4.83888510708974,19.6929928227072,0.));
#16497=CARTESIAN_POINT('Ctrl Pts',(4.86804682289087,19.7330450480715,0.));
#16498=CARTESIAN_POINT('Ctrl Pts',(4.89751233527805,19.772971552601,0.));
#16499=CARTESIAN_POINT('Ctrl Pts',(4.92727531494347,19.8127733387903,0.));
#16500=CARTESIAN_POINT('Ctrl Pts',(4.95733049830096,19.8524510953961,0.));
#16501=CARTESIAN_POINT('Ctrl Pts',(4.98767405031333,19.8920050831202,0.));
#16502=CARTESIAN_POINT('Ctrl Pts',(5.01830302225557,19.931435301086,0.));
#16503=CARTESIAN_POINT('Ctrl Pts',(5.04921502064063,19.9707415879783,0.));
#16504=CARTESIAN_POINT('Ctrl Pts',(5.08040781745337,20.0099237417206,0.));
#16505=CARTESIAN_POINT('Ctrl Pts',(5.11187891582335,20.0489816528155,0.));
#16506=CARTESIAN_POINT('Ctrl Pts',(5.14362537555398,20.087915358486,0.));
#16507=CARTESIAN_POINT('Ctrl Pts',(5.17564404279922,20.1267249732337,0.));
#16508=CARTESIAN_POINT('Ctrl Pts',(5.20793168386164,20.1654106491899,0.));
#16509=CARTESIAN_POINT('Ctrl Pts',(5.24048514441891,20.2039725283917,0.));
#16510=CARTESIAN_POINT('Ctrl Pts',(5.2733015229815,20.2424106921768,0.));
#16511=CARTESIAN_POINT('Ctrl Pts',(5.30637824220998,20.2807251380077,0.));
#16512=CARTESIAN_POINT('Ctrl Pts',(5.33971294212214,20.3189158047642,0.));
#16513=CARTESIAN_POINT('Ctrl Pts',(5.37330341114649,20.3569825877537,0.));
#16514=CARTESIAN_POINT('Ctrl Pts',(5.40714750595875,20.3949253578015,0.));
#16515=CARTESIAN_POINT('Ctrl Pts',(5.44124306065111,20.4327439816542,0.));
#16516=CARTESIAN_POINT('Ctrl Pts',(5.47558784449851,20.4704383353718,0.));
#16517=CARTESIAN_POINT('Ctrl Pts',(5.51017962306782,20.5080083009242,0.));
#16518=CARTESIAN_POINT('Ctrl Pts',(5.5450161968946,20.5454537676144,0.));
#16519=CARTESIAN_POINT('Ctrl Pts',(5.58009544402475,20.5827746317185,0.));
#16520=CARTESIAN_POINT('Ctrl Pts',(5.61541536715149,20.6199707996366,0.));
#16521=CARTESIAN_POINT('Ctrl Pts',(5.65097411164335,20.6570421847033,0.));
#16522=CARTESIAN_POINT('Ctrl Pts',(5.68676990500163,20.6939886877061,0.));
#16523=CARTESIAN_POINT('Ctrl Pts',(5.72280100798241,20.7308101804425,0.));
#16524=CARTESIAN_POINT('Ctrl Pts',(5.75906566327796,20.7675064905026,0.));
#16525=CARTESIAN_POINT('Ctrl Pts',(5.79556203439644,20.8040773827343,0.));
#16526=CARTESIAN_POINT('Ctrl Pts',(5.83228817460178,20.8405225541277,0.));
#16527=CARTESIAN_POINT('Ctrl Pts',(5.86924212736288,20.8768416821402,0.));
#16528=CARTESIAN_POINT('Ctrl Pts',(5.906422006626,20.9130344665641,0.));
#16529=CARTESIAN_POINT('Ctrl Pts',(5.94382608200804,20.9491006734021,0.));
#16530=CARTESIAN_POINT('Ctrl Pts',(5.98145286361837,20.9850401822713,0.));
#16531=CARTESIAN_POINT('Ctrl Pts',(6.02687083887287,21.0280155918661,0.));
#16532=CARTESIAN_POINT('Ctrl Pts',(6.06499496148845,21.0636702474951,0.));
#16533=CARTESIAN_POINT('Ctrl Pts',(6.09567013127872,21.0920928984154,0.));
#16534=CARTESIAN_POINT('Ctrl Pts',(6.11877533761501,21.1133530893457,0.));
#16535=CARTESIAN_POINT('Ctrl Pts',(6.13422273260091,21.1275013067528,0.));
#16536=CARTESIAN_POINT('',(6.13422273260085,21.1275013067529,13.));
#16537=CARTESIAN_POINT('Ctrl Pts',(6.13422273260091,21.1275013067528,13.));
#16538=CARTESIAN_POINT('Ctrl Pts',(6.05818207473574,21.0578559224639,13.));
#16539=CARTESIAN_POINT('Ctrl Pts',(5.98341417184728,20.9874765040291,13.));
#16540=CARTESIAN_POINT('Ctrl Pts',(5.90994468705573,20.9163599154701,13.));
#16541=CARTESIAN_POINT('Ctrl Pts',(5.78820256793375,20.7985166473367,13.));
#16542=CARTESIAN_POINT('Ctrl Pts',(5.67003811891006,20.6786545089329,13.));
#16543=CARTESIAN_POINT('Ctrl Pts',(5.55573863837942,20.5568062999927,13.));
#16544=CARTESIAN_POINT('Ctrl Pts',(5.46788135576792,20.4631466221109,13.));
#16545=CARTESIAN_POINT('Ctrl Pts',(5.38230707228741,20.3683108766733,13.));
#16546=CARTESIAN_POINT('Ctrl Pts',(5.29917141508608,20.2723075580748,13.));
#16547=CARTESIAN_POINT('Ctrl Pts',(5.20967788534761,20.1689623012113,13.));
#16548=CARTESIAN_POINT('Ctrl Pts',(5.12300395967644,20.064265111617,13.));
#16549=CARTESIAN_POINT('Ctrl Pts',(5.03941267492058,19.9582092059413,13.));
#16550=CARTESIAN_POINT('Ctrl Pts',(4.9931342664069,19.8994937723589,13.));
#16551=CARTESIAN_POINT('Ctrl Pts',(4.94779583855815,19.8403635590138,13.));
#16552=CARTESIAN_POINT('Ctrl Pts',(4.90344584338495,19.7808173191098,13.));
#16553=CARTESIAN_POINT('Ctrl Pts',(4.86070845303356,19.7234362328482,13.));
#16554=CARTESIAN_POINT('Ctrl Pts',(4.81889538663267,19.6656667932077,13.));
#16555=CARTESIAN_POINT('Ctrl Pts',(4.77808296591823,19.6074986363137,13.));
#16556=CARTESIAN_POINT('Ctrl Pts',(4.74280851516602,19.5572235056112,13.));
#16557=CARTESIAN_POINT('Ctrl Pts',(4.70827845343013,19.5066514996463,13.));
#16558=CARTESIAN_POINT('Ctrl Pts',(4.67449772183394,19.4557905178253,13.));
#16559=CARTESIAN_POINT('Ctrl Pts',(4.65025481932131,19.4192898925955,13.));
#16560=CARTESIAN_POINT('Ctrl Pts',(4.62639514873701,19.3826412892821,13.));
#16561=CARTESIAN_POINT('Ctrl Pts',(4.60295743098886,19.3458364388947,13.));
#16562=CARTESIAN_POINT('Ctrl Pts',(4.57990136672579,19.309630908781,13.));
#16563=CARTESIAN_POINT('Ctrl Pts',(4.55725972003952,19.2732722738433,13.));
#16564=CARTESIAN_POINT('Ctrl Pts',(4.53508357570349,19.2367485577747,13.));
#16565=CARTESIAN_POINT('Ctrl Pts',(4.51585555588996,19.2050803504619,13.));
#16566=CARTESIAN_POINT('Ctrl Pts',(4.49697986260364,19.1732873013817,13.));
#16567=CARTESIAN_POINT('Ctrl Pts',(4.47844262266263,19.1413765621746,13.));
#16568=CARTESIAN_POINT('Ctrl Pts',(4.46165213672774,19.1124727545132,13.));
#16569=CARTESIAN_POINT('Ctrl Pts',(4.44513401132745,19.0834740457553,13.));
#16570=CARTESIAN_POINT('Ctrl Pts',(4.42886646477444,19.0543895553857,13.));
#16571=CARTESIAN_POINT('Ctrl Pts',(4.41516354273523,19.0298903168075,13.));
#16572=CARTESIAN_POINT('Ctrl Pts',(4.4016367609421,19.0053307307673,13.));
#16573=CARTESIAN_POINT('Ctrl Pts',(4.3883055171539,18.9807063065615,13.));
#16574=CARTESIAN_POINT('Ctrl Pts',(4.36901375650801,18.9450720847762,13.));
#16575=CARTESIAN_POINT('Ctrl Pts',(4.35013223001517,18.9093017976082,13.));
#16576=CARTESIAN_POINT('Ctrl Pts',(4.33187128665099,18.8733353263476,13.));
#16577=CARTESIAN_POINT('Ctrl Pts',(4.32083731650082,18.8516029896122,13.));
#16578=CARTESIAN_POINT('Ctrl Pts',(4.31003325580781,18.8297980041067,13.));
#16579=CARTESIAN_POINT('Ctrl Pts',(4.29948469299916,18.8079138028469,13.));
#16580=CARTESIAN_POINT('Ctrl Pts',(4.28975595055798,18.7877304128013,13.));
#16581=CARTESIAN_POINT('Ctrl Pts',(4.2802457999774,18.7674792480964,13.));
#16582=CARTESIAN_POINT('Ctrl Pts',(4.27093067973601,18.7471689056956,13.));
#16583=CARTESIAN_POINT('Ctrl Pts',(4.25811678806992,18.7192299719535,13.));
#16584=CARTESIAN_POINT('Ctrl Pts',(4.24566493397902,18.6911811213441,13.));
#16585=CARTESIAN_POINT('Ctrl Pts',(4.23343245343651,18.66307117359,13.));
#16586=CARTESIAN_POINT('Ctrl Pts',(4.22567194943085,18.6452377209729,13.));
#16587=CARTESIAN_POINT('Ctrl Pts',(4.21799814921963,18.6273802008541,13.));
#16588=CARTESIAN_POINT('Ctrl Pts',(4.21040342108918,18.6095026819599,13.));
#16589=CARTESIAN_POINT('Ctrl Pts',(4.20358750609861,18.5934584408847,13.));
#16590=CARTESIAN_POINT('Ctrl Pts',(4.19683458198288,18.5773983085052,13.));
#16591=CARTESIAN_POINT('Ctrl Pts',(4.19017810368263,18.561313537851,13.));
#16592=CARTESIAN_POINT('Ctrl Pts',(4.18318081928036,18.5444052404397,13.));
#16593=CARTESIAN_POINT('Ctrl Pts',(4.17628995976728,18.5274697699695,13.));
#16594=CARTESIAN_POINT('Ctrl Pts',(4.16960404102764,18.5104789585715,13.));
#16595=CARTESIAN_POINT('Ctrl Pts',(4.15849874476065,18.4822572583475,13.));
#16596=CARTESIAN_POINT('Ctrl Pts',(4.14796697295334,18.4538805850238,13.));
#16597=CARTESIAN_POINT('Ctrl Pts',(4.13860964460812,18.4251735640121,13.));
#16598=CARTESIAN_POINT('Ctrl Pts',(4.1334496807422,18.4093434909769,13.));
#16599=CARTESIAN_POINT('Ctrl Pts',(4.12864814561696,18.3934125378817,13.));
#16600=CARTESIAN_POINT('Ctrl Pts',(4.12427889810931,18.3773590065429,13.));
#16601=CARTESIAN_POINT('Ctrl Pts',(4.12072474060618,18.3643002867611,13.));
#16602=CARTESIAN_POINT('Ctrl Pts',(4.11745655843541,18.3511604736782,13.));
#16603=CARTESIAN_POINT('Ctrl Pts',(4.11448919812531,18.337935196262,13.));
#16604=CARTESIAN_POINT('',(6.13422273260085,21.1275013067529,0.));
#16605=CARTESIAN_POINT('Origin',(1.75106900012182E-12,5.38923623413286E-12,
0.));
#16606=CARTESIAN_POINT('',(7.45574324794401,20.698113262342,0.));
#16607=CARTESIAN_POINT('Origin',(1.75106900012182E-12,5.38923623413286E-12,
0.));
#16608=CARTESIAN_POINT('',(7.45574324794401,20.698113262342,13.));
#16609=CARTESIAN_POINT('Origin',(1.75106900012182E-12,5.38923623413286E-12,
13.));
#16610=CARTESIAN_POINT('',(7.45574324794401,20.698113262342,0.));
#16611=CARTESIAN_POINT('Ctrl Pts',(7.45007618140239,17.2541372868972,0.));
#16612=CARTESIAN_POINT('Ctrl Pts',(7.45007618140239,17.2541372868972,21.));
#16613=CARTESIAN_POINT('Ctrl Pts',(7.45381253347183,17.2627905583523,0.));
#16614=CARTESIAN_POINT('Ctrl Pts',(7.45381253347183,17.2627905583523,21.));
#16615=CARTESIAN_POINT('Ctrl Pts',(7.46105049818251,17.2801832097582,0.));
#16616=CARTESIAN_POINT('Ctrl Pts',(7.46105049818251,17.2801832097582,21.));
#16617=CARTESIAN_POINT('Ctrl Pts',(7.4712032346092,17.3065305096784,0.));
#16618=CARTESIAN_POINT('Ctrl Pts',(7.4712032346092,17.3065305096784,21.));
#16619=CARTESIAN_POINT('Ctrl Pts',(7.48340100912745,17.3421522689127,0.));
#16620=CARTESIAN_POINT('Ctrl Pts',(7.48340100912745,17.3421522689127,21.));
#16621=CARTESIAN_POINT('Ctrl Pts',(7.49681774451751,17.3873563447297,0.));
#16622=CARTESIAN_POINT('Ctrl Pts',(7.49681774451751,17.3873563447297,21.));
#16623=CARTESIAN_POINT('Ctrl Pts',(7.50891486634214,17.4330545448126,0.));
#16624=CARTESIAN_POINT('Ctrl Pts',(7.50891486634214,17.4330545448126,21.));
#16625=CARTESIAN_POINT('Ctrl Pts',(7.52019696747329,17.4790653226646,0.));
#16626=CARTESIAN_POINT('Ctrl Pts',(7.52019696747329,17.4790653226646,21.));
#16627=CARTESIAN_POINT('Ctrl Pts',(7.53103903007864,17.5252518287336,0.));
#16628=CARTESIAN_POINT('Ctrl Pts',(7.53103903007864,17.5252518287336,21.));
#16629=CARTESIAN_POINT('Ctrl Pts',(7.54158441095317,17.5715579419204,0.));
#16630=CARTESIAN_POINT('Ctrl Pts',(7.54158441095317,17.5715579419204,21.));
#16631=CARTESIAN_POINT('Ctrl Pts',(7.55182125346564,17.6179818599248,0.));
#16632=CARTESIAN_POINT('Ctrl Pts',(7.55182125346564,17.6179818599248,21.));
#16633=CARTESIAN_POINT('Ctrl Pts',(7.56164400295863,17.6645549117314,0.));
#16634=CARTESIAN_POINT('Ctrl Pts',(7.56164400295863,17.6645549117314,21.));
#16635=CARTESIAN_POINT('Ctrl Pts',(7.57091795530423,17.7113192869136,0.));
#16636=CARTESIAN_POINT('Ctrl Pts',(7.57091795530423,17.7113192869136,21.));
#16637=CARTESIAN_POINT('Ctrl Pts',(7.57954834582804,17.7583042294209,0.));
#16638=CARTESIAN_POINT('Ctrl Pts',(7.57954834582804,17.7583042294209,21.));
#16639=CARTESIAN_POINT('Ctrl Pts',(7.58752955799499,17.8055090348024,0.));
#16640=CARTESIAN_POINT('Ctrl Pts',(7.58752955799499,17.8055090348024,21.));
#16641=CARTESIAN_POINT('Ctrl Pts',(7.59491004201956,17.8529149331931,0.));
#16642=CARTESIAN_POINT('Ctrl Pts',(7.59491004201956,17.8529149331931,21.));
#16643=CARTESIAN_POINT('Ctrl Pts',(7.60176928403058,17.900492838997,0.));
#16644=CARTESIAN_POINT('Ctrl Pts',(7.60176928403058,17.900492838997,21.));
#16645=CARTESIAN_POINT('Ctrl Pts',(7.60819152580111,17.9482122228183,0.));
#16646=CARTESIAN_POINT('Ctrl Pts',(7.60819152580111,17.9482122228183,21.));
#16647=CARTESIAN_POINT('Ctrl Pts',(7.61423755067038,17.9960506269561,0.));
#16648=CARTESIAN_POINT('Ctrl Pts',(7.61423755067038,17.9960506269561,21.));
#16649=CARTESIAN_POINT('Ctrl Pts',(7.61992799636654,18.0439992897906,0.));
#16650=CARTESIAN_POINT('Ctrl Pts',(7.61992799636654,18.0439992897906,21.));
#16651=CARTESIAN_POINT('Ctrl Pts',(7.62525915358074,18.0920577897363,0.));
#16652=CARTESIAN_POINT('Ctrl Pts',(7.62525915358074,18.0920577897363,21.));
#16653=CARTESIAN_POINT('Ctrl Pts',(7.63021285851762,18.1402306858819,0.));
#16654=CARTESIAN_POINT('Ctrl Pts',(7.63021285851762,18.1402306858819,21.));
#16655=CARTESIAN_POINT('Ctrl Pts',(7.63476798969017,18.1885236169197,0.));
#16656=CARTESIAN_POINT('Ctrl Pts',(7.63476798969017,18.1885236169197,21.));
#16657=CARTESIAN_POINT('Ctrl Pts',(7.63891299603827,18.2369390502576,0.));
#16658=CARTESIAN_POINT('Ctrl Pts',(7.63891299603827,18.2369390502576,21.));
#16659=CARTESIAN_POINT('Ctrl Pts',(7.6426522027076,18.2854741391282,0.));
#16660=CARTESIAN_POINT('Ctrl Pts',(7.6426522027076,18.2854741391282,21.));
#16661=CARTESIAN_POINT('Ctrl Pts',(7.64599903846601,18.3341230095852,0.));
#16662=CARTESIAN_POINT('Ctrl Pts',(7.64599903846601,18.3341230095852,21.));
#16663=CARTESIAN_POINT('Ctrl Pts',(7.6489719793775,18.3828781275628,0.));
#16664=CARTESIAN_POINT('Ctrl Pts',(7.6489719793775,18.3828781275628,21.));
#16665=CARTESIAN_POINT('Ctrl Pts',(7.65158974829126,18.4317319183719,0.));
#16666=CARTESIAN_POINT('Ctrl Pts',(7.65158974829126,18.4317319183719,21.));
#16667=CARTESIAN_POINT('Ctrl Pts',(7.65386603444743,18.4806785483052,0.));
#16668=CARTESIAN_POINT('Ctrl Pts',(7.65386603444743,18.4806785483052,21.));
#16669=CARTESIAN_POINT('Ctrl Pts',(7.65580722110437,18.5297146894905,0.));
#16670=CARTESIAN_POINT('Ctrl Pts',(7.65580722110437,18.5297146894905,21.));
#16671=CARTESIAN_POINT('Ctrl Pts',(7.65741532450727,18.5788385228928,0.));
#16672=CARTESIAN_POINT('Ctrl Pts',(7.65741532450727,18.5788385228928,21.));
#16673=CARTESIAN_POINT('Ctrl Pts',(7.65868976978872,18.6280491346907,0.));
#16674=CARTESIAN_POINT('Ctrl Pts',(7.65868976978872,18.6280491346907,21.));
#16675=CARTESIAN_POINT('Ctrl Pts',(7.65962948375621,18.6773458057584,0.));
#16676=CARTESIAN_POINT('Ctrl Pts',(7.65962948375621,18.6773458057584,21.));
#16677=CARTESIAN_POINT('Ctrl Pts',(7.66023521705905,18.7267272235231,0.));
#16678=CARTESIAN_POINT('Ctrl Pts',(7.66023521705905,18.7267272235231,21.));
#16679=CARTESIAN_POINT('Ctrl Pts',(7.66051046922541,18.7761911671591,0.));
#16680=CARTESIAN_POINT('Ctrl Pts',(7.66051046922541,18.7761911671591,21.));
#16681=CARTESIAN_POINT('Ctrl Pts',(7.66046025294775,18.8257349246207,0.));
#16682=CARTESIAN_POINT('Ctrl Pts',(7.66046025294775,18.8257349246207,21.));
#16683=CARTESIAN_POINT('Ctrl Pts',(7.66009036321663,18.8753555389435,0.));
#16684=CARTESIAN_POINT('Ctrl Pts',(7.66009036321663,18.8753555389435,21.));
#16685=CARTESIAN_POINT('Ctrl Pts',(7.65940650980099,18.9250501008887,0.));
#16686=CARTESIAN_POINT('Ctrl Pts',(7.65940650980099,18.9250501008887,21.));
#16687=CARTESIAN_POINT('Ctrl Pts',(7.65841335587266,18.974816073814,0.));
#16688=CARTESIAN_POINT('Ctrl Pts',(7.65841335587266,18.974816073814,21.));
#16689=CARTESIAN_POINT('Ctrl Pts',(7.65711415727855,19.0246514144531,0.));
#16690=CARTESIAN_POINT('Ctrl Pts',(7.65711415727855,19.0246514144531,21.));
#16691=CARTESIAN_POINT('Ctrl Pts',(7.65551129907202,19.0745543888799,0.));
#16692=CARTESIAN_POINT('Ctrl Pts',(7.65551129907202,19.0745543888799,21.));
#16693=CARTESIAN_POINT('Ctrl Pts',(7.65360662280609,19.1245234597312,0.));
#16694=CARTESIAN_POINT('Ctrl Pts',(7.65360662280609,19.1245234597312,21.));
#16695=CARTESIAN_POINT('Ctrl Pts',(7.65140181220526,19.1745571539291,0.));
#16696=CARTESIAN_POINT('Ctrl Pts',(7.65140181220526,19.1745571539291,21.));
#16697=CARTESIAN_POINT('Ctrl Pts',(7.64889882291924,19.224653915265,0.));
#16698=CARTESIAN_POINT('Ctrl Pts',(7.64889882291924,19.224653915265,21.));
#16699=CARTESIAN_POINT('Ctrl Pts',(7.64610005549614,19.2748120456486,0.));
#16700=CARTESIAN_POINT('Ctrl Pts',(7.64610005549614,19.2748120456486,21.));
#16701=CARTESIAN_POINT('Ctrl Pts',(7.64300812875339,19.3250297839295,0.));
#16702=CARTESIAN_POINT('Ctrl Pts',(7.64300812875339,19.3250297839295,21.));
#16703=CARTESIAN_POINT('Ctrl Pts',(7.63962574822761,19.3753053524647,0.));
#16704=CARTESIAN_POINT('Ctrl Pts',(7.63962574822761,19.3753053524647,21.));
#16705=CARTESIAN_POINT('Ctrl Pts',(7.63595554930654,19.4256370121006,0.));
#16706=CARTESIAN_POINT('Ctrl Pts',(7.63595554930654,19.4256370121006,21.));
#16707=CARTESIAN_POINT('Ctrl Pts',(7.63199992715366,19.4760231231881,0.));
#16708=CARTESIAN_POINT('Ctrl Pts',(7.63199992715366,19.4760231231881,21.));
#16709=CARTESIAN_POINT('Ctrl Pts',(7.62776096538883,19.5264621687521,0.));
#16710=CARTESIAN_POINT('Ctrl Pts',(7.62776096538883,19.5264621687521,21.));
#16711=CARTESIAN_POINT('Ctrl Pts',(7.6232405373522,19.5769527121826,0.));
#16712=CARTESIAN_POINT('Ctrl Pts',(7.6232405373522,19.5769527121826,21.));
#16713=CARTESIAN_POINT('Ctrl Pts',(7.61844037070591,19.6274933688524,0.));
#16714=CARTESIAN_POINT('Ctrl Pts',(7.61844037070591,19.6274933688524,21.));
#16715=CARTESIAN_POINT('Ctrl Pts',(7.61336212350879,19.6780827744426,0.));
#16716=CARTESIAN_POINT('Ctrl Pts',(7.61336212350879,19.6780827744426,21.));
#16717=CARTESIAN_POINT('Ctrl Pts',(7.60800746969262,19.7287195480601,0.));
#16718=CARTESIAN_POINT('Ctrl Pts',(7.60800746969262,19.7287195480601,21.));
#16719=CARTESIAN_POINT('Ctrl Pts',(7.60237814110187,19.7794022782484,0.));
#16720=CARTESIAN_POINT('Ctrl Pts',(7.60237814110187,19.7794022782484,21.));
#16721=CARTESIAN_POINT('Ctrl Pts',(7.59647587605448,19.830129556152,0.));
#16722=CARTESIAN_POINT('Ctrl Pts',(7.59647587605448,19.830129556152,21.));
#16723=CARTESIAN_POINT('Ctrl Pts',(7.59030238888852,19.8808999994024,0.));
#16724=CARTESIAN_POINT('Ctrl Pts',(7.59030238888852,19.8808999994024,21.));
#16725=CARTESIAN_POINT('Ctrl Pts',(7.58385933533352,19.931712276832,0.));
#16726=CARTESIAN_POINT('Ctrl Pts',(7.58385933533352,19.931712276832,21.));
#16727=CARTESIAN_POINT('Ctrl Pts',(7.57714827622806,19.9825651387294,0.));
#16728=CARTESIAN_POINT('Ctrl Pts',(7.57714827622806,19.9825651387294,21.));
#16729=CARTESIAN_POINT('Ctrl Pts',(7.57017066105973,20.0334574248557,0.));
#16730=CARTESIAN_POINT('Ctrl Pts',(7.57017066105973,20.0334574248557,21.));
#16731=CARTESIAN_POINT('Ctrl Pts',(7.5629278654946,20.0843880130978,0.));
#16732=CARTESIAN_POINT('Ctrl Pts',(7.5629278654946,20.0843880130978,21.));
#16733=CARTESIAN_POINT('Ctrl Pts',(7.55542122125495,20.1353557774357,0.));
#16734=CARTESIAN_POINT('Ctrl Pts',(7.55542122125495,20.1353557774357,21.));
#16735=CARTESIAN_POINT('Ctrl Pts',(7.54765204869254,20.1863595454674,0.));
#16736=CARTESIAN_POINT('Ctrl Pts',(7.54765204869254,20.1863595454674,21.));
#16737=CARTESIAN_POINT('Ctrl Pts',(7.53962169534167,20.2373980474879,0.));
#16738=CARTESIAN_POINT('Ctrl Pts',(7.53962169534167,20.2373980474879,21.));
#16739=CARTESIAN_POINT('Ctrl Pts',(7.53133155804008,20.2884698940944,0.));
#16740=CARTESIAN_POINT('Ctrl Pts',(7.53133155804008,20.2884698940944,21.));
#16741=CARTESIAN_POINT('Ctrl Pts',(7.52278303006887,20.3395736743243,0.));
#16742=CARTESIAN_POINT('Ctrl Pts',(7.52278303006887,20.3395736743243,21.));
#16743=CARTESIAN_POINT('Ctrl Pts',(7.51397746081994,20.3907080367098,0.));
#16744=CARTESIAN_POINT('Ctrl Pts',(7.51397746081994,20.3907080367098,21.));
#16745=CARTESIAN_POINT('Ctrl Pts',(7.50491611266253,20.4418717748497,0.));
#16746=CARTESIAN_POINT('Ctrl Pts',(7.50491611266253,20.4418717748497,21.));
#16747=CARTESIAN_POINT('Ctrl Pts',(7.49560012018406,20.4930639156161,0.));
#16748=CARTESIAN_POINT('Ctrl Pts',(7.49560012018406,20.4930639156161,21.));
#16749=CARTESIAN_POINT('Ctrl Pts',(7.48603045196745,20.5442837929044,0.));
#16750=CARTESIAN_POINT('Ctrl Pts',(7.48603045196745,20.5442837929044,21.));
#16751=CARTESIAN_POINT('Ctrl Pts',(7.47620789245428,20.5955309838521,0.));
#16752=CARTESIAN_POINT('Ctrl Pts',(7.47620789245428,20.5955309838521,21.));
#16753=CARTESIAN_POINT('Ctrl Pts',(7.46814799701906,20.6365504027501,0.));
#16754=CARTESIAN_POINT('Ctrl Pts',(7.46814799701906,20.6365504027501,21.));
#16755=CARTESIAN_POINT('Ctrl Pts',(7.46198969876654,20.6673271112931,0.));
#16756=CARTESIAN_POINT('Ctrl Pts',(7.46198969876654,20.6673271112931,21.));
#16757=CARTESIAN_POINT('Ctrl Pts',(7.45783379370108,20.6878503127065,0.));
#16758=CARTESIAN_POINT('Ctrl Pts',(7.45783379370108,20.6878503127065,21.));
#16759=CARTESIAN_POINT('Ctrl Pts',(7.45574324794401,20.698113262342,0.));
#16760=CARTESIAN_POINT('Ctrl Pts',(7.45574324794401,20.698113262342,21.));
#16761=CARTESIAN_POINT('Ctrl Pts',(7.45007618140239,17.2541372868972,0.));
#16762=CARTESIAN_POINT('Ctrl Pts',(7.45381253347183,17.2627905583523,0.));
#16763=CARTESIAN_POINT('Ctrl Pts',(7.46105049818251,17.2801832097582,0.));
#16764=CARTESIAN_POINT('Ctrl Pts',(7.4712032346092,17.3065305096784,0.));
#16765=CARTESIAN_POINT('Ctrl Pts',(7.48340100912745,17.3421522689127,0.));
#16766=CARTESIAN_POINT('Ctrl Pts',(7.49681774451751,17.3873563447297,0.));
#16767=CARTESIAN_POINT('Ctrl Pts',(7.50891486634214,17.4330545448126,0.));
#16768=CARTESIAN_POINT('Ctrl Pts',(7.52019696747329,17.4790653226646,0.));
#16769=CARTESIAN_POINT('Ctrl Pts',(7.53103903007864,17.5252518287336,0.));
#16770=CARTESIAN_POINT('Ctrl Pts',(7.54158441095317,17.5715579419204,0.));
#16771=CARTESIAN_POINT('Ctrl Pts',(7.55182125346564,17.6179818599248,0.));
#16772=CARTESIAN_POINT('Ctrl Pts',(7.56164400295863,17.6645549117314,0.));
#16773=CARTESIAN_POINT('Ctrl Pts',(7.57091795530423,17.7113192869136,0.));
#16774=CARTESIAN_POINT('Ctrl Pts',(7.57954834582804,17.7583042294209,0.));
#16775=CARTESIAN_POINT('Ctrl Pts',(7.58752955799499,17.8055090348024,0.));
#16776=CARTESIAN_POINT('Ctrl Pts',(7.59491004201956,17.8529149331931,0.));
#16777=CARTESIAN_POINT('Ctrl Pts',(7.60176928403058,17.900492838997,0.));
#16778=CARTESIAN_POINT('Ctrl Pts',(7.60819152580111,17.9482122228183,0.));
#16779=CARTESIAN_POINT('Ctrl Pts',(7.61423755067038,17.9960506269561,0.));
#16780=CARTESIAN_POINT('Ctrl Pts',(7.61992799636654,18.0439992897906,0.));
#16781=CARTESIAN_POINT('Ctrl Pts',(7.62525915358074,18.0920577897363,0.));
#16782=CARTESIAN_POINT('Ctrl Pts',(7.63021285851762,18.1402306858819,0.));
#16783=CARTESIAN_POINT('Ctrl Pts',(7.63476798969017,18.1885236169197,0.));
#16784=CARTESIAN_POINT('Ctrl Pts',(7.63891299603827,18.2369390502576,0.));
#16785=CARTESIAN_POINT('Ctrl Pts',(7.6426522027076,18.2854741391282,0.));
#16786=CARTESIAN_POINT('Ctrl Pts',(7.64599903846601,18.3341230095852,0.));
#16787=CARTESIAN_POINT('Ctrl Pts',(7.6489719793775,18.3828781275628,0.));
#16788=CARTESIAN_POINT('Ctrl Pts',(7.65158974829126,18.4317319183719,0.));
#16789=CARTESIAN_POINT('Ctrl Pts',(7.65386603444743,18.4806785483052,0.));
#16790=CARTESIAN_POINT('Ctrl Pts',(7.65580722110437,18.5297146894905,0.));
#16791=CARTESIAN_POINT('Ctrl Pts',(7.65741532450727,18.5788385228928,0.));
#16792=CARTESIAN_POINT('Ctrl Pts',(7.65868976978872,18.6280491346907,0.));
#16793=CARTESIAN_POINT('Ctrl Pts',(7.65962948375621,18.6773458057584,0.));
#16794=CARTESIAN_POINT('Ctrl Pts',(7.66023521705905,18.7267272235231,0.));
#16795=CARTESIAN_POINT('Ctrl Pts',(7.66051046922541,18.7761911671591,0.));
#16796=CARTESIAN_POINT('Ctrl Pts',(7.66046025294775,18.8257349246207,0.));
#16797=CARTESIAN_POINT('Ctrl Pts',(7.66009036321663,18.8753555389435,0.));
#16798=CARTESIAN_POINT('Ctrl Pts',(7.65940650980099,18.9250501008887,0.));
#16799=CARTESIAN_POINT('Ctrl Pts',(7.65841335587266,18.974816073814,0.));
#16800=CARTESIAN_POINT('Ctrl Pts',(7.65711415727855,19.0246514144531,0.));
#16801=CARTESIAN_POINT('Ctrl Pts',(7.65551129907202,19.0745543888799,0.));
#16802=CARTESIAN_POINT('Ctrl Pts',(7.65360662280609,19.1245234597312,0.));
#16803=CARTESIAN_POINT('Ctrl Pts',(7.65140181220526,19.1745571539291,0.));
#16804=CARTESIAN_POINT('Ctrl Pts',(7.64889882291924,19.224653915265,0.));
#16805=CARTESIAN_POINT('Ctrl Pts',(7.64610005549614,19.2748120456486,0.));
#16806=CARTESIAN_POINT('Ctrl Pts',(7.64300812875339,19.3250297839295,0.));
#16807=CARTESIAN_POINT('Ctrl Pts',(7.63962574822761,19.3753053524647,0.));
#16808=CARTESIAN_POINT('Ctrl Pts',(7.63595554930654,19.4256370121006,0.));
#16809=CARTESIAN_POINT('Ctrl Pts',(7.63199992715366,19.4760231231881,0.));
#16810=CARTESIAN_POINT('Ctrl Pts',(7.62776096538883,19.5264621687521,0.));
#16811=CARTESIAN_POINT('Ctrl Pts',(7.6232405373522,19.5769527121826,0.));
#16812=CARTESIAN_POINT('Ctrl Pts',(7.61844037070591,19.6274933688524,0.));
#16813=CARTESIAN_POINT('Ctrl Pts',(7.61336212350879,19.6780827744426,0.));
#16814=CARTESIAN_POINT('Ctrl Pts',(7.60800746969262,19.7287195480601,0.));
#16815=CARTESIAN_POINT('Ctrl Pts',(7.60237814110187,19.7794022782484,0.));
#16816=CARTESIAN_POINT('Ctrl Pts',(7.59647587605448,19.830129556152,0.));
#16817=CARTESIAN_POINT('Ctrl Pts',(7.59030238888852,19.8808999994024,0.));
#16818=CARTESIAN_POINT('Ctrl Pts',(7.58385933533352,19.931712276832,0.));
#16819=CARTESIAN_POINT('Ctrl Pts',(7.57714827622806,19.9825651387294,0.));
#16820=CARTESIAN_POINT('Ctrl Pts',(7.57017066105973,20.0334574248557,0.));
#16821=CARTESIAN_POINT('Ctrl Pts',(7.5629278654946,20.0843880130978,0.));
#16822=CARTESIAN_POINT('Ctrl Pts',(7.55542122125495,20.1353557774357,0.));
#16823=CARTESIAN_POINT('Ctrl Pts',(7.54765204869254,20.1863595454674,0.));
#16824=CARTESIAN_POINT('Ctrl Pts',(7.53962169534167,20.2373980474879,0.));
#16825=CARTESIAN_POINT('Ctrl Pts',(7.53133155804008,20.2884698940944,0.));
#16826=CARTESIAN_POINT('Ctrl Pts',(7.52278303006887,20.3395736743243,0.));
#16827=CARTESIAN_POINT('Ctrl Pts',(7.51397746081994,20.3907080367098,0.));
#16828=CARTESIAN_POINT('Ctrl Pts',(7.50491611266253,20.4418717748497,0.));
#16829=CARTESIAN_POINT('Ctrl Pts',(7.49560012018406,20.4930639156161,0.));
#16830=CARTESIAN_POINT('Ctrl Pts',(7.48411651832413,20.5545277683621,0.));
#16831=CARTESIAN_POINT('Ctrl Pts',(7.47423073598682,20.6057817877246,0.));
#16832=CARTESIAN_POINT('Ctrl Pts',(7.46612041736314,20.6468066077586,0.));
#16833=CARTESIAN_POINT('Ctrl Pts',(7.45992433946824,20.6775873630604,0.));
#16834=CARTESIAN_POINT('Ctrl Pts',(7.45574324794401,20.698113262342,0.));
#16835=CARTESIAN_POINT('Ctrl Pts',(7.45007618140239,17.2541372868972,13.));
#16836=CARTESIAN_POINT('Ctrl Pts',(7.45637364573816,17.2687220121489,13.));
#16837=CARTESIAN_POINT('Ctrl Pts',(7.46226667103919,17.2834550499008,13.));
#16838=CARTESIAN_POINT('Ctrl Pts',(7.46778231425445,17.2983267669067,13.));
#16839=CARTESIAN_POINT('Ctrl Pts',(7.47424706065699,17.3157575315993,13.));
#16840=CARTESIAN_POINT('Ctrl Pts',(7.48019417753821,17.3333785326113,13.));
#16841=CARTESIAN_POINT('Ctrl Pts',(7.48573450280811,17.3511502187375,13.));
#16842=CARTESIAN_POINT('Ctrl Pts',(7.49353000563121,17.3761558316968,13.));
#16843=CARTESIAN_POINT('Ctrl Pts',(7.50052692940225,17.4014574303076,13.));
#16844=CARTESIAN_POINT('Ctrl Pts',(7.50711117101491,17.4269165094415,13.));
#16845=CARTESIAN_POINT('Ctrl Pts',(7.5114907300879,17.4438508122163,13.));
#16846=CARTESIAN_POINT('Ctrl Pts',(7.51568961154289,17.4608540901313,13.));
#16847=CARTESIAN_POINT('Ctrl Pts',(7.5197927693323,17.477895354957,13.));
#16848=CARTESIAN_POINT('Ctrl Pts',(7.5241120155096,17.4958340796498,13.));
#16849=CARTESIAN_POINT('Ctrl Pts',(7.52832602172349,17.5138146001176,13.));
#16850=CARTESIAN_POINT('Ctrl Pts',(7.53247314101595,17.5318219263294,13.));
#16851=CARTESIAN_POINT('Ctrl Pts',(7.53707874400533,17.5518200478164,13.));
#16852=CARTESIAN_POINT('Ctrl Pts',(7.54160061545783,17.5718516505933,13.));
#16853=CARTESIAN_POINT('Ctrl Pts',(7.54602601378991,17.5919190740375,13.));
#16854=CARTESIAN_POINT('Ctrl Pts',(7.55269751656652,17.6221716888714,13.));
#16855=CARTESIAN_POINT('Ctrl Pts',(7.55914375118896,17.652507694639,13.));
#16856=CARTESIAN_POINT('Ctrl Pts',(7.56521559976847,17.6829731243237,13.));
#16857=CARTESIAN_POINT('Ctrl Pts',(7.5696266650164,17.7051055929427,13.));
#16858=CARTESIAN_POINT('Ctrl Pts',(7.57383703867086,17.7273074810788,13.));
#16859=CARTESIAN_POINT('Ctrl Pts',(7.57782678310958,17.7495842480019,13.));
#16860=CARTESIAN_POINT('Ctrl Pts',(7.58270390405198,17.7768156880499,13.));
#16861=CARTESIAN_POINT('Ctrl Pts',(7.58725254420758,17.8041586050609,13.));
#16862=CARTESIAN_POINT('Ctrl Pts',(7.5915173324576,17.8315958505033,13.));
#16863=CARTESIAN_POINT('Ctrl Pts',(7.59612401157631,17.8612326292236,13.));
#16864=CARTESIAN_POINT('Ctrl Pts',(7.60040516926094,17.8909775513386,13.));
#16865=CARTESIAN_POINT('Ctrl Pts',(7.60444696777939,17.9207992272241,13.));
#16866=CARTESIAN_POINT('Ctrl Pts',(7.60817833718686,17.9483304583261,13.));
#16867=CARTESIAN_POINT('Ctrl Pts',(7.61170808544563,17.9759263070109,13.));
#16868=CARTESIAN_POINT('Ctrl Pts',(7.61506270604984,18.0035762489985,13.));
#16869=CARTESIAN_POINT('Ctrl Pts',(7.61962013038162,18.0411401148582,13.));
#16870=CARTESIAN_POINT('Ctrl Pts',(7.62385245909446,18.0788044381321,13.));
#16871=CARTESIAN_POINT('Ctrl Pts',(7.62773031180607,18.116575681107,13.));
#16872=CARTESIAN_POINT('Ctrl Pts',(7.63147235591991,18.1530241148041,13.));
#16873=CARTESIAN_POINT('Ctrl Pts',(7.63487692331691,18.1895746221268,13.));
#16874=CARTESIAN_POINT('Ctrl Pts',(7.6379279464237,18.2262298441586,13.));
#16875=CARTESIAN_POINT('Ctrl Pts',(7.6420728467974,18.2760269902896,13.));
#16876=CARTESIAN_POINT('Ctrl Pts',(7.64556831472686,18.3260163400101,13.));
#16877=CARTESIAN_POINT('Ctrl Pts',(7.64849356609469,18.3761647741644,13.));
#16878=CARTESIAN_POINT('Ctrl Pts',(7.6510647984552,18.4202441576132,13.));
#16879=CARTESIAN_POINT('Ctrl Pts',(7.65320196597345,18.4644442731511,13.));
#16880=CARTESIAN_POINT('Ctrl Pts',(7.65493429570875,18.5087513218552,13.));
#16881=CARTESIAN_POINT('Ctrl Pts',(7.65748817031438,18.5740706685303,13.));
#16882=CARTESIAN_POINT('Ctrl Pts',(7.65915358769477,18.6396252901549,13.));
#16883=CARTESIAN_POINT('Ctrl Pts',(7.65993127489918,18.705403439409,13.));
#16884=CARTESIAN_POINT('Ctrl Pts',(7.66091272374058,18.7884161056964,13.));
#16885=CARTESIAN_POINT('Ctrl Pts',(7.66048522719276,18.8717830757028,13.));
#16886=CARTESIAN_POINT('Ctrl Pts',(7.6587598380681,18.9554457129728,13.));
#16887=CARTESIAN_POINT('Ctrl Pts',(7.65642266547611,19.0687732053082,13.));
#16888=CARTESIAN_POINT('Ctrl Pts',(7.65169843823839,19.1826450749753,13.));
#16889=CARTESIAN_POINT('Ctrl Pts',(7.64469887385525,19.296975739756,13.));
#16890=CARTESIAN_POINT('Ctrl Pts',(7.63845857891208,19.3989045213524,13.));
#16891=CARTESIAN_POINT('Ctrl Pts',(7.63041784746716,19.5011952230932,13.));
#16892=CARTESIAN_POINT('Ctrl Pts',(7.62065725315594,19.6037897795266,13.));
#16893=CARTESIAN_POINT('Ctrl Pts',(7.60682380699052,19.7491944780556,13.));
#16894=CARTESIAN_POINT('Ctrl Pts',(7.58953015253691,19.8952104276061,13.));
#16895=CARTESIAN_POINT('Ctrl Pts',(7.56895177486366,20.041695755794,13.));
#16896=CARTESIAN_POINT('Ctrl Pts',(7.55296697986665,20.155482079397,13.));
#16897=CARTESIAN_POINT('Ctrl Pts',(7.53499708083853,20.2695554917631,13.));
#16898=CARTESIAN_POINT('Ctrl Pts',(7.51511029115765,20.3838501742203,13.));
#16899=CARTESIAN_POINT('Ctrl Pts',(7.49790671588851,20.482723708062,13.));
#16900=CARTESIAN_POINT('Ctrl Pts',(7.47927116735874,20.5817593865392,13.));
#16901=CARTESIAN_POINT('Ctrl Pts',(7.45922688154243,20.6809436222924,13.));
#16902=CARTESIAN_POINT('Ctrl Pts',(7.45807037082203,20.6866663321457,13.));
#16903=CARTESIAN_POINT('Ctrl Pts',(7.45690915953565,20.6923895455068,13.));
#16904=CARTESIAN_POINT('Ctrl Pts',(7.45574324794401,20.698113262342,13.));
#16905=CARTESIAN_POINT('Ctrl Pts',(12.3627494547115,18.1978687191668,0.));
#16906=CARTESIAN_POINT('Ctrl Pts',(12.3627494547115,18.1978687191668,21.));
#16907=CARTESIAN_POINT('Ctrl Pts',(12.3532177620787,18.1935275957711,0.));
#16908=CARTESIAN_POINT('Ctrl Pts',(12.3532177620787,18.1935275957711,21.));
#16909=CARTESIAN_POINT('Ctrl Pts',(12.3341713636489,18.1848265584754,0.));
#16910=CARTESIAN_POINT('Ctrl Pts',(12.3341713636489,18.1848265584754,21.));
#16911=CARTESIAN_POINT('Ctrl Pts',(12.3056527265146,18.1717186310224,0.));
#16912=CARTESIAN_POINT('Ctrl Pts',(12.3056527265146,18.1717186310224,21.));
#16913=CARTESIAN_POINT('Ctrl Pts',(12.2677298318549,18.1541286139166,0.));
#16914=CARTESIAN_POINT('Ctrl Pts',(12.2677298318549,18.1541286139166,21.));
#16915=CARTESIAN_POINT('Ctrl Pts',(12.2204964278426,18.1319528884305,0.));
#16916=CARTESIAN_POINT('Ctrl Pts',(12.2204964278426,18.1319528884305,21.));
#16917=CARTESIAN_POINT('Ctrl Pts',(12.1734337668195,18.109588624154,0.));
#16918=CARTESIAN_POINT('Ctrl Pts',(12.1734337668195,18.109588624154,21.));
#16919=CARTESIAN_POINT('Ctrl Pts',(12.1265426519718,18.0870354350128,0.));
#16920=CARTESIAN_POINT('Ctrl Pts',(12.1265426519718,18.0870354350128,21.));
#16921=CARTESIAN_POINT('Ctrl Pts',(12.0798241915081,18.0642929289333,0.));
#16922=CARTESIAN_POINT('Ctrl Pts',(12.0798241915081,18.0642929289333,21.));
#16923=CARTESIAN_POINT('Ctrl Pts',(12.0332798395991,18.0413607600052,0.));
#16924=CARTESIAN_POINT('Ctrl Pts',(12.0332798395991,18.0413607600052,21.));
#16925=CARTESIAN_POINT('Ctrl Pts',(11.986911314246,18.0182386160553,0.));
#16926=CARTESIAN_POINT('Ctrl Pts',(11.986911314246,18.0182386160553,21.));
#16927=CARTESIAN_POINT('Ctrl Pts',(11.9407205019619,17.9949261997754,0.));
#16928=CARTESIAN_POINT('Ctrl Pts',(11.9407205019619,17.9949261997754,21.));
#16929=CARTESIAN_POINT('Ctrl Pts',(11.8947093631895,17.9714232133203,0.));
#16930=CARTESIAN_POINT('Ctrl Pts',(11.8947093631895,17.9714232133203,21.));
#16931=CARTESIAN_POINT('Ctrl Pts',(11.8488798430201,17.9477293432951,0.));
#16932=CARTESIAN_POINT('Ctrl Pts',(11.8488798430201,17.9477293432951,21.));
#16933=CARTESIAN_POINT('Ctrl Pts',(11.8032337607271,17.9238442458356,0.));
#16934=CARTESIAN_POINT('Ctrl Pts',(11.8032337607271,17.9238442458356,21.));
#16935=CARTESIAN_POINT('Ctrl Pts',(11.7577728408871,17.8997675418752,0.));
#16936=CARTESIAN_POINT('Ctrl Pts',(11.7577728408871,17.8997675418752,21.));
#16937=CARTESIAN_POINT('Ctrl Pts',(11.7124987772363,17.8754988158862,0.));
#16938=CARTESIAN_POINT('Ctrl Pts',(11.7124987772363,17.8754988158862,21.));
#16939=CARTESIAN_POINT('Ctrl Pts',(11.6674132861792,17.8510376144926,0.));
#16940=CARTESIAN_POINT('Ctrl Pts',(11.6674132861792,17.8510376144926,21.));
#16941=CARTESIAN_POINT('Ctrl Pts',(11.6225181583564,17.8263834470057,0.));
#16942=CARTESIAN_POINT('Ctrl Pts',(11.6225181583564,17.8263834470057,21.));
#16943=CARTESIAN_POINT('Ctrl Pts',(11.5778153222435,17.8015357852426,0.));
#16944=CARTESIAN_POINT('Ctrl Pts',(11.5778153222435,17.8015357852426,21.));
#16945=CARTESIAN_POINT('Ctrl Pts',(11.5333068279911,17.7764940721306,0.));
#16946=CARTESIAN_POINT('Ctrl Pts',(11.5333068279911,17.7764940721306,21.));
#16947=CARTESIAN_POINT('Ctrl Pts',(11.4889948016216,17.7512577332768,0.));
#16948=CARTESIAN_POINT('Ctrl Pts',(11.4889948016216,17.7512577332768,21.));
#16949=CARTESIAN_POINT('Ctrl Pts',(11.4448814046804,17.725826190457,0.));
#16950=CARTESIAN_POINT('Ctrl Pts',(11.4448814046804,17.725826190457,21.));
#16951=CARTESIAN_POINT('Ctrl Pts',(11.4009687970126,17.700198872213,0.));
#16952=CARTESIAN_POINT('Ctrl Pts',(11.4009687970126,17.700198872213,21.));
#16953=CARTESIAN_POINT('Ctrl Pts',(11.3572590796967,17.674375235974,0.));
#16954=CARTESIAN_POINT('Ctrl Pts',(11.3572590796967,17.674375235974,21.));
#16955=CARTESIAN_POINT('Ctrl Pts',(11.3137543310722,17.6483547422688,0.));
#16956=CARTESIAN_POINT('Ctrl Pts',(11.3137543310722,17.6483547422688,21.));
#16957=CARTESIAN_POINT('Ctrl Pts',(11.2704566868205,17.6221368072528,0.));
#16958=CARTESIAN_POINT('Ctrl Pts',(11.2704566868205,17.6221368072528,21.));
#16959=CARTESIAN_POINT('Ctrl Pts',(11.2273684103051,17.5957207597803,0.));
#16960=CARTESIAN_POINT('Ctrl Pts',(11.2273684103051,17.5957207597803,21.));
#16961=CARTESIAN_POINT('Ctrl Pts',(11.1844919535058,17.5691058058227,0.));
#16962=CARTESIAN_POINT('Ctrl Pts',(11.1844919535058,17.5691058058227,21.));
#16963=CARTESIAN_POINT('Ctrl Pts',(11.1418300507683,17.5422909714139,0.));
#16964=CARTESIAN_POINT('Ctrl Pts',(11.1418300507683,17.5422909714139,21.));
#16965=CARTESIAN_POINT('Ctrl Pts',(11.0993856581394,17.5152751467292,0.));
#16966=CARTESIAN_POINT('Ctrl Pts',(11.0993856581394,17.5152751467292,21.));
#16967=CARTESIAN_POINT('Ctrl Pts',(11.0571618040371,17.4880571878157,0.));
#16968=CARTESIAN_POINT('Ctrl Pts',(11.0571618040371,17.4880571878157,21.));
#16969=CARTESIAN_POINT('Ctrl Pts',(11.0151614525642,17.460636011184,0.));
#16970=CARTESIAN_POINT('Ctrl Pts',(11.0151614525642,17.460636011184,21.));
#16971=CARTESIAN_POINT('Ctrl Pts',(10.9733873885115,17.4330106728622,0.));
#16972=CARTESIAN_POINT('Ctrl Pts',(10.9733873885115,17.4330106728622,21.));
#16973=CARTESIAN_POINT('Ctrl Pts',(10.9318420203801,17.4051805054129,0.));
#16974=CARTESIAN_POINT('Ctrl Pts',(10.9318420203801,17.4051805054129,21.));
#16975=CARTESIAN_POINT('Ctrl Pts',(10.8905275295837,17.377145012528,0.));
#16976=CARTESIAN_POINT('Ctrl Pts',(10.8905275295837,17.377145012528,21.));
#16977=CARTESIAN_POINT('Ctrl Pts',(10.8494462423128,17.3489036079991,0.));
#16978=CARTESIAN_POINT('Ctrl Pts',(10.8494462423128,17.3489036079991,21.));
#16979=CARTESIAN_POINT('Ctrl Pts',(10.8086009632423,17.3204553814537,0.));
#16980=CARTESIAN_POINT('Ctrl Pts',(10.8086009632423,17.3204553814537,21.));
#16981=CARTESIAN_POINT('Ctrl Pts',(10.7679952591482,17.2917988998581,0.));
#16982=CARTESIAN_POINT('Ctrl Pts',(10.7679952591482,17.2917988998581,21.));
#16983=CARTESIAN_POINT('Ctrl Pts',(10.7276339231608,17.2629318816279,0.));
#16984=CARTESIAN_POINT('Ctrl Pts',(10.7276339231608,17.2629318816279,21.));
#16985=CARTESIAN_POINT('Ctrl Pts',(10.6875226650217,17.2338514174708,0.));
#16986=CARTESIAN_POINT('Ctrl Pts',(10.6875226650217,17.2338514174708,21.));
#16987=CARTESIAN_POINT('Ctrl Pts',(10.6476672831754,17.2045545572011,0.));
#16988=CARTESIAN_POINT('Ctrl Pts',(10.6476672831754,17.2045545572011,21.));
#16989=CARTESIAN_POINT('Ctrl Pts',(10.6080729180997,17.1750388395657,0.));
#16990=CARTESIAN_POINT('Ctrl Pts',(10.6080729180997,17.1750388395657,21.));
#16991=CARTESIAN_POINT('Ctrl Pts',(10.5687434234512,17.1453027387554,0.));
#16992=CARTESIAN_POINT('Ctrl Pts',(10.5687434234512,17.1453027387554,21.));
#16993=CARTESIAN_POINT('Ctrl Pts',(10.5296803023445,17.1153464189932,0.));
#16994=CARTESIAN_POINT('Ctrl Pts',(10.5296803023445,17.1153464189932,21.));
#16995=CARTESIAN_POINT('Ctrl Pts',(10.4908835057575,17.0851711712016,0.));
#16996=CARTESIAN_POINT('Ctrl Pts',(10.4908835057575,17.0851711712016,21.));
#16997=CARTESIAN_POINT('Ctrl Pts',(10.452353435089,17.0547779975888,0.));
#16998=CARTESIAN_POINT('Ctrl Pts',(10.452353435089,17.0547779975888,21.));
#16999=CARTESIAN_POINT('Ctrl Pts',(10.4140927470882,17.0241663361802,0.));
#17000=CARTESIAN_POINT('Ctrl Pts',(10.4140927470882,17.0241663361802,21.));
#17001=CARTESIAN_POINT('Ctrl Pts',(10.3761078860454,16.9933329788855,0.));
#17002=CARTESIAN_POINT('Ctrl Pts',(10.3761078860454,16.9933329788855,21.));
#17003=CARTESIAN_POINT('Ctrl Pts',(10.3384116178624,16.9622702798438,0.));
#17004=CARTESIAN_POINT('Ctrl Pts',(10.3384116178624,16.9622702798438,21.));
#17005=CARTESIAN_POINT('Ctrl Pts',(10.3010210756062,16.9309675442426,0.));
#17006=CARTESIAN_POINT('Ctrl Pts',(10.3010210756062,16.9309675442426,21.));
#17007=CARTESIAN_POINT('Ctrl Pts',(10.2639532144219,16.8994142530447,0.));
#17008=CARTESIAN_POINT('Ctrl Pts',(10.2639532144219,16.8994142530447,21.));
#17009=CARTESIAN_POINT('Ctrl Pts',(10.2272206796636,16.8676029947679,0.));
#17010=CARTESIAN_POINT('Ctrl Pts',(10.2272206796636,16.8676029947679,21.));
#17011=CARTESIAN_POINT('Ctrl Pts',(10.1908283166713,16.8355319435838,0.));
#17012=CARTESIAN_POINT('Ctrl Pts',(10.1908283166713,16.8355319435838,21.));
#17013=CARTESIAN_POINT('Ctrl Pts',(10.1547673397274,16.8032089941901,0.));
#17014=CARTESIAN_POINT('Ctrl Pts',(10.1547673397274,16.8032089941901,21.));
#17015=CARTESIAN_POINT('Ctrl Pts',(10.1190207721353,16.7706479198888,0.));
#17016=CARTESIAN_POINT('Ctrl Pts',(10.1190207721353,16.7706479198888,21.));
#17017=CARTESIAN_POINT('Ctrl Pts',(10.0835742491038,16.7378607357337,0.));
#17018=CARTESIAN_POINT('Ctrl Pts',(10.0835742491038,16.7378607357337,21.));
#17019=CARTESIAN_POINT('Ctrl Pts',(10.0484259314257,16.7048506904207,0.));
#17020=CARTESIAN_POINT('Ctrl Pts',(10.0484259314257,16.7048506904207,21.));
#17021=CARTESIAN_POINT('Ctrl Pts',(10.0135950379525,16.6716062376277,0.));
#17022=CARTESIAN_POINT('Ctrl Pts',(10.0135950379525,16.6716062376277,21.));
#17023=CARTESIAN_POINT('Ctrl Pts',(9.97913546489641,16.6380914029057,0.));
#17024=CARTESIAN_POINT('Ctrl Pts',(9.97913546489641,16.6380914029057,21.));
#17025=CARTESIAN_POINT('Ctrl Pts',(9.9451214271291,16.6042559779574,0.));
#17026=CARTESIAN_POINT('Ctrl Pts',(9.9451214271291,16.6042559779574,21.));
#17027=CARTESIAN_POINT('Ctrl Pts',(9.91162317616649,16.5700527532381,0.));
#17028=CARTESIAN_POINT('Ctrl Pts',(9.91162317616649,16.5700527532381,21.));
#17029=CARTESIAN_POINT('Ctrl Pts',(9.8786843754698,16.5354535643506,0.));
#17030=CARTESIAN_POINT('Ctrl Pts',(9.8786843754698,16.5354535643506,21.));
#17031=CARTESIAN_POINT('Ctrl Pts',(9.84630229363521,16.5004633692332,0.));
#17032=CARTESIAN_POINT('Ctrl Pts',(9.84630229363521,16.5004633692332,21.));
#17033=CARTESIAN_POINT('Ctrl Pts',(9.81439757053278,16.4651416449558,0.));
#17034=CARTESIAN_POINT('Ctrl Pts',(9.81439757053278,16.4651416449558,21.));
#17035=CARTESIAN_POINT('Ctrl Pts',(9.78285689698057,16.4295725710378,0.));
#17036=CARTESIAN_POINT('Ctrl Pts',(9.78285689698057,16.4295725710378,21.));
#17037=CARTESIAN_POINT('Ctrl Pts',(9.75159288382684,16.3938231282759,0.));
#17038=CARTESIAN_POINT('Ctrl Pts',(9.75159288382684,16.3938231282759,21.));
#17039=CARTESIAN_POINT('Ctrl Pts',(9.72060002001011,16.3579039682519,0.));
#17040=CARTESIAN_POINT('Ctrl Pts',(9.72060002001011,16.3579039682519,21.));
#17041=CARTESIAN_POINT('Ctrl Pts',(9.69000797146315,16.3217321000366,0.));
#17042=CARTESIAN_POINT('Ctrl Pts',(9.69000797146315,16.3217321000366,21.));
#17043=CARTESIAN_POINT('Ctrl Pts',(9.66014786078746,16.2850845948324,0.));
#17044=CARTESIAN_POINT('Ctrl Pts',(9.66014786078746,16.2850845948324,21.));
#17045=CARTESIAN_POINT('Ctrl Pts',(9.63146315443273,16.2476599387841,0.));
#17046=CARTESIAN_POINT('Ctrl Pts',(9.63146315443273,16.2476599387841,21.));
#17047=CARTESIAN_POINT('Ctrl Pts',(9.60981421781524,16.2168537871666,0.));
#17048=CARTESIAN_POINT('Ctrl Pts',(9.60981421781524,16.2168537871666,21.));
#17049=CARTESIAN_POINT('Ctrl Pts',(9.59446643316596,16.1931534965272,0.));
#17050=CARTESIAN_POINT('Ctrl Pts',(9.59446643316596,16.1931534965272,21.));
#17051=CARTESIAN_POINT('Ctrl Pts',(9.58464985151482,16.1770747160769,0.));
#17052=CARTESIAN_POINT('Ctrl Pts',(9.58464985151482,16.1770747160769,21.));
#17053=CARTESIAN_POINT('Ctrl Pts',(9.57984538049455,16.1689656784104,0.));
#17054=CARTESIAN_POINT('Ctrl Pts',(9.57984538049455,16.1689656784104,21.));
#17055=CARTESIAN_POINT('',(12.3627494547114,18.1978687191669,0.));
#17056=CARTESIAN_POINT('Ctrl Pts',(9.57984538049455,16.1689656784104,0.));
#17057=CARTESIAN_POINT('Ctrl Pts',(9.58464985151482,16.1770747160769,0.));
#17058=CARTESIAN_POINT('Ctrl Pts',(9.59446643316596,16.1931534965272,0.));
#17059=CARTESIAN_POINT('Ctrl Pts',(9.60981421781524,16.2168537871666,0.));
#17060=CARTESIAN_POINT('Ctrl Pts',(9.63146315443273,16.2476599387841,0.));
#17061=CARTESIAN_POINT('Ctrl Pts',(9.66014786078746,16.2850845948324,0.));
#17062=CARTESIAN_POINT('Ctrl Pts',(9.69000797146315,16.3217321000366,0.));
#17063=CARTESIAN_POINT('Ctrl Pts',(9.72060002001011,16.3579039682519,0.));
#17064=CARTESIAN_POINT('Ctrl Pts',(9.75159288382684,16.3938231282759,0.));
#17065=CARTESIAN_POINT('Ctrl Pts',(9.78285689698057,16.4295725710378,0.));
#17066=CARTESIAN_POINT('Ctrl Pts',(9.81439757053278,16.4651416449558,0.));
#17067=CARTESIAN_POINT('Ctrl Pts',(9.84630229363521,16.5004633692332,0.));
#17068=CARTESIAN_POINT('Ctrl Pts',(9.8786843754698,16.5354535643506,0.));
#17069=CARTESIAN_POINT('Ctrl Pts',(9.91162317616649,16.5700527532381,0.));
#17070=CARTESIAN_POINT('Ctrl Pts',(9.9451214271291,16.6042559779574,0.));
#17071=CARTESIAN_POINT('Ctrl Pts',(9.97913546489641,16.6380914029057,0.));
#17072=CARTESIAN_POINT('Ctrl Pts',(10.0135950379525,16.6716062376277,0.));
#17073=CARTESIAN_POINT('Ctrl Pts',(10.0484259314257,16.7048506904207,0.));
#17074=CARTESIAN_POINT('Ctrl Pts',(10.0835742491038,16.7378607357337,0.));
#17075=CARTESIAN_POINT('Ctrl Pts',(10.1190207721353,16.7706479198888,0.));
#17076=CARTESIAN_POINT('Ctrl Pts',(10.1547673397274,16.8032089941901,0.));
#17077=CARTESIAN_POINT('Ctrl Pts',(10.1908283166713,16.8355319435838,0.));
#17078=CARTESIAN_POINT('Ctrl Pts',(10.2272206796636,16.8676029947679,0.));
#17079=CARTESIAN_POINT('Ctrl Pts',(10.2639532144219,16.8994142530447,0.));
#17080=CARTESIAN_POINT('Ctrl Pts',(10.3010210756062,16.9309675442426,0.));
#17081=CARTESIAN_POINT('Ctrl Pts',(10.3384116178624,16.9622702798438,0.));
#17082=CARTESIAN_POINT('Ctrl Pts',(10.3761078860454,16.9933329788855,0.));
#17083=CARTESIAN_POINT('Ctrl Pts',(10.4140927470882,17.0241663361802,0.));
#17084=CARTESIAN_POINT('Ctrl Pts',(10.452353435089,17.0547779975888,0.));
#17085=CARTESIAN_POINT('Ctrl Pts',(10.4908835057575,17.0851711712016,0.));
#17086=CARTESIAN_POINT('Ctrl Pts',(10.5296803023445,17.1153464189932,0.));
#17087=CARTESIAN_POINT('Ctrl Pts',(10.5687434234512,17.1453027387554,0.));
#17088=CARTESIAN_POINT('Ctrl Pts',(10.6080729180997,17.1750388395657,0.));
#17089=CARTESIAN_POINT('Ctrl Pts',(10.6476672831754,17.2045545572011,0.));
#17090=CARTESIAN_POINT('Ctrl Pts',(10.6875226650217,17.2338514174708,0.));
#17091=CARTESIAN_POINT('Ctrl Pts',(10.7276339231608,17.2629318816279,0.));
#17092=CARTESIAN_POINT('Ctrl Pts',(10.7679952591482,17.2917988998581,0.));
#17093=CARTESIAN_POINT('Ctrl Pts',(10.8086009632423,17.3204553814537,0.));
#17094=CARTESIAN_POINT('Ctrl Pts',(10.8494462423128,17.3489036079991,0.));
#17095=CARTESIAN_POINT('Ctrl Pts',(10.8905275295837,17.377145012528,0.));
#17096=CARTESIAN_POINT('Ctrl Pts',(10.9318420203801,17.4051805054129,0.));
#17097=CARTESIAN_POINT('Ctrl Pts',(10.9733873885115,17.4330106728622,0.));
#17098=CARTESIAN_POINT('Ctrl Pts',(11.0151614525642,17.460636011184,0.));
#17099=CARTESIAN_POINT('Ctrl Pts',(11.0571618040371,17.4880571878157,0.));
#17100=CARTESIAN_POINT('Ctrl Pts',(11.0993856581394,17.5152751467292,0.));
#17101=CARTESIAN_POINT('Ctrl Pts',(11.1418300507683,17.5422909714139,0.));
#17102=CARTESIAN_POINT('Ctrl Pts',(11.1844919535058,17.5691058058227,0.));
#17103=CARTESIAN_POINT('Ctrl Pts',(11.2273684103051,17.5957207597803,0.));
#17104=CARTESIAN_POINT('Ctrl Pts',(11.2704566868205,17.6221368072528,0.));
#17105=CARTESIAN_POINT('Ctrl Pts',(11.3137543310722,17.6483547422688,0.));
#17106=CARTESIAN_POINT('Ctrl Pts',(11.3572590796967,17.674375235974,0.));
#17107=CARTESIAN_POINT('Ctrl Pts',(11.4009687970126,17.700198872213,0.));
#17108=CARTESIAN_POINT('Ctrl Pts',(11.4448814046804,17.725826190457,0.));
#17109=CARTESIAN_POINT('Ctrl Pts',(11.4889948016216,17.7512577332768,0.));
#17110=CARTESIAN_POINT('Ctrl Pts',(11.5333068279911,17.7764940721306,0.));
#17111=CARTESIAN_POINT('Ctrl Pts',(11.5778153222435,17.8015357852426,0.));
#17112=CARTESIAN_POINT('Ctrl Pts',(11.6225181583564,17.8263834470057,0.));
#17113=CARTESIAN_POINT('Ctrl Pts',(11.6674132861792,17.8510376144926,0.));
#17114=CARTESIAN_POINT('Ctrl Pts',(11.7124987772363,17.8754988158862,0.));
#17115=CARTESIAN_POINT('Ctrl Pts',(11.7577728408871,17.8997675418752,0.));
#17116=CARTESIAN_POINT('Ctrl Pts',(11.8032337607271,17.9238442458356,0.));
#17117=CARTESIAN_POINT('Ctrl Pts',(11.8488798430201,17.9477293432951,0.));
#17118=CARTESIAN_POINT('Ctrl Pts',(11.8947093631895,17.9714232133203,0.));
#17119=CARTESIAN_POINT('Ctrl Pts',(11.9407205019619,17.9949261997754,0.));
#17120=CARTESIAN_POINT('Ctrl Pts',(11.986911314246,18.0182386160553,0.));
#17121=CARTESIAN_POINT('Ctrl Pts',(12.0332798395991,18.0413607600052,0.));
#17122=CARTESIAN_POINT('Ctrl Pts',(12.0798241915081,18.0642929289333,0.));
#17123=CARTESIAN_POINT('Ctrl Pts',(12.1265426519718,18.0870354350128,0.));
#17124=CARTESIAN_POINT('Ctrl Pts',(12.1734337668195,18.109588624154,0.));
#17125=CARTESIAN_POINT('Ctrl Pts',(12.2299089600472,18.1364257412858,0.));
#17126=CARTESIAN_POINT('Ctrl Pts',(12.2771850498068,18.1585543320743,0.));
#17127=CARTESIAN_POINT('Ctrl Pts',(12.3151419520839,18.1761067306718,0.));
#17128=CARTESIAN_POINT('Ctrl Pts',(12.3436860694314,18.1891864723772,0.));
#17129=CARTESIAN_POINT('Ctrl Pts',(12.3627494547115,18.1978687191668,0.));
#17130=CARTESIAN_POINT('',(12.3627494547114,18.1978687191669,13.));
#17131=CARTESIAN_POINT('Ctrl Pts',(12.3627494547115,18.1978687191668,13.));
#17132=CARTESIAN_POINT('Ctrl Pts',(12.2657596014803,18.1536955657482,13.));
#17133=CARTESIAN_POINT('Ctrl Pts',(12.169023050136,18.1079923296861,13.));
#17134=CARTESIAN_POINT('Ctrl Pts',(12.0727475247274,18.0607552358515,13.));
#17135=CARTESIAN_POINT('Ctrl Pts',(11.9463830806602,17.9987551680626,13.));
#17136=CARTESIAN_POINT('Ctrl Pts',(11.8208236442934,17.9341116361939,13.));
#17137=CARTESIAN_POINT('Ctrl Pts',(11.6966194524201,17.8668433674001,13.));
#17138=CARTESIAN_POINT('Ctrl Pts',(11.5669851023492,17.7966341564713,13.));
#17139=CARTESIAN_POINT('Ctrl Pts',(11.4388217697851,17.7235639107164,13.));
#17140=CARTESIAN_POINT('Ctrl Pts',(11.3127555917358,17.6476730730182,13.));
#17141=CARTESIAN_POINT('Ctrl Pts',(11.1945685498145,17.5765254126762,13.));
#17142=CARTESIAN_POINT('Ctrl Pts',(11.0782188859152,17.5029025452135,13.));
#17143=CARTESIAN_POINT('Ctrl Pts',(10.9642554050871,17.4268346378942,13.));
#17144=CARTESIAN_POINT('Ctrl Pts',(10.9600254617552,17.4240112515339,13.));
#17145=CARTESIAN_POINT('Ctrl Pts',(10.9557986898388,17.4211844233848,13.));
#17146=CARTESIAN_POINT('Ctrl Pts',(10.9515873193929,17.4183623684055,13.));
#17147=CARTESIAN_POINT('Ctrl Pts',(10.8848661681826,17.3736522771363,13.));
#17148=CARTESIAN_POINT('Ctrl Pts',(10.821246862648,17.3296352982567,13.));
#17149=CARTESIAN_POINT('Ctrl Pts',(10.7606710931032,17.2864928503383,13.));
#17150=CARTESIAN_POINT('Ctrl Pts',(10.7071165337234,17.2483509529062,13.));
#17151=CARTESIAN_POINT('Ctrl Pts',(10.6559465493499,17.2108884656131,13.));
#17152=CARTESIAN_POINT('Ctrl Pts',(10.6071256521871,17.1742227594056,13.));
#17153=CARTESIAN_POINT('Ctrl Pts',(10.5586309624272,17.1378020430589,13.));
#17154=CARTESIAN_POINT('Ctrl Pts',(10.5124511278601,17.1021695681408,13.));
#17155=CARTESIAN_POINT('Ctrl Pts',(10.4685087734972,17.0674664166947,13.));
#17156=CARTESIAN_POINT('Ctrl Pts',(10.4297467459301,17.0368543902677,13.));
#17157=CARTESIAN_POINT('Ctrl Pts',(10.3927227952995,17.0069675134053,13.));
#17158=CARTESIAN_POINT('Ctrl Pts',(10.3574204589883,16.9778741242538,13.));
#17159=CARTESIAN_POINT('Ctrl Pts',(10.3251177699006,16.9512528067301,13.));
#17160=CARTESIAN_POINT('Ctrl Pts',(10.294261944748,16.9252920099693,13.));
#17161=CARTESIAN_POINT('Ctrl Pts',(10.2648422441037,16.900041094165,13.));
#17162=CARTESIAN_POINT('Ctrl Pts',(10.2348002062189,16.8742560265875,13.));
#17163=CARTESIAN_POINT('Ctrl Pts',(10.2062569586814,16.849210296515,13.));
#17164=CARTESIAN_POINT('Ctrl Pts',(10.1791517798772,16.8249897307869,13.));
#17165=CARTESIAN_POINT('Ctrl Pts',(10.1529843049216,16.8016070756981,13.));
#17166=CARTESIAN_POINT('Ctrl Pts',(10.1281515192515,16.778997431011,13.));
#17167=CARTESIAN_POINT('Ctrl Pts',(10.104594858302,16.7572394204805,13.));
#17168=CARTESIAN_POINT('Ctrl Pts',(10.0816981615767,16.736090983122,13.));
#17169=CARTESIAN_POINT('Ctrl Pts',(10.0600064453471,16.7157475741055,13.));
#17170=CARTESIAN_POINT('Ctrl Pts',(10.0395060154369,16.6962518487154,13.));
#17171=CARTESIAN_POINT('Ctrl Pts',(10.0146112621281,16.6725771610972,13.));
#17172=CARTESIAN_POINT('Ctrl Pts',(9.99147913670146,16.6501483869943,13.));
#17173=CARTESIAN_POINT('Ctrl Pts',(9.97012646745884,16.6290105279122,13.));
#17174=CARTESIAN_POINT('Ctrl Pts',(9.95071237566143,16.6097917439767,13.));
#17175=CARTESIAN_POINT('Ctrl Pts',(9.93277105321012,16.5916388348028,13.));
#17176=CARTESIAN_POINT('Ctrl Pts',(9.91627156066964,16.5746150219053,13.));
#17177=CARTESIAN_POINT('Ctrl Pts',(9.89217566126396,16.5497534037634,13.));
#17178=CARTESIAN_POINT('Ctrl Pts',(9.87115249083465,16.5273017471855,13.));
#17179=CARTESIAN_POINT('Ctrl Pts',(9.85298457624544,16.5075382670064,13.));
#17180=CARTESIAN_POINT('Ctrl Pts',(9.8397201346617,16.4931088988453,13.));
#17181=CARTESIAN_POINT('Ctrl Pts',(9.82797372144175,16.4801151434696,13.));
#17182=CARTESIAN_POINT('Ctrl Pts',(9.81768546292149,16.4686464995442,13.));
#17183=CARTESIAN_POINT('Ctrl Pts',(9.81140156894346,16.4616416461614,13.));
#17184=CARTESIAN_POINT('Ctrl Pts',(9.80566257035652,16.4552050742887,13.));
#17185=CARTESIAN_POINT('Ctrl Pts',(9.80046232294511,16.4493517473189,13.));
#17186=CARTESIAN_POINT('Ctrl Pts',(9.79879887487039,16.4474793930427,13.));
#17187=CARTESIAN_POINT('Ctrl Pts',(9.79719059001671,16.4456666910777,13.));
#17188=CARTESIAN_POINT('Ctrl Pts',(9.79563736221273,16.4439140626976,13.));
#17189=CARTESIAN_POINT('Ctrl Pts',(9.79500566407819,16.4432012682991,13.));
#17190=CARTESIAN_POINT('Ctrl Pts',(9.79438446351028,16.4424999805057,13.));
#17191=CARTESIAN_POINT('Ctrl Pts',(9.79376929391731,16.4418051873884,13.));
#17192=CARTESIAN_POINT('Ctrl Pts',(9.77984315351516,16.4260765385531,13.));
#17193=CARTESIAN_POINT('Ctrl Pts',(9.76683512585064,16.4112295751864,13.));
#17194=CARTESIAN_POINT('Ctrl Pts',(9.75465239268516,16.3972210812639,13.));
#17195=CARTESIAN_POINT('Ctrl Pts',(9.73997218062171,16.3803408247009,13.));
#17196=CARTESIAN_POINT('Ctrl Pts',(9.72649172856169,16.3646770770088,13.));
#17197=CARTESIAN_POINT('Ctrl Pts',(9.71411692998175,16.3501049923794,13.));
#17198=CARTESIAN_POINT('Ctrl Pts',(9.70072429268956,16.334334340213,13.));
#17199=CARTESIAN_POINT('Ctrl Pts',(9.68863308112708,16.3198378092419,13.));
#17200=CARTESIAN_POINT('Ctrl Pts',(9.67773230410014,16.3064499392455,13.));
#17201=CARTESIAN_POINT('Ctrl Pts',(9.66640622721792,16.2925397340835,13.));
#17202=CARTESIAN_POINT('Ctrl Pts',(9.65636576393748,16.279825988344,13.));
#17203=CARTESIAN_POINT('Ctrl Pts',(9.64743434299806,16.2681588091213,13.));
#17204=CARTESIAN_POINT('Ctrl Pts',(9.63114001841937,16.2468734160732,13.));
#17205=CARTESIAN_POINT('Ctrl Pts',(9.61852759006646,16.2290773159714,13.));
#17206=CARTESIAN_POINT('Ctrl Pts',(9.60835104757439,16.2139851574147,13.));
#17207=CARTESIAN_POINT('Ctrl Pts',(9.60185659561648,16.2043536643252,13.));
#17208=CARTESIAN_POINT('Ctrl Pts',(9.59635317286195,16.1958243014909,13.));
#17209=CARTESIAN_POINT('Ctrl Pts',(9.59155330605552,16.1881695092273,13.));
#17210=CARTESIAN_POINT('Ctrl Pts',(9.58711261470323,16.1810875273349,13.));
#17211=CARTESIAN_POINT('Ctrl Pts',(9.58327471391801,16.1747537441068,13.));
#17212=CARTESIAN_POINT('Ctrl Pts',(9.57984538049455,16.1689656784104,13.));
#17213=CARTESIAN_POINT('',(12.3627494547114,18.1978687191669,0.));
#17214=CARTESIAN_POINT('Origin',(3.33073116609659E-12,4.58435815896522E-12,
0.));
#17215=CARTESIAN_POINT('',(13.4869019493419,17.3811241238545,0.));
#17216=CARTESIAN_POINT('Origin',(3.33073116609659E-12,4.58435815896522E-12,
0.));
#17217=CARTESIAN_POINT('',(13.4869019493419,17.3811241238545,13.));
#17218=CARTESIAN_POINT('Origin',(3.33073116609659E-12,4.58435815896522E-12,
13.));
#17219=CARTESIAN_POINT('',(13.4869019493419,17.3811241238545,0.));
#17220=CARTESIAN_POINT('Ctrl Pts',(12.4172651441477,14.1074595503134,0.));
#17221=CARTESIAN_POINT('Ctrl Pts',(12.4172651441477,14.1074595503134,21.));
#17222=CARTESIAN_POINT('Ctrl Pts',(12.4234926340671,14.1145347042316,0.));
#17223=CARTESIAN_POINT('Ctrl Pts',(12.4234926340671,14.1145347042316,21.));
#17224=CARTESIAN_POINT('Ctrl Pts',(12.4357509724316,14.1288394445866,0.));
#17225=CARTESIAN_POINT('Ctrl Pts',(12.4357509724316,14.1288394445866,21.));
#17226=CARTESIAN_POINT('Ctrl Pts',(12.4535485619996,14.1507598477672,0.));
#17227=CARTESIAN_POINT('Ctrl Pts',(12.4535485619996,14.1507598477672,21.));
#17228=CARTESIAN_POINT('Ctrl Pts',(12.4761570639125,14.1808688343892,0.));
#17229=CARTESIAN_POINT('Ctrl Pts',(12.4761570639125,14.1808688343892,21.));
#17230=CARTESIAN_POINT('Ctrl Pts',(12.5028859651751,14.2197144660135,0.));
#17231=CARTESIAN_POINT('Ctrl Pts',(12.5028859651751,14.2197144660135,21.));
#17232=CARTESIAN_POINT('Ctrl Pts',(12.5285125321527,14.2594378207584,0.));
#17233=CARTESIAN_POINT('Ctrl Pts',(12.5285125321527,14.2594378207584,21.));
#17234=CARTESIAN_POINT('Ctrl Pts',(12.5534605602317,14.2997103098726,0.));
#17235=CARTESIAN_POINT('Ctrl Pts',(12.5534605602317,14.2997103098726,21.));
#17236=CARTESIAN_POINT('Ctrl Pts',(12.5780443898087,14.3402859058353,0.));
#17237=CARTESIAN_POINT('Ctrl Pts',(12.5780443898087,14.3402859058353,21.));
#17238=CARTESIAN_POINT('Ctrl Pts',(12.6023830189244,14.3810669346235,0.));
#17239=CARTESIAN_POINT('Ctrl Pts',(12.6023830189244,14.3810669346235,21.));
#17240=CARTESIAN_POINT('Ctrl Pts',(12.626464614311,14.4220553460485,0.));
#17241=CARTESIAN_POINT('Ctrl Pts',(12.626464614311,14.4220553460485,21.));
#17242=CARTESIAN_POINT('Ctrl Pts',(12.6501984687124,14.463313553928,0.));
#17243=CARTESIAN_POINT('Ctrl Pts',(12.6501984687124,14.463313553928,21.));
#17244=CARTESIAN_POINT('Ctrl Pts',(12.6734695081852,14.5049233087958,0.));
#17245=CARTESIAN_POINT('Ctrl Pts',(12.6734695081852,14.5049233087958,21.));
#17246=CARTESIAN_POINT('Ctrl Pts',(12.6961966430455,14.5469417071951,0.));
#17247=CARTESIAN_POINT('Ctrl Pts',(12.6961966430455,14.5469417071951,21.));
#17248=CARTESIAN_POINT('Ctrl Pts',(12.7183743139638,14.5893698147583,0.));
#17249=CARTESIAN_POINT('Ctrl Pts',(12.7183743139638,14.5893698147583,21.));
#17250=CARTESIAN_POINT('Ctrl Pts',(12.7400427996251,14.6321748083434,0.));
#17251=CARTESIAN_POINT('Ctrl Pts',(12.7400427996251,14.6321748083434,21.));
#17252=CARTESIAN_POINT('Ctrl Pts',(12.7612687078867,14.6753044633399,0.));
#17253=CARTESIAN_POINT('Ctrl Pts',(12.7612687078867,14.6753044633399,21.));
#17254=CARTESIAN_POINT('Ctrl Pts',(12.7821227233337,14.7187037124277,0.));
#17255=CARTESIAN_POINT('Ctrl Pts',(12.7821227233337,14.7187037124277,21.));
#17256=CARTESIAN_POINT('Ctrl Pts',(12.8026557145457,14.7623324139791,0.));
#17257=CARTESIAN_POINT('Ctrl Pts',(12.8026557145457,14.7623324139791,21.));
#17258=CARTESIAN_POINT('Ctrl Pts',(12.8228846016791,14.8061758577898,0.));
#17259=CARTESIAN_POINT('Ctrl Pts',(12.8228846016791,14.8061758577898,21.));
#17260=CARTESIAN_POINT('Ctrl Pts',(12.8428057266944,14.8502347891476,0.));
#17261=CARTESIAN_POINT('Ctrl Pts',(12.8428057266944,14.8502347891476,21.));
#17262=CARTESIAN_POINT('Ctrl Pts',(12.8624032236317,14.8945191569251,0.));
#17263=CARTESIAN_POINT('Ctrl Pts',(12.8624032236317,14.8945191569251,21.));
#17264=CARTESIAN_POINT('Ctrl Pts',(12.8816587472147,14.9390408507356,0.));
#17265=CARTESIAN_POINT('Ctrl Pts',(12.8816587472147,14.9390408507356,21.));
#17266=CARTESIAN_POINT('Ctrl Pts',(12.9005620742036,14.9838057866976,0.));
#17267=CARTESIAN_POINT('Ctrl Pts',(12.9005620742036,14.9838057866976,21.));
#17268=CARTESIAN_POINT('Ctrl Pts',(12.9191164383568,15.0288099208306,0.));
#17269=CARTESIAN_POINT('Ctrl Pts',(12.9191164383568,15.0288099208306,21.));
#17270=CARTESIAN_POINT('Ctrl Pts',(12.9373327960422,15.0740435169624,0.));
#17271=CARTESIAN_POINT('Ctrl Pts',(12.9373327960422,15.0740435169624,21.));
#17272=CARTESIAN_POINT('Ctrl Pts',(12.9552263908864,15.1194937003528,0.));
#17273=CARTESIAN_POINT('Ctrl Pts',(12.9552263908864,15.1194937003528,21.));
#17274=CARTESIAN_POINT('Ctrl Pts',(12.9728126886697,15.1651474813659,0.));
#17275=CARTESIAN_POINT('Ctrl Pts',(12.9728126886697,15.1651474813659,21.));
#17276=CARTESIAN_POINT('Ctrl Pts',(12.9901029059182,15.2109950816083,0.));
#17277=CARTESIAN_POINT('Ctrl Pts',(12.9901029059182,15.2109950816083,21.));
#17278=CARTESIAN_POINT('Ctrl Pts',(13.0071020851025,15.2570313635503,0.));
#17279=CARTESIAN_POINT('Ctrl Pts',(13.0071020851025,15.2570313635503,21.));
#17280=CARTESIAN_POINT('Ctrl Pts',(13.0238115816728,15.3032539741328,0.));
#17281=CARTESIAN_POINT('Ctrl Pts',(13.0238115816728,15.3032539741328,21.));
#17282=CARTESIAN_POINT('Ctrl Pts',(13.0402305665115,15.3496622219036,0.));
#17283=CARTESIAN_POINT('Ctrl Pts',(13.0402305665115,15.3496622219036,21.));
#17284=CARTESIAN_POINT('Ctrl Pts',(13.0563577967298,15.3962557545684,0.));
#17285=CARTESIAN_POINT('Ctrl Pts',(13.0563577967298,15.3962557545684,21.));
#17286=CARTESIAN_POINT('Ctrl Pts',(13.0721935806302,15.4430330918328,0.));
#17287=CARTESIAN_POINT('Ctrl Pts',(13.0721935806302,15.4430330918328,21.));
#17288=CARTESIAN_POINT('Ctrl Pts',(13.087740560189,15.4899910401523,0.));
#17289=CARTESIAN_POINT('Ctrl Pts',(13.087740560189,15.4899910401523,21.));
#17290=CARTESIAN_POINT('Ctrl Pts',(13.1030026646917,15.5371254712111,0.));
#17291=CARTESIAN_POINT('Ctrl Pts',(13.1030026646917,15.5371254712111,21.));
#17292=CARTESIAN_POINT('Ctrl Pts',(13.1179844917497,15.5844317820184,0.));
#17293=CARTESIAN_POINT('Ctrl Pts',(13.1179844917497,15.5844317820184,21.));
#17294=CARTESIAN_POINT('Ctrl Pts',(13.1326905726717,15.6319054413079,0.));
#17295=CARTESIAN_POINT('Ctrl Pts',(13.1326905726717,15.6319054413079,21.));
#17296=CARTESIAN_POINT('Ctrl Pts',(13.147124558532,15.6795425955901,0.));
#17297=CARTESIAN_POINT('Ctrl Pts',(13.147124558532,15.6795425955901,21.));
#17298=CARTESIAN_POINT('Ctrl Pts',(13.161288914421,15.7273402954914,0.));
#17299=CARTESIAN_POINT('Ctrl Pts',(13.161288914421,15.7273402954914,21.));
#17300=CARTESIAN_POINT('Ctrl Pts',(13.1751853728467,15.7752961549278,0.));
#17301=CARTESIAN_POINT('Ctrl Pts',(13.1751853728467,15.7752961549278,21.));
#17302=CARTESIAN_POINT('Ctrl Pts',(13.1888152101588,15.8234081427091,0.));
#17303=CARTESIAN_POINT('Ctrl Pts',(13.1888152101588,15.8234081427091,21.));
#17304=CARTESIAN_POINT('Ctrl Pts',(13.2021795724682,15.8716743375555,0.));
#17305=CARTESIAN_POINT('Ctrl Pts',(13.2021795724682,15.8716743375555,21.));
#17306=CARTESIAN_POINT('Ctrl Pts',(13.2152798388134,15.9200926550954,0.));
#17307=CARTESIAN_POINT('Ctrl Pts',(13.2152798388134,15.9200926550954,21.));
#17308=CARTESIAN_POINT('Ctrl Pts',(13.2281177675127,15.9686607385389,0.));
#17309=CARTESIAN_POINT('Ctrl Pts',(13.2281177675127,15.9686607385389,21.));
#17310=CARTESIAN_POINT('Ctrl Pts',(13.240695304984,16.0173761036734,0.));
#17311=CARTESIAN_POINT('Ctrl Pts',(13.240695304984,16.0173761036734,21.));
#17312=CARTESIAN_POINT('Ctrl Pts',(13.2530144750236,16.0662362238032,0.));
#17313=CARTESIAN_POINT('Ctrl Pts',(13.2530144750236,16.0662362238032,21.));
#17314=CARTESIAN_POINT('Ctrl Pts',(13.2650772466062,16.1152386305152,0.));
#17315=CARTESIAN_POINT('Ctrl Pts',(13.2650772466062,16.1152386305152,21.));
#17316=CARTESIAN_POINT('Ctrl Pts',(13.2768853909882,16.1643810242643,0.));
#17317=CARTESIAN_POINT('Ctrl Pts',(13.2768853909882,16.1643810242643,21.));
#17318=CARTESIAN_POINT('Ctrl Pts',(13.2884404210388,16.2136613184475,0.));
#17319=CARTESIAN_POINT('Ctrl Pts',(13.2884404210388,16.2136613184475,21.));
#17320=CARTESIAN_POINT('Ctrl Pts',(13.2997436744733,16.2630775678735,0.));
#17321=CARTESIAN_POINT('Ctrl Pts',(13.2997436744733,16.2630775678735,21.));
#17322=CARTESIAN_POINT('Ctrl Pts',(13.3107963665229,16.3126279218067,0.));
#17323=CARTESIAN_POINT('Ctrl Pts',(13.3107963665229,16.3126279218067,21.));
#17324=CARTESIAN_POINT('Ctrl Pts',(13.3215996524974,16.3623105703343,0.));
#17325=CARTESIAN_POINT('Ctrl Pts',(13.3215996524974,16.3623105703343,21.));
#17326=CARTESIAN_POINT('Ctrl Pts',(13.3321546976812,16.4121236828756,0.));
#17327=CARTESIAN_POINT('Ctrl Pts',(13.3321546976812,16.4121236828756,21.));
#17328=CARTESIAN_POINT('Ctrl Pts',(13.3424627129921,16.4620653818862,0.));
#17329=CARTESIAN_POINT('Ctrl Pts',(13.3424627129921,16.4620653818862,21.));
#17330=CARTESIAN_POINT('Ctrl Pts',(13.3525249163084,16.5121337902953,0.));
#17331=CARTESIAN_POINT('Ctrl Pts',(13.3525249163084,16.5121337902953,21.));
#17332=CARTESIAN_POINT('Ctrl Pts',(13.3623425108873,16.5623270636327,0.));
#17333=CARTESIAN_POINT('Ctrl Pts',(13.3623425108873,16.5623270636327,21.));
#17334=CARTESIAN_POINT('Ctrl Pts',(13.3719166600676,16.612643424234,0.));
#17335=CARTESIAN_POINT('Ctrl Pts',(13.3719166600676,16.612643424234,21.));
#17336=CARTESIAN_POINT('Ctrl Pts',(13.381248462113,16.6630812012276,0.));
#17337=CARTESIAN_POINT('Ctrl Pts',(13.381248462113,16.6630812012276,21.));
#17338=CARTESIAN_POINT('Ctrl Pts',(13.3903389370346,16.7136388432444,0.));
#17339=CARTESIAN_POINT('Ctrl Pts',(13.3903389370346,16.7136388432444,21.));
#17340=CARTESIAN_POINT('Ctrl Pts',(13.3991890464165,16.7643148579873,0.));
#17341=CARTESIAN_POINT('Ctrl Pts',(13.3991890464165,16.7643148579873,21.));
#17342=CARTESIAN_POINT('Ctrl Pts',(13.4077997088426,16.8151077630226,0.));
#17343=CARTESIAN_POINT('Ctrl Pts',(13.4077997088426,16.8151077630226,21.));
#17344=CARTESIAN_POINT('Ctrl Pts',(13.4161718177499,16.8660160353187,0.));
#17345=CARTESIAN_POINT('Ctrl Pts',(13.4161718177499,16.8660160353187,21.));
#17346=CARTESIAN_POINT('Ctrl Pts',(13.4243062623592,16.9170380509036,0.));
#17347=CARTESIAN_POINT('Ctrl Pts',(13.4243062623592,16.9170380509036,21.));
#17348=CARTESIAN_POINT('Ctrl Pts',(13.432203941793,16.9681720567298,0.));
#17349=CARTESIAN_POINT('Ctrl Pts',(13.432203941793,16.9681720567298,21.));
#17350=CARTESIAN_POINT('Ctrl Pts',(13.4398657451291,17.0194162803447,0.));
#17351=CARTESIAN_POINT('Ctrl Pts',(13.4398657451291,17.0194162803447,21.));
#17352=CARTESIAN_POINT('Ctrl Pts',(13.4472925380889,17.0707690194412,0.));
#17353=CARTESIAN_POINT('Ctrl Pts',(13.4472925380889,17.0707690194412,21.));
#17354=CARTESIAN_POINT('Ctrl Pts',(13.4544851484583,17.1222287365697,0.));
#17355=CARTESIAN_POINT('Ctrl Pts',(13.4544851484583,17.1222287365697,21.));
#17356=CARTESIAN_POINT('Ctrl Pts',(13.4614443545811,17.173794155624,0.));
#17357=CARTESIAN_POINT('Ctrl Pts',(13.4614443545811,17.173794155624,21.));
#17358=CARTESIAN_POINT('Ctrl Pts',(13.4681708717969,17.2254643437923,0.));
#17359=CARTESIAN_POINT('Ctrl Pts',(13.4681708717969,17.2254643437923,21.));
#17360=CARTESIAN_POINT('Ctrl Pts',(13.474665315482,17.2772386565028,0.));
#17361=CARTESIAN_POINT('Ctrl Pts',(13.474665315482,17.2772386565028,21.));
#17362=CARTESIAN_POINT('Ctrl Pts',(13.4796755969465,17.3187410868027,0.));
#17363=CARTESIAN_POINT('Ctrl Pts',(13.4796755969465,17.3187410868027,21.));
#17364=CARTESIAN_POINT('Ctrl Pts',(13.4833292332349,17.3499144948292,0.));
#17365=CARTESIAN_POINT('Ctrl Pts',(13.4833292332349,17.3499144948292,21.));
#17366=CARTESIAN_POINT('Ctrl Pts',(13.485718750657,17.3707174645609,0.));
#17367=CARTESIAN_POINT('Ctrl Pts',(13.485718750657,17.3707174645609,21.));
#17368=CARTESIAN_POINT('Ctrl Pts',(13.4869019493419,17.3811241238545,0.));
#17369=CARTESIAN_POINT('Ctrl Pts',(13.4869019493419,17.3811241238545,21.));
#17370=CARTESIAN_POINT('Ctrl Pts',(12.4172651441477,14.1074595503134,0.));
#17371=CARTESIAN_POINT('Ctrl Pts',(12.4234926340671,14.1145347042316,0.));
#17372=CARTESIAN_POINT('Ctrl Pts',(12.4357509724316,14.1288394445866,0.));
#17373=CARTESIAN_POINT('Ctrl Pts',(12.4535485619996,14.1507598477672,0.));
#17374=CARTESIAN_POINT('Ctrl Pts',(12.4761570639125,14.1808688343892,0.));
#17375=CARTESIAN_POINT('Ctrl Pts',(12.5028859651751,14.2197144660135,0.));
#17376=CARTESIAN_POINT('Ctrl Pts',(12.5285125321527,14.2594378207584,0.));
#17377=CARTESIAN_POINT('Ctrl Pts',(12.5534605602317,14.2997103098726,0.));
#17378=CARTESIAN_POINT('Ctrl Pts',(12.5780443898087,14.3402859058353,0.));
#17379=CARTESIAN_POINT('Ctrl Pts',(12.6023830189244,14.3810669346235,0.));
#17380=CARTESIAN_POINT('Ctrl Pts',(12.626464614311,14.4220553460485,0.));
#17381=CARTESIAN_POINT('Ctrl Pts',(12.6501984687124,14.463313553928,0.));
#17382=CARTESIAN_POINT('Ctrl Pts',(12.6734695081852,14.5049233087958,0.));
#17383=CARTESIAN_POINT('Ctrl Pts',(12.6961966430455,14.5469417071951,0.));
#17384=CARTESIAN_POINT('Ctrl Pts',(12.7183743139638,14.5893698147583,0.));
#17385=CARTESIAN_POINT('Ctrl Pts',(12.7400427996251,14.6321748083434,0.));
#17386=CARTESIAN_POINT('Ctrl Pts',(12.7612687078867,14.6753044633399,0.));
#17387=CARTESIAN_POINT('Ctrl Pts',(12.7821227233337,14.7187037124277,0.));
#17388=CARTESIAN_POINT('Ctrl Pts',(12.8026557145457,14.7623324139791,0.));
#17389=CARTESIAN_POINT('Ctrl Pts',(12.8228846016791,14.8061758577898,0.));
#17390=CARTESIAN_POINT('Ctrl Pts',(12.8428057266944,14.8502347891476,0.));
#17391=CARTESIAN_POINT('Ctrl Pts',(12.8624032236317,14.8945191569251,0.));
#17392=CARTESIAN_POINT('Ctrl Pts',(12.8816587472147,14.9390408507356,0.));
#17393=CARTESIAN_POINT('Ctrl Pts',(12.9005620742036,14.9838057866976,0.));
#17394=CARTESIAN_POINT('Ctrl Pts',(12.9191164383568,15.0288099208306,0.));
#17395=CARTESIAN_POINT('Ctrl Pts',(12.9373327960422,15.0740435169624,0.));
#17396=CARTESIAN_POINT('Ctrl Pts',(12.9552263908864,15.1194937003528,0.));
#17397=CARTESIAN_POINT('Ctrl Pts',(12.9728126886697,15.1651474813659,0.));
#17398=CARTESIAN_POINT('Ctrl Pts',(12.9901029059182,15.2109950816083,0.));
#17399=CARTESIAN_POINT('Ctrl Pts',(13.0071020851025,15.2570313635503,0.));
#17400=CARTESIAN_POINT('Ctrl Pts',(13.0238115816728,15.3032539741328,0.));
#17401=CARTESIAN_POINT('Ctrl Pts',(13.0402305665115,15.3496622219036,0.));
#17402=CARTESIAN_POINT('Ctrl Pts',(13.0563577967298,15.3962557545684,0.));
#17403=CARTESIAN_POINT('Ctrl Pts',(13.0721935806302,15.4430330918328,0.));
#17404=CARTESIAN_POINT('Ctrl Pts',(13.087740560189,15.4899910401523,0.));
#17405=CARTESIAN_POINT('Ctrl Pts',(13.1030026646917,15.5371254712111,0.));
#17406=CARTESIAN_POINT('Ctrl Pts',(13.1179844917497,15.5844317820184,0.));
#17407=CARTESIAN_POINT('Ctrl Pts',(13.1326905726717,15.6319054413079,0.));
#17408=CARTESIAN_POINT('Ctrl Pts',(13.147124558532,15.6795425955901,0.));
#17409=CARTESIAN_POINT('Ctrl Pts',(13.161288914421,15.7273402954914,0.));
#17410=CARTESIAN_POINT('Ctrl Pts',(13.1751853728467,15.7752961549278,0.));
#17411=CARTESIAN_POINT('Ctrl Pts',(13.1888152101588,15.8234081427091,0.));
#17412=CARTESIAN_POINT('Ctrl Pts',(13.2021795724682,15.8716743375555,0.));
#17413=CARTESIAN_POINT('Ctrl Pts',(13.2152798388134,15.9200926550954,0.));
#17414=CARTESIAN_POINT('Ctrl Pts',(13.2281177675127,15.9686607385389,0.));
#17415=CARTESIAN_POINT('Ctrl Pts',(13.240695304984,16.0173761036734,0.));
#17416=CARTESIAN_POINT('Ctrl Pts',(13.2530144750236,16.0662362238032,0.));
#17417=CARTESIAN_POINT('Ctrl Pts',(13.2650772466062,16.1152386305152,0.));
#17418=CARTESIAN_POINT('Ctrl Pts',(13.2768853909882,16.1643810242643,0.));
#17419=CARTESIAN_POINT('Ctrl Pts',(13.2884404210388,16.2136613184475,0.));
#17420=CARTESIAN_POINT('Ctrl Pts',(13.2997436744733,16.2630775678735,0.));
#17421=CARTESIAN_POINT('Ctrl Pts',(13.3107963665229,16.3126279218067,0.));
#17422=CARTESIAN_POINT('Ctrl Pts',(13.3215996524974,16.3623105703343,0.));
#17423=CARTESIAN_POINT('Ctrl Pts',(13.3321546976812,16.4121236828756,0.));
#17424=CARTESIAN_POINT('Ctrl Pts',(13.3424627129921,16.4620653818862,0.));
#17425=CARTESIAN_POINT('Ctrl Pts',(13.3525249163084,16.5121337902953,0.));
#17426=CARTESIAN_POINT('Ctrl Pts',(13.3623425108873,16.5623270636327,0.));
#17427=CARTESIAN_POINT('Ctrl Pts',(13.3719166600676,16.612643424234,0.));
#17428=CARTESIAN_POINT('Ctrl Pts',(13.381248462113,16.6630812012276,0.));
#17429=CARTESIAN_POINT('Ctrl Pts',(13.3903389370346,16.7136388432444,0.));
#17430=CARTESIAN_POINT('Ctrl Pts',(13.3991890464165,16.7643148579873,0.));
#17431=CARTESIAN_POINT('Ctrl Pts',(13.4077997088426,16.8151077630226,0.));
#17432=CARTESIAN_POINT('Ctrl Pts',(13.4161718177499,16.8660160353187,0.));
#17433=CARTESIAN_POINT('Ctrl Pts',(13.4243062623592,16.9170380509036,0.));
#17434=CARTESIAN_POINT('Ctrl Pts',(13.432203941793,16.9681720567298,0.));
#17435=CARTESIAN_POINT('Ctrl Pts',(13.4398657451291,17.0194162803447,0.));
#17436=CARTESIAN_POINT('Ctrl Pts',(13.4472925380889,17.0707690194412,0.));
#17437=CARTESIAN_POINT('Ctrl Pts',(13.4544851484583,17.1222287365697,0.));
#17438=CARTESIAN_POINT('Ctrl Pts',(13.4614443545811,17.173794155624,0.));
#17439=CARTESIAN_POINT('Ctrl Pts',(13.4695161752401,17.235798381426,0.));
#17440=CARTESIAN_POINT('Ctrl Pts',(13.4759526005425,17.287598725272,0.));
#17441=CARTESIAN_POINT('Ctrl Pts',(13.4809165957478,17.3291218739796,0.));
#17442=CARTESIAN_POINT('Ctrl Pts',(13.4845355519784,17.360310805254,0.));
#17443=CARTESIAN_POINT('Ctrl Pts',(13.4869019493419,17.3811241238545,0.));
#17444=CARTESIAN_POINT('Ctrl Pts',(12.4172651441477,14.1074595503134,13.));
#17445=CARTESIAN_POINT('Ctrl Pts',(12.4277613166149,14.1193844248164,13.));
#17446=CARTESIAN_POINT('Ctrl Pts',(12.4379186757848,14.1315753314249,13.));
#17447=CARTESIAN_POINT('Ctrl Pts',(12.4477599775084,14.14401474732,13.));
#17448=CARTESIAN_POINT('Ctrl Pts',(12.45929471922,14.1585946731696,13.));
#17449=CARTESIAN_POINT('Ctrl Pts',(12.4703959522577,14.1735154808295,13.));
#17450=CARTESIAN_POINT('Ctrl Pts',(12.4811568677436,14.1887053040703,13.));
#17451=CARTESIAN_POINT('Ctrl Pts',(12.4962979908344,14.2100781123335,13.));
#17452=CARTESIAN_POINT('Ctrl Pts',(12.5107710847127,14.2319791941756,13.));
#17453=CARTESIAN_POINT('Ctrl Pts',(12.5249003586941,14.254157574695,13.));
#17454=CARTESIAN_POINT('Ctrl Pts',(12.5342985542355,14.2689096955178,13.));
#17455=CARTESIAN_POINT('Ctrl Pts',(12.5435462296413,14.2837832480516,13.));
#17456=CARTESIAN_POINT('Ctrl Pts',(12.5527146050322,14.298722508524,13.));
#17457=CARTESIAN_POINT('Ctrl Pts',(12.5623658230416,14.3144485290642,13.));
#17458=CARTESIAN_POINT('Ctrl Pts',(12.5719298675028,14.330246820686,13.));
#17459=CARTESIAN_POINT('Ctrl Pts',(12.5814385821519,14.3460912752807,13.));
#17460=CARTESIAN_POINT('Ctrl Pts',(12.5919985302804,14.3636874094394,13.));
#17461=CARTESIAN_POINT('Ctrl Pts',(12.6024891912727,14.381341260665,13.));
#17462=CARTESIAN_POINT('Ctrl Pts',(12.6128991700701,14.3990589912032,13.));
#17463=CARTESIAN_POINT('Ctrl Pts',(12.6285927183677,14.4257693299403,13.));
#17464=CARTESIAN_POINT('Ctrl Pts',(12.6440977931351,14.452628589856,13.));
#17465=CARTESIAN_POINT('Ctrl Pts',(12.6592867998067,14.4797266308813,13.));
#17466=CARTESIAN_POINT('Ctrl Pts',(12.6703212810873,14.4994127652612,13.));
#17467=CARTESIAN_POINT('Ctrl Pts',(12.6811863451307,14.5192269386383,13.));
#17468=CARTESIAN_POINT('Ctrl Pts',(12.6918647171384,14.5391805041508,13.));
#17469=CARTESIAN_POINT('Ctrl Pts',(12.7049181125412,14.5635720293893,13.));
#17470=CARTESIAN_POINT('Ctrl Pts',(12.7176935524276,14.5881710816651,13.));
#17471=CARTESIAN_POINT('Ctrl Pts',(12.7302281821981,14.612947560673,13.));
#17472=CARTESIAN_POINT('Ctrl Pts',(12.7437676626773,14.6397102700639,13.));
#17473=CARTESIAN_POINT('Ctrl Pts',(12.7570309720221,14.6666764215902,13.));
#17474=CARTESIAN_POINT('Ctrl Pts',(12.7700903554915,14.6937895363403,13.));
#17475=CARTESIAN_POINT('Ctrl Pts',(12.7821467169645,14.7188202365146,13.));
#17476=CARTESIAN_POINT('Ctrl Pts',(12.7940312932615,14.7439746960234,13.));
#17477=CARTESIAN_POINT('Ctrl Pts',(12.8057660290113,14.7692347187417,13.));
#17478=CARTESIAN_POINT('Ctrl Pts',(12.8217082700361,14.8035517565561,13.));
#17479=CARTESIAN_POINT('Ctrl Pts',(12.8373723698026,14.8380647951195,13.));
#17480=CARTESIAN_POINT('Ctrl Pts',(12.8527323828633,14.8727890594696,13.));
#17481=CARTESIAN_POINT('Ctrl Pts',(12.8675544637349,14.9062972246236,13.));
#17482=CARTESIAN_POINT('Ctrl Pts',(12.8820871276608,14.940006753605,13.));
#17483=CARTESIAN_POINT('Ctrl Pts',(12.8963159096104,14.9739251233869,13.));
#17484=CARTESIAN_POINT('Ctrl Pts',(12.9156461084297,15.0200041787713,13.));
#17485=CARTESIAN_POINT('Ctrl Pts',(12.9344180544732,15.0664667162891,13.));
#17486=CARTESIAN_POINT('Ctrl Pts',(12.9526968521391,15.113256758699,13.));
#17487=CARTESIAN_POINT('Ctrl Pts',(12.9687635180149,15.1543841890393,13.));
#17488=CARTESIAN_POINT('Ctrl Pts',(12.9844546719612,15.1957605758326,13.));
#17489=CARTESIAN_POINT('Ctrl Pts',(12.999793846462,15.2373637638652,13.));
#17490=CARTESIAN_POINT('Ctrl Pts',(13.0224075138868,15.2986969638966,13.));
#17491=CARTESIAN_POINT('Ctrl Pts',(13.0442489122257,15.3605284720897,13.));
#17492=CARTESIAN_POINT('Ctrl Pts',(13.0653151028224,15.4228468914086,13.));
#17493=CARTESIAN_POINT('Ctrl Pts',(13.0919008408212,15.5014933444024,13.));
#17494=CARTESIAN_POINT('Ctrl Pts',(13.1172560779922,15.5809121483295,13.));
#17495=CARTESIAN_POINT('Ctrl Pts',(13.1414683121752,15.6610132193997,13.));
#17496=CARTESIAN_POINT('Ctrl Pts',(13.1742656500619,15.7695162957013,13.));
#17497=CARTESIAN_POINT('Ctrl Pts',(13.2049609859129,15.8792747460677,13.));
#17498=CARTESIAN_POINT('Ctrl Pts',(13.2336341230255,15.9901726543658,13.));
#17499=CARTESIAN_POINT('Ctrl Pts',(13.2591969755608,16.0890410434498,13.));
#17500=CARTESIAN_POINT('Ctrl Pts',(13.2831593507059,16.1888100045206,13.));
#17501=CARTESIAN_POINT('Ctrl Pts',(13.3055799353303,16.2893994154296,13.));
#17502=CARTESIAN_POINT('Ctrl Pts',(13.3373560689398,16.4319622706935,13.));
#17503=CARTESIAN_POINT('Ctrl Pts',(13.3660302358948,16.576175723372,13.));
#17504=CARTESIAN_POINT('Ctrl Pts',(13.3917254914339,16.7218506169446,13.));
#17505=CARTESIAN_POINT('Ctrl Pts',(13.4116849578761,16.8350074269757,13.));
#17506=CARTESIAN_POINT('Ctrl Pts',(13.4298451931126,16.9490507057181,13.));
#17507=CARTESIAN_POINT('Ctrl Pts',(13.4462507328471,17.0638967767752,13.));
#17508=CARTESIAN_POINT('Ctrl Pts',(13.4604427660419,17.163247318062,13.));
#17509=CARTESIAN_POINT('Ctrl Pts',(13.4733230165186,17.2631945724315,13.));
#17510=CARTESIAN_POINT('Ctrl Pts',(13.4849093842842,17.3637184372217,13.));
#17511=CARTESIAN_POINT('Ctrl Pts',(13.4855778874128,17.3695184014096,13.));
#17512=CARTESIAN_POINT('Ctrl Pts',(13.4862420756862,17.3753202969914,13.));
#17513=CARTESIAN_POINT('Ctrl Pts',(13.4869019493419,17.3811241238545,13.));
#17514=CARTESIAN_POINT('Ctrl Pts',(17.3811241238545,13.4869019493419,0.));
#17515=CARTESIAN_POINT('Ctrl Pts',(17.3811241238545,13.4869019493419,21.));
#17516=CARTESIAN_POINT('Ctrl Pts',(17.3707174645609,13.485718750657,0.));
#17517=CARTESIAN_POINT('Ctrl Pts',(17.3707174645609,13.485718750657,21.));
#17518=CARTESIAN_POINT('Ctrl Pts',(17.3499144948292,13.4833292332349,0.));
#17519=CARTESIAN_POINT('Ctrl Pts',(17.3499144948292,13.4833292332349,21.));
#17520=CARTESIAN_POINT('Ctrl Pts',(17.3187410868027,13.4796755969465,0.));
#17521=CARTESIAN_POINT('Ctrl Pts',(17.3187410868027,13.4796755969465,21.));
#17522=CARTESIAN_POINT('Ctrl Pts',(17.2772386565028,13.474665315482,0.));
#17523=CARTESIAN_POINT('Ctrl Pts',(17.2772386565028,13.474665315482,21.));
#17524=CARTESIAN_POINT('Ctrl Pts',(17.2254643437923,13.4681708717969,0.));
#17525=CARTESIAN_POINT('Ctrl Pts',(17.2254643437923,13.4681708717969,21.));
#17526=CARTESIAN_POINT('Ctrl Pts',(17.173794155624,13.4614443545811,0.));
#17527=CARTESIAN_POINT('Ctrl Pts',(17.173794155624,13.4614443545811,21.));
#17528=CARTESIAN_POINT('Ctrl Pts',(17.1222287365697,13.4544851484583,0.));
#17529=CARTESIAN_POINT('Ctrl Pts',(17.1222287365697,13.4544851484583,21.));
#17530=CARTESIAN_POINT('Ctrl Pts',(17.0707690194411,13.4472925380889,0.));
#17531=CARTESIAN_POINT('Ctrl Pts',(17.0707690194411,13.4472925380889,21.));
#17532=CARTESIAN_POINT('Ctrl Pts',(17.0194162803447,13.4398657451291,0.));
#17533=CARTESIAN_POINT('Ctrl Pts',(17.0194162803447,13.4398657451291,21.));
#17534=CARTESIAN_POINT('Ctrl Pts',(16.9681720567298,13.432203941793,0.));
#17535=CARTESIAN_POINT('Ctrl Pts',(16.9681720567298,13.432203941793,21.));
#17536=CARTESIAN_POINT('Ctrl Pts',(16.9170380509036,13.4243062623592,0.));
#17537=CARTESIAN_POINT('Ctrl Pts',(16.9170380509036,13.4243062623592,21.));
#17538=CARTESIAN_POINT('Ctrl Pts',(16.8660160353187,13.4161718177499,0.));
#17539=CARTESIAN_POINT('Ctrl Pts',(16.8660160353187,13.4161718177499,21.));
#17540=CARTESIAN_POINT('Ctrl Pts',(16.8151077630226,13.4077997088426,0.));
#17541=CARTESIAN_POINT('Ctrl Pts',(16.8151077630226,13.4077997088426,21.));
#17542=CARTESIAN_POINT('Ctrl Pts',(16.7643148579873,13.3991890464165,0.));
#17543=CARTESIAN_POINT('Ctrl Pts',(16.7643148579873,13.3991890464165,21.));
#17544=CARTESIAN_POINT('Ctrl Pts',(16.7136388432444,13.3903389370346,0.));
#17545=CARTESIAN_POINT('Ctrl Pts',(16.7136388432444,13.3903389370346,21.));
#17546=CARTESIAN_POINT('Ctrl Pts',(16.6630812012276,13.381248462113,0.));
#17547=CARTESIAN_POINT('Ctrl Pts',(16.6630812012276,13.381248462113,21.));
#17548=CARTESIAN_POINT('Ctrl Pts',(16.612643424234,13.3719166600676,0.));
#17549=CARTESIAN_POINT('Ctrl Pts',(16.612643424234,13.3719166600676,21.));
#17550=CARTESIAN_POINT('Ctrl Pts',(16.5623270636327,13.3623425108873,0.));
#17551=CARTESIAN_POINT('Ctrl Pts',(16.5623270636327,13.3623425108873,21.));
#17552=CARTESIAN_POINT('Ctrl Pts',(16.5121337902953,13.3525249163084,0.));
#17553=CARTESIAN_POINT('Ctrl Pts',(16.5121337902953,13.3525249163084,21.));
#17554=CARTESIAN_POINT('Ctrl Pts',(16.4620653818862,13.3424627129921,0.));
#17555=CARTESIAN_POINT('Ctrl Pts',(16.4620653818862,13.3424627129921,21.));
#17556=CARTESIAN_POINT('Ctrl Pts',(16.4121236828756,13.3321546976812,0.));
#17557=CARTESIAN_POINT('Ctrl Pts',(16.4121236828756,13.3321546976812,21.));
#17558=CARTESIAN_POINT('Ctrl Pts',(16.3623105703343,13.3215996524974,0.));
#17559=CARTESIAN_POINT('Ctrl Pts',(16.3623105703343,13.3215996524974,21.));
#17560=CARTESIAN_POINT('Ctrl Pts',(16.3126279218067,13.3107963665229,0.));
#17561=CARTESIAN_POINT('Ctrl Pts',(16.3126279218067,13.3107963665229,21.));
#17562=CARTESIAN_POINT('Ctrl Pts',(16.2630775678735,13.2997436744733,0.));
#17563=CARTESIAN_POINT('Ctrl Pts',(16.2630775678735,13.2997436744733,21.));
#17564=CARTESIAN_POINT('Ctrl Pts',(16.2136613184475,13.2884404210387,0.));
#17565=CARTESIAN_POINT('Ctrl Pts',(16.2136613184475,13.2884404210387,21.));
#17566=CARTESIAN_POINT('Ctrl Pts',(16.1643810242643,13.2768853909882,0.));
#17567=CARTESIAN_POINT('Ctrl Pts',(16.1643810242643,13.2768853909882,21.));
#17568=CARTESIAN_POINT('Ctrl Pts',(16.1152386305152,13.2650772466062,0.));
#17569=CARTESIAN_POINT('Ctrl Pts',(16.1152386305152,13.2650772466062,21.));
#17570=CARTESIAN_POINT('Ctrl Pts',(16.0662362238032,13.2530144750236,0.));
#17571=CARTESIAN_POINT('Ctrl Pts',(16.0662362238032,13.2530144750236,21.));
#17572=CARTESIAN_POINT('Ctrl Pts',(16.0173761036734,13.240695304984,0.));
#17573=CARTESIAN_POINT('Ctrl Pts',(16.0173761036734,13.240695304984,21.));
#17574=CARTESIAN_POINT('Ctrl Pts',(15.9686607385389,13.2281177675127,0.));
#17575=CARTESIAN_POINT('Ctrl Pts',(15.9686607385389,13.2281177675127,21.));
#17576=CARTESIAN_POINT('Ctrl Pts',(15.9200926550954,13.2152798388134,0.));
#17577=CARTESIAN_POINT('Ctrl Pts',(15.9200926550954,13.2152798388134,21.));
#17578=CARTESIAN_POINT('Ctrl Pts',(15.8716743375555,13.2021795724682,0.));
#17579=CARTESIAN_POINT('Ctrl Pts',(15.8716743375555,13.2021795724682,21.));
#17580=CARTESIAN_POINT('Ctrl Pts',(15.8234081427091,13.1888152101588,0.));
#17581=CARTESIAN_POINT('Ctrl Pts',(15.8234081427091,13.1888152101588,21.));
#17582=CARTESIAN_POINT('Ctrl Pts',(15.7752961549278,13.1751853728467,0.));
#17583=CARTESIAN_POINT('Ctrl Pts',(15.7752961549278,13.1751853728467,21.));
#17584=CARTESIAN_POINT('Ctrl Pts',(15.7273402954914,13.161288914421,0.));
#17585=CARTESIAN_POINT('Ctrl Pts',(15.7273402954914,13.161288914421,21.));
#17586=CARTESIAN_POINT('Ctrl Pts',(15.6795425955901,13.147124558532,0.));
#17587=CARTESIAN_POINT('Ctrl Pts',(15.6795425955901,13.147124558532,21.));
#17588=CARTESIAN_POINT('Ctrl Pts',(15.6319054413079,13.1326905726717,0.));
#17589=CARTESIAN_POINT('Ctrl Pts',(15.6319054413079,13.1326905726717,21.));
#17590=CARTESIAN_POINT('Ctrl Pts',(15.5844317820184,13.1179844917497,0.));
#17591=CARTESIAN_POINT('Ctrl Pts',(15.5844317820184,13.1179844917497,21.));
#17592=CARTESIAN_POINT('Ctrl Pts',(15.5371254712111,13.1030026646917,0.));
#17593=CARTESIAN_POINT('Ctrl Pts',(15.5371254712111,13.1030026646917,21.));
#17594=CARTESIAN_POINT('Ctrl Pts',(15.4899910401523,13.087740560189,0.));
#17595=CARTESIAN_POINT('Ctrl Pts',(15.4899910401523,13.087740560189,21.));
#17596=CARTESIAN_POINT('Ctrl Pts',(15.4430330918328,13.0721935806302,0.));
#17597=CARTESIAN_POINT('Ctrl Pts',(15.4430330918328,13.0721935806302,21.));
#17598=CARTESIAN_POINT('Ctrl Pts',(15.3962557545684,13.0563577967298,0.));
#17599=CARTESIAN_POINT('Ctrl Pts',(15.3962557545684,13.0563577967298,21.));
#17600=CARTESIAN_POINT('Ctrl Pts',(15.3496622219036,13.0402305665115,0.));
#17601=CARTESIAN_POINT('Ctrl Pts',(15.3496622219036,13.0402305665115,21.));
#17602=CARTESIAN_POINT('Ctrl Pts',(15.3032539741328,13.0238115816728,0.));
#17603=CARTESIAN_POINT('Ctrl Pts',(15.3032539741328,13.0238115816728,21.));
#17604=CARTESIAN_POINT('Ctrl Pts',(15.2570313635503,13.0071020851025,0.));
#17605=CARTESIAN_POINT('Ctrl Pts',(15.2570313635503,13.0071020851025,21.));
#17606=CARTESIAN_POINT('Ctrl Pts',(15.2109950816083,12.9901029059182,0.));
#17607=CARTESIAN_POINT('Ctrl Pts',(15.2109950816083,12.9901029059182,21.));
#17608=CARTESIAN_POINT('Ctrl Pts',(15.1651474813659,12.9728126886697,0.));
#17609=CARTESIAN_POINT('Ctrl Pts',(15.1651474813659,12.9728126886697,21.));
#17610=CARTESIAN_POINT('Ctrl Pts',(15.1194937003528,12.9552263908864,0.));
#17611=CARTESIAN_POINT('Ctrl Pts',(15.1194937003528,12.9552263908864,21.));
#17612=CARTESIAN_POINT('Ctrl Pts',(15.0740435169624,12.9373327960422,0.));
#17613=CARTESIAN_POINT('Ctrl Pts',(15.0740435169624,12.9373327960422,21.));
#17614=CARTESIAN_POINT('Ctrl Pts',(15.0288099208306,12.9191164383568,0.));
#17615=CARTESIAN_POINT('Ctrl Pts',(15.0288099208306,12.9191164383568,21.));
#17616=CARTESIAN_POINT('Ctrl Pts',(14.9838057866976,12.9005620742036,0.));
#17617=CARTESIAN_POINT('Ctrl Pts',(14.9838057866976,12.9005620742036,21.));
#17618=CARTESIAN_POINT('Ctrl Pts',(14.9390408507356,12.8816587472147,0.));
#17619=CARTESIAN_POINT('Ctrl Pts',(14.9390408507356,12.8816587472147,21.));
#17620=CARTESIAN_POINT('Ctrl Pts',(14.8945191569251,12.8624032236317,0.));
#17621=CARTESIAN_POINT('Ctrl Pts',(14.8945191569251,12.8624032236317,21.));
#17622=CARTESIAN_POINT('Ctrl Pts',(14.8502347891476,12.8428057266944,0.));
#17623=CARTESIAN_POINT('Ctrl Pts',(14.8502347891476,12.8428057266944,21.));
#17624=CARTESIAN_POINT('Ctrl Pts',(14.8061758577898,12.8228846016791,0.));
#17625=CARTESIAN_POINT('Ctrl Pts',(14.8061758577898,12.8228846016791,21.));
#17626=CARTESIAN_POINT('Ctrl Pts',(14.7623324139791,12.8026557145457,0.));
#17627=CARTESIAN_POINT('Ctrl Pts',(14.7623324139791,12.8026557145457,21.));
#17628=CARTESIAN_POINT('Ctrl Pts',(14.7187037124277,12.7821227233337,0.));
#17629=CARTESIAN_POINT('Ctrl Pts',(14.7187037124277,12.7821227233337,21.));
#17630=CARTESIAN_POINT('Ctrl Pts',(14.6753044633399,12.7612687078867,0.));
#17631=CARTESIAN_POINT('Ctrl Pts',(14.6753044633399,12.7612687078867,21.));
#17632=CARTESIAN_POINT('Ctrl Pts',(14.6321748083434,12.7400427996251,0.));
#17633=CARTESIAN_POINT('Ctrl Pts',(14.6321748083434,12.7400427996251,21.));
#17634=CARTESIAN_POINT('Ctrl Pts',(14.5893698147583,12.7183743139638,0.));
#17635=CARTESIAN_POINT('Ctrl Pts',(14.5893698147583,12.7183743139638,21.));
#17636=CARTESIAN_POINT('Ctrl Pts',(14.5469417071951,12.6961966430455,0.));
#17637=CARTESIAN_POINT('Ctrl Pts',(14.5469417071951,12.6961966430455,21.));
#17638=CARTESIAN_POINT('Ctrl Pts',(14.5049233087958,12.6734695081852,0.));
#17639=CARTESIAN_POINT('Ctrl Pts',(14.5049233087958,12.6734695081852,21.));
#17640=CARTESIAN_POINT('Ctrl Pts',(14.463313553928,12.6501984687124,0.));
#17641=CARTESIAN_POINT('Ctrl Pts',(14.463313553928,12.6501984687124,21.));
#17642=CARTESIAN_POINT('Ctrl Pts',(14.4220553460485,12.626464614311,0.));
#17643=CARTESIAN_POINT('Ctrl Pts',(14.4220553460485,12.626464614311,21.));
#17644=CARTESIAN_POINT('Ctrl Pts',(14.3810669346235,12.6023830189244,0.));
#17645=CARTESIAN_POINT('Ctrl Pts',(14.3810669346235,12.6023830189244,21.));
#17646=CARTESIAN_POINT('Ctrl Pts',(14.3402859058353,12.5780443898087,0.));
#17647=CARTESIAN_POINT('Ctrl Pts',(14.3402859058353,12.5780443898087,21.));
#17648=CARTESIAN_POINT('Ctrl Pts',(14.2997103098726,12.5534605602317,0.));
#17649=CARTESIAN_POINT('Ctrl Pts',(14.2997103098726,12.5534605602317,21.));
#17650=CARTESIAN_POINT('Ctrl Pts',(14.2594378207584,12.5285125321527,0.));
#17651=CARTESIAN_POINT('Ctrl Pts',(14.2594378207584,12.5285125321527,21.));
#17652=CARTESIAN_POINT('Ctrl Pts',(14.2197144660135,12.502885965175,0.));
#17653=CARTESIAN_POINT('Ctrl Pts',(14.2197144660135,12.502885965175,21.));
#17654=CARTESIAN_POINT('Ctrl Pts',(14.1808688343892,12.4761570639125,0.));
#17655=CARTESIAN_POINT('Ctrl Pts',(14.1808688343892,12.4761570639125,21.));
#17656=CARTESIAN_POINT('Ctrl Pts',(14.1507598477672,12.4535485619996,0.));
#17657=CARTESIAN_POINT('Ctrl Pts',(14.1507598477672,12.4535485619996,21.));
#17658=CARTESIAN_POINT('Ctrl Pts',(14.1288394445866,12.4357509724316,0.));
#17659=CARTESIAN_POINT('Ctrl Pts',(14.1288394445866,12.4357509724316,21.));
#17660=CARTESIAN_POINT('Ctrl Pts',(14.1145347042316,12.4234926340671,0.));
#17661=CARTESIAN_POINT('Ctrl Pts',(14.1145347042316,12.4234926340671,21.));
#17662=CARTESIAN_POINT('Ctrl Pts',(14.1074595503134,12.4172651441477,0.));
#17663=CARTESIAN_POINT('Ctrl Pts',(14.1074595503134,12.4172651441477,21.));
#17664=CARTESIAN_POINT('',(17.3811241238545,13.486901949342,0.));
#17665=CARTESIAN_POINT('Ctrl Pts',(14.1074595503134,12.4172651441477,0.));
#17666=CARTESIAN_POINT('Ctrl Pts',(14.1145347042316,12.4234926340671,0.));
#17667=CARTESIAN_POINT('Ctrl Pts',(14.1288394445866,12.4357509724316,0.));
#17668=CARTESIAN_POINT('Ctrl Pts',(14.1507598477672,12.4535485619996,0.));
#17669=CARTESIAN_POINT('Ctrl Pts',(14.1808688343892,12.4761570639125,0.));
#17670=CARTESIAN_POINT('Ctrl Pts',(14.2197144660135,12.502885965175,0.));
#17671=CARTESIAN_POINT('Ctrl Pts',(14.2594378207584,12.5285125321527,0.));
#17672=CARTESIAN_POINT('Ctrl Pts',(14.2997103098726,12.5534605602317,0.));
#17673=CARTESIAN_POINT('Ctrl Pts',(14.3402859058353,12.5780443898087,0.));
#17674=CARTESIAN_POINT('Ctrl Pts',(14.3810669346235,12.6023830189244,0.));
#17675=CARTESIAN_POINT('Ctrl Pts',(14.4220553460485,12.626464614311,0.));
#17676=CARTESIAN_POINT('Ctrl Pts',(14.463313553928,12.6501984687124,0.));
#17677=CARTESIAN_POINT('Ctrl Pts',(14.5049233087958,12.6734695081852,0.));
#17678=CARTESIAN_POINT('Ctrl Pts',(14.5469417071951,12.6961966430455,0.));
#17679=CARTESIAN_POINT('Ctrl Pts',(14.5893698147583,12.7183743139638,0.));
#17680=CARTESIAN_POINT('Ctrl Pts',(14.6321748083434,12.7400427996251,0.));
#17681=CARTESIAN_POINT('Ctrl Pts',(14.6753044633399,12.7612687078867,0.));
#17682=CARTESIAN_POINT('Ctrl Pts',(14.7187037124277,12.7821227233337,0.));
#17683=CARTESIAN_POINT('Ctrl Pts',(14.7623324139791,12.8026557145457,0.));
#17684=CARTESIAN_POINT('Ctrl Pts',(14.8061758577898,12.8228846016791,0.));
#17685=CARTESIAN_POINT('Ctrl Pts',(14.8502347891476,12.8428057266944,0.));
#17686=CARTESIAN_POINT('Ctrl Pts',(14.8945191569251,12.8624032236317,0.));
#17687=CARTESIAN_POINT('Ctrl Pts',(14.9390408507356,12.8816587472147,0.));
#17688=CARTESIAN_POINT('Ctrl Pts',(14.9838057866976,12.9005620742036,0.));
#17689=CARTESIAN_POINT('Ctrl Pts',(15.0288099208306,12.9191164383568,0.));
#17690=CARTESIAN_POINT('Ctrl Pts',(15.0740435169624,12.9373327960422,0.));
#17691=CARTESIAN_POINT('Ctrl Pts',(15.1194937003528,12.9552263908864,0.));
#17692=CARTESIAN_POINT('Ctrl Pts',(15.1651474813659,12.9728126886697,0.));
#17693=CARTESIAN_POINT('Ctrl Pts',(15.2109950816083,12.9901029059182,0.));
#17694=CARTESIAN_POINT('Ctrl Pts',(15.2570313635503,13.0071020851025,0.));
#17695=CARTESIAN_POINT('Ctrl Pts',(15.3032539741328,13.0238115816728,0.));
#17696=CARTESIAN_POINT('Ctrl Pts',(15.3496622219036,13.0402305665115,0.));
#17697=CARTESIAN_POINT('Ctrl Pts',(15.3962557545684,13.0563577967298,0.));
#17698=CARTESIAN_POINT('Ctrl Pts',(15.4430330918328,13.0721935806302,0.));
#17699=CARTESIAN_POINT('Ctrl Pts',(15.4899910401523,13.087740560189,0.));
#17700=CARTESIAN_POINT('Ctrl Pts',(15.5371254712111,13.1030026646917,0.));
#17701=CARTESIAN_POINT('Ctrl Pts',(15.5844317820184,13.1179844917497,0.));
#17702=CARTESIAN_POINT('Ctrl Pts',(15.6319054413079,13.1326905726717,0.));
#17703=CARTESIAN_POINT('Ctrl Pts',(15.6795425955901,13.147124558532,0.));
#17704=CARTESIAN_POINT('Ctrl Pts',(15.7273402954914,13.161288914421,0.));
#17705=CARTESIAN_POINT('Ctrl Pts',(15.7752961549278,13.1751853728467,0.));
#17706=CARTESIAN_POINT('Ctrl Pts',(15.8234081427091,13.1888152101588,0.));
#17707=CARTESIAN_POINT('Ctrl Pts',(15.8716743375555,13.2021795724682,0.));
#17708=CARTESIAN_POINT('Ctrl Pts',(15.9200926550954,13.2152798388134,0.));
#17709=CARTESIAN_POINT('Ctrl Pts',(15.9686607385389,13.2281177675127,0.));
#17710=CARTESIAN_POINT('Ctrl Pts',(16.0173761036734,13.240695304984,0.));
#17711=CARTESIAN_POINT('Ctrl Pts',(16.0662362238032,13.2530144750236,0.));
#17712=CARTESIAN_POINT('Ctrl Pts',(16.1152386305152,13.2650772466062,0.));
#17713=CARTESIAN_POINT('Ctrl Pts',(16.1643810242643,13.2768853909882,0.));
#17714=CARTESIAN_POINT('Ctrl Pts',(16.2136613184475,13.2884404210387,0.));
#17715=CARTESIAN_POINT('Ctrl Pts',(16.2630775678735,13.2997436744733,0.));
#17716=CARTESIAN_POINT('Ctrl Pts',(16.3126279218067,13.3107963665229,0.));
#17717=CARTESIAN_POINT('Ctrl Pts',(16.3623105703343,13.3215996524974,0.));
#17718=CARTESIAN_POINT('Ctrl Pts',(16.4121236828756,13.3321546976812,0.));
#17719=CARTESIAN_POINT('Ctrl Pts',(16.4620653818862,13.3424627129921,0.));
#17720=CARTESIAN_POINT('Ctrl Pts',(16.5121337902953,13.3525249163084,0.));
#17721=CARTESIAN_POINT('Ctrl Pts',(16.5623270636327,13.3623425108873,0.));
#17722=CARTESIAN_POINT('Ctrl Pts',(16.612643424234,13.3719166600676,0.));
#17723=CARTESIAN_POINT('Ctrl Pts',(16.6630812012276,13.381248462113,0.));
#17724=CARTESIAN_POINT('Ctrl Pts',(16.7136388432444,13.3903389370346,0.));
#17725=CARTESIAN_POINT('Ctrl Pts',(16.7643148579873,13.3991890464165,0.));
#17726=CARTESIAN_POINT('Ctrl Pts',(16.8151077630226,13.4077997088426,0.));
#17727=CARTESIAN_POINT('Ctrl Pts',(16.8660160353187,13.4161718177499,0.));
#17728=CARTESIAN_POINT('Ctrl Pts',(16.9170380509036,13.4243062623592,0.));
#17729=CARTESIAN_POINT('Ctrl Pts',(16.9681720567298,13.432203941793,0.));
#17730=CARTESIAN_POINT('Ctrl Pts',(17.0194162803447,13.4398657451291,0.));
#17731=CARTESIAN_POINT('Ctrl Pts',(17.0707690194411,13.4472925380889,0.));
#17732=CARTESIAN_POINT('Ctrl Pts',(17.1222287365697,13.4544851484583,0.));
#17733=CARTESIAN_POINT('Ctrl Pts',(17.173794155624,13.4614443545811,0.));
#17734=CARTESIAN_POINT('Ctrl Pts',(17.235798381426,13.4695161752401,0.));
#17735=CARTESIAN_POINT('Ctrl Pts',(17.287598725272,13.4759526005425,0.));
#17736=CARTESIAN_POINT('Ctrl Pts',(17.3291218739796,13.4809165957478,0.));
#17737=CARTESIAN_POINT('Ctrl Pts',(17.360310805254,13.4845355519784,0.));
#17738=CARTESIAN_POINT('Ctrl Pts',(17.3811241238545,13.4869019493419,0.));
#17739=CARTESIAN_POINT('',(17.3811241238545,13.486901949342,13.));
#17740=CARTESIAN_POINT('Ctrl Pts',(17.3811241238545,13.4869019493419,13.));
#17741=CARTESIAN_POINT('Ctrl Pts',(17.2786694026925,13.475253226354,13.));
#17742=CARTESIAN_POINT('Ctrl Pts',(17.1768129075703,13.4622625504827,13.));
#17743=CARTESIAN_POINT('Ctrl Pts',(17.0755735571126,13.4479123002588,13.));
#17744=CARTESIAN_POINT('Ctrl Pts',(16.9078155789347,13.4241333155753,13.));
#17745=CARTESIAN_POINT('Ctrl Pts',(16.7417653345045,13.3966181288102,13.));
#17746=CARTESIAN_POINT('Ctrl Pts',(16.5776745323047,13.3652244057455,13.));
#17747=CARTESIAN_POINT('Ctrl Pts',(16.4515447193844,13.3410933492578,13.));
#17748=CARTESIAN_POINT('Ctrl Pts',(16.326570616418,13.3146689208721,13.));
#17749=CARTESIAN_POINT('Ctrl Pts',(16.2028831212964,13.285866517354,13.));
#17750=CARTESIAN_POINT('Ctrl Pts',(16.06973652377,13.2548614264574,13.));
#17751=CARTESIAN_POINT('Ctrl Pts',(15.9380763875928,13.2211052775845,13.));
#17752=CARTESIAN_POINT('Ctrl Pts',(15.8081115268615,13.1844379737316,13.));
#17753=CARTESIAN_POINT('Ctrl Pts',(15.7361594415553,13.1641379560196,13.));
#17754=CARTESIAN_POINT('Ctrl Pts',(15.6647240151602,13.1429498676482,13.));
#17755=CARTESIAN_POINT('Ctrl Pts',(15.5938437133287,13.1208442205595,13.));
#17756=CARTESIAN_POINT('Ctrl Pts',(15.5255406834836,13.0995423548249,13.));
#17757=CARTESIAN_POINT('Ctrl Pts',(15.4577571790122,13.0773830006569,13.));
#17758=CARTESIAN_POINT('Ctrl Pts',(15.3905488537597,13.0543129127178,13.));
#17759=CARTESIAN_POINT('Ctrl Pts',(15.332460243202,13.0343732795132,13.));
#17760=CARTESIAN_POINT('Ctrl Pts',(15.2747993571085,13.0137559282893,13.));
#17761=CARTESIAN_POINT('Ctrl Pts',(15.2175748360866,12.9924643454807,13.));
#17762=CARTESIAN_POINT('Ctrl Pts',(15.1765073868617,12.9771843399814,13.));
#17763=CARTESIAN_POINT('Ctrl Pts',(15.1356629994431,12.9615593596241,13.));
#17764=CARTESIAN_POINT('Ctrl Pts',(15.0950681393122,12.9455599550767,13.));
#17765=CARTESIAN_POINT('Ctrl Pts',(15.0551343146459,12.929821080404,13.));
#17766=CARTESIAN_POINT('Ctrl Pts',(15.0154457680865,12.9137147527836,13.));
#17767=CARTESIAN_POINT('Ctrl Pts',(14.9760367885877,12.8972012563026,13.));
#17768=CARTESIAN_POINT('Ctrl Pts',(14.9418668884515,12.8828830848393,13.));
#17769=CARTESIAN_POINT('Ctrl Pts',(14.9079086463149,12.8682568219259,13.));
#17770=CARTESIAN_POINT('Ctrl Pts',(14.8741550421669,12.8533364078128,13.));
#17771=CARTESIAN_POINT('Ctrl Pts',(14.8435820219545,12.8398219362837,13.));
#17772=CARTESIAN_POINT('Ctrl Pts',(14.8131735645768,12.8260705986513,13.));
#17773=CARTESIAN_POINT('Ctrl Pts',(14.7829174085775,12.812102575688,13.));
#17774=CARTESIAN_POINT('Ctrl Pts',(14.757431220614,12.8003366508055,13.));
#17775=CARTESIAN_POINT('Ctrl Pts',(14.7320520617549,12.7884183711613,13.));
#17776=CARTESIAN_POINT('Ctrl Pts',(14.7067929855474,12.7763327019834,13.));
#17777=CARTESIAN_POINT('Ctrl Pts',(14.670240352911,12.7588434231993,13.));
#17778=CARTESIAN_POINT('Ctrl Pts',(14.6339396294554,12.7410029356166,13.));
#17779=CARTESIAN_POINT('Ctrl Pts',(14.5980256541895,12.7226389621465,13.));
#17780=CARTESIAN_POINT('Ctrl Pts',(14.5763250378172,12.7115427373371,13.));
#17781=CARTESIAN_POINT('Ctrl Pts',(14.5547677202271,12.70025260105,13.));
#17782=CARTESIAN_POINT('Ctrl Pts',(14.533370542915,12.6887481999834,13.));
#17783=CARTESIAN_POINT('Ctrl Pts',(14.5136363259179,12.6781379057488,13.));
#17784=CARTESIAN_POINT('Ctrl Pts',(14.4940391165059,12.6673442955906,13.));
#17785=CARTESIAN_POINT('Ctrl Pts',(14.4745649061758,12.6563881737138,13.));
#17786=CARTESIAN_POINT('Ctrl Pts',(14.4477761570948,12.6413169181978,13.));
#17787=CARTESIAN_POINT('Ctrl Pts',(14.4212156950463,12.6259439377271,13.));
#17788=CARTESIAN_POINT('Ctrl Pts',(14.3947967979234,12.6103925840948,13.));
#17789=CARTESIAN_POINT('Ctrl Pts',(14.3780361778422,12.6005265276593,13.));
#17790=CARTESIAN_POINT('Ctrl Pts',(14.3613315560818,12.5905900369939,13.));
#17791=CARTESIAN_POINT('Ctrl Pts',(14.3446791499932,12.5805908895765,13.));
#17792=CARTESIAN_POINT('Ctrl Pts',(14.3297343906419,12.5716171201957,13.));
#17793=CARTESIAN_POINT('Ctrl Pts',(14.3148312513045,12.5625934693725,13.));
#17794=CARTESIAN_POINT('Ctrl Pts',(14.2999916562562,12.5534931963385,13.));
#17795=CARTESIAN_POINT('Ctrl Pts',(14.2843922864144,12.5439269969742,13.));
#17796=CARTESIAN_POINT('Ctrl Pts',(14.2688630441931,12.5342762591635,13.));
#17797=CARTESIAN_POINT('Ctrl Pts',(14.2534670739585,12.5244602884384,13.));
#17798=CARTESIAN_POINT('Ctrl Pts',(14.2278944013234,12.508155982693,13.));
#17799=CARTESIAN_POINT('Ctrl Pts',(14.2026946288202,12.4913891918572,13.));
#17800=CARTESIAN_POINT('Ctrl Pts',(14.1782508275394,12.4736648235789,13.));
#17801=CARTESIAN_POINT('Ctrl Pts',(14.1647716456173,12.4638909761427,13.));
#17802=CARTESIAN_POINT('Ctrl Pts',(14.1515231428256,12.4538248358964,13.));
#17803=CARTESIAN_POINT('Ctrl Pts',(14.1385523183786,12.4434054354823,13.));
#17804=CARTESIAN_POINT('Ctrl Pts',(14.1280012216095,12.4349297905843,13.));
#17805=CARTESIAN_POINT('Ctrl Pts',(14.1176338182992,12.4262204477427,13.));
#17806=CARTESIAN_POINT('Ctrl Pts',(14.1074595503134,12.4172651441477,13.));
#17807=CARTESIAN_POINT('',(17.3811241238545,13.486901949342,0.));
#17808=CARTESIAN_POINT('Origin',(4.58435815896522E-12,3.33073116609659E-12,
0.));
#17809=CARTESIAN_POINT('',(18.1978687191668,12.3627494547115,0.));
#17810=CARTESIAN_POINT('Origin',(4.58435815896522E-12,3.33073116609659E-12,
0.));
#17811=CARTESIAN_POINT('',(18.1978687191668,12.3627494547115,13.));
#17812=CARTESIAN_POINT('Origin',(4.58435815896522E-12,3.33073116609659E-12,
13.));
#17813=CARTESIAN_POINT('',(18.1978687191668,12.3627494547115,0.));
#17814=CARTESIAN_POINT('Ctrl Pts',(16.1689656784104,9.57984538049455,0.));
#17815=CARTESIAN_POINT('Ctrl Pts',(16.1689656784104,9.57984538049455,21.));
#17816=CARTESIAN_POINT('Ctrl Pts',(16.1770747160769,9.58464985151482,0.));
#17817=CARTESIAN_POINT('Ctrl Pts',(16.1770747160769,9.58464985151482,21.));
#17818=CARTESIAN_POINT('Ctrl Pts',(16.1931534965272,9.59446643316596,0.));
#17819=CARTESIAN_POINT('Ctrl Pts',(16.1931534965272,9.59446643316596,21.));
#17820=CARTESIAN_POINT('Ctrl Pts',(16.2168537871666,9.60981421781524,0.));
#17821=CARTESIAN_POINT('Ctrl Pts',(16.2168537871666,9.60981421781524,21.));
#17822=CARTESIAN_POINT('Ctrl Pts',(16.2476599387841,9.63146315443273,0.));
#17823=CARTESIAN_POINT('Ctrl Pts',(16.2476599387841,9.63146315443273,21.));
#17824=CARTESIAN_POINT('Ctrl Pts',(16.2850845948324,9.66014786078746,0.));
#17825=CARTESIAN_POINT('Ctrl Pts',(16.2850845948324,9.66014786078746,21.));
#17826=CARTESIAN_POINT('Ctrl Pts',(16.3217321000366,9.69000797146315,0.));
#17827=CARTESIAN_POINT('Ctrl Pts',(16.3217321000366,9.69000797146315,21.));
#17828=CARTESIAN_POINT('Ctrl Pts',(16.3579039682519,9.72060002001012,0.));
#17829=CARTESIAN_POINT('Ctrl Pts',(16.3579039682519,9.72060002001012,21.));
#17830=CARTESIAN_POINT('Ctrl Pts',(16.3938231282759,9.75159288382684,0.));
#17831=CARTESIAN_POINT('Ctrl Pts',(16.3938231282759,9.75159288382684,21.));
#17832=CARTESIAN_POINT('Ctrl Pts',(16.4295725710378,9.78285689698057,0.));
#17833=CARTESIAN_POINT('Ctrl Pts',(16.4295725710378,9.78285689698057,21.));
#17834=CARTESIAN_POINT('Ctrl Pts',(16.4651416449558,9.81439757053278,0.));
#17835=CARTESIAN_POINT('Ctrl Pts',(16.4651416449558,9.81439757053278,21.));
#17836=CARTESIAN_POINT('Ctrl Pts',(16.5004633692332,9.84630229363521,0.));
#17837=CARTESIAN_POINT('Ctrl Pts',(16.5004633692332,9.84630229363521,21.));
#17838=CARTESIAN_POINT('Ctrl Pts',(16.5354535643506,9.8786843754698,0.));
#17839=CARTESIAN_POINT('Ctrl Pts',(16.5354535643506,9.8786843754698,21.));
#17840=CARTESIAN_POINT('Ctrl Pts',(16.5700527532381,9.91162317616648,0.));
#17841=CARTESIAN_POINT('Ctrl Pts',(16.5700527532381,9.91162317616648,21.));
#17842=CARTESIAN_POINT('Ctrl Pts',(16.6042559779574,9.9451214271291,0.));
#17843=CARTESIAN_POINT('Ctrl Pts',(16.6042559779574,9.9451214271291,21.));
#17844=CARTESIAN_POINT('Ctrl Pts',(16.6380914029057,9.97913546489641,0.));
#17845=CARTESIAN_POINT('Ctrl Pts',(16.6380914029057,9.97913546489641,21.));
#17846=CARTESIAN_POINT('Ctrl Pts',(16.6716062376277,10.0135950379525,0.));
#17847=CARTESIAN_POINT('Ctrl Pts',(16.6716062376277,10.0135950379525,21.));
#17848=CARTESIAN_POINT('Ctrl Pts',(16.7048506904207,10.0484259314257,0.));
#17849=CARTESIAN_POINT('Ctrl Pts',(16.7048506904207,10.0484259314257,21.));
#17850=CARTESIAN_POINT('Ctrl Pts',(16.7378607357337,10.0835742491038,0.));
#17851=CARTESIAN_POINT('Ctrl Pts',(16.7378607357337,10.0835742491038,21.));
#17852=CARTESIAN_POINT('Ctrl Pts',(16.7706479198888,10.1190207721353,0.));
#17853=CARTESIAN_POINT('Ctrl Pts',(16.7706479198888,10.1190207721353,21.));
#17854=CARTESIAN_POINT('Ctrl Pts',(16.8032089941901,10.1547673397274,0.));
#17855=CARTESIAN_POINT('Ctrl Pts',(16.8032089941901,10.1547673397274,21.));
#17856=CARTESIAN_POINT('Ctrl Pts',(16.8355319435838,10.1908283166713,0.));
#17857=CARTESIAN_POINT('Ctrl Pts',(16.8355319435838,10.1908283166713,21.));
#17858=CARTESIAN_POINT('Ctrl Pts',(16.8676029947679,10.2272206796636,0.));
#17859=CARTESIAN_POINT('Ctrl Pts',(16.8676029947679,10.2272206796636,21.));
#17860=CARTESIAN_POINT('Ctrl Pts',(16.8994142530447,10.2639532144219,0.));
#17861=CARTESIAN_POINT('Ctrl Pts',(16.8994142530447,10.2639532144219,21.));
#17862=CARTESIAN_POINT('Ctrl Pts',(16.9309675442426,10.3010210756062,0.));
#17863=CARTESIAN_POINT('Ctrl Pts',(16.9309675442426,10.3010210756062,21.));
#17864=CARTESIAN_POINT('Ctrl Pts',(16.9622702798438,10.3384116178624,0.));
#17865=CARTESIAN_POINT('Ctrl Pts',(16.9622702798438,10.3384116178624,21.));
#17866=CARTESIAN_POINT('Ctrl Pts',(16.9933329788855,10.3761078860454,0.));
#17867=CARTESIAN_POINT('Ctrl Pts',(16.9933329788855,10.3761078860454,21.));
#17868=CARTESIAN_POINT('Ctrl Pts',(17.0241663361802,10.4140927470882,0.));
#17869=CARTESIAN_POINT('Ctrl Pts',(17.0241663361802,10.4140927470882,21.));
#17870=CARTESIAN_POINT('Ctrl Pts',(17.0547779975888,10.452353435089,0.));
#17871=CARTESIAN_POINT('Ctrl Pts',(17.0547779975888,10.452353435089,21.));
#17872=CARTESIAN_POINT('Ctrl Pts',(17.0851711712016,10.4908835057575,0.));
#17873=CARTESIAN_POINT('Ctrl Pts',(17.0851711712016,10.4908835057575,21.));
#17874=CARTESIAN_POINT('Ctrl Pts',(17.1153464189932,10.5296803023445,0.));
#17875=CARTESIAN_POINT('Ctrl Pts',(17.1153464189932,10.5296803023445,21.));
#17876=CARTESIAN_POINT('Ctrl Pts',(17.1453027387554,10.5687434234512,0.));
#17877=CARTESIAN_POINT('Ctrl Pts',(17.1453027387554,10.5687434234512,21.));
#17878=CARTESIAN_POINT('Ctrl Pts',(17.1750388395657,10.6080729180997,0.));
#17879=CARTESIAN_POINT('Ctrl Pts',(17.1750388395657,10.6080729180997,21.));
#17880=CARTESIAN_POINT('Ctrl Pts',(17.2045545572011,10.6476672831754,0.));
#17881=CARTESIAN_POINT('Ctrl Pts',(17.2045545572011,10.6476672831754,21.));
#17882=CARTESIAN_POINT('Ctrl Pts',(17.2338514174708,10.6875226650217,0.));
#17883=CARTESIAN_POINT('Ctrl Pts',(17.2338514174708,10.6875226650217,21.));
#17884=CARTESIAN_POINT('Ctrl Pts',(17.2629318816279,10.7276339231608,0.));
#17885=CARTESIAN_POINT('Ctrl Pts',(17.2629318816279,10.7276339231608,21.));
#17886=CARTESIAN_POINT('Ctrl Pts',(17.2917988998581,10.7679952591482,0.));
#17887=CARTESIAN_POINT('Ctrl Pts',(17.2917988998581,10.7679952591482,21.));
#17888=CARTESIAN_POINT('Ctrl Pts',(17.3204553814537,10.8086009632423,0.));
#17889=CARTESIAN_POINT('Ctrl Pts',(17.3204553814537,10.8086009632423,21.));
#17890=CARTESIAN_POINT('Ctrl Pts',(17.3489036079991,10.8494462423128,0.));
#17891=CARTESIAN_POINT('Ctrl Pts',(17.3489036079991,10.8494462423128,21.));
#17892=CARTESIAN_POINT('Ctrl Pts',(17.377145012528,10.8905275295837,0.));
#17893=CARTESIAN_POINT('Ctrl Pts',(17.377145012528,10.8905275295837,21.));
#17894=CARTESIAN_POINT('Ctrl Pts',(17.4051805054129,10.9318420203801,0.));
#17895=CARTESIAN_POINT('Ctrl Pts',(17.4051805054129,10.9318420203801,21.));
#17896=CARTESIAN_POINT('Ctrl Pts',(17.4330106728622,10.9733873885115,0.));
#17897=CARTESIAN_POINT('Ctrl Pts',(17.4330106728622,10.9733873885115,21.));
#17898=CARTESIAN_POINT('Ctrl Pts',(17.460636011184,11.0151614525642,0.));
#17899=CARTESIAN_POINT('Ctrl Pts',(17.460636011184,11.0151614525642,21.));
#17900=CARTESIAN_POINT('Ctrl Pts',(17.4880571878157,11.0571618040371,0.));
#17901=CARTESIAN_POINT('Ctrl Pts',(17.4880571878157,11.0571618040371,21.));
#17902=CARTESIAN_POINT('Ctrl Pts',(17.5152751467292,11.0993856581394,0.));
#17903=CARTESIAN_POINT('Ctrl Pts',(17.5152751467292,11.0993856581394,21.));
#17904=CARTESIAN_POINT('Ctrl Pts',(17.5422909714139,11.1418300507683,0.));
#17905=CARTESIAN_POINT('Ctrl Pts',(17.5422909714139,11.1418300507683,21.));
#17906=CARTESIAN_POINT('Ctrl Pts',(17.5691058058227,11.1844919535058,0.));
#17907=CARTESIAN_POINT('Ctrl Pts',(17.5691058058227,11.1844919535058,21.));
#17908=CARTESIAN_POINT('Ctrl Pts',(17.5957207597803,11.2273684103051,0.));
#17909=CARTESIAN_POINT('Ctrl Pts',(17.5957207597803,11.2273684103051,21.));
#17910=CARTESIAN_POINT('Ctrl Pts',(17.6221368072528,11.2704566868205,0.));
#17911=CARTESIAN_POINT('Ctrl Pts',(17.6221368072528,11.2704566868205,21.));
#17912=CARTESIAN_POINT('Ctrl Pts',(17.6483547422688,11.3137543310722,0.));
#17913=CARTESIAN_POINT('Ctrl Pts',(17.6483547422688,11.3137543310722,21.));
#17914=CARTESIAN_POINT('Ctrl Pts',(17.674375235974,11.3572590796967,0.));
#17915=CARTESIAN_POINT('Ctrl Pts',(17.674375235974,11.3572590796967,21.));
#17916=CARTESIAN_POINT('Ctrl Pts',(17.700198872213,11.4009687970126,0.));
#17917=CARTESIAN_POINT('Ctrl Pts',(17.700198872213,11.4009687970126,21.));
#17918=CARTESIAN_POINT('Ctrl Pts',(17.725826190457,11.4448814046804,0.));
#17919=CARTESIAN_POINT('Ctrl Pts',(17.725826190457,11.4448814046804,21.));
#17920=CARTESIAN_POINT('Ctrl Pts',(17.7512577332768,11.4889948016216,0.));
#17921=CARTESIAN_POINT('Ctrl Pts',(17.7512577332768,11.4889948016216,21.));
#17922=CARTESIAN_POINT('Ctrl Pts',(17.7764940721306,11.5333068279911,0.));
#17923=CARTESIAN_POINT('Ctrl Pts',(17.7764940721306,11.5333068279911,21.));
#17924=CARTESIAN_POINT('Ctrl Pts',(17.8015357852426,11.5778153222435,0.));
#17925=CARTESIAN_POINT('Ctrl Pts',(17.8015357852426,11.5778153222435,21.));
#17926=CARTESIAN_POINT('Ctrl Pts',(17.8263834470057,11.6225181583564,0.));
#17927=CARTESIAN_POINT('Ctrl Pts',(17.8263834470057,11.6225181583564,21.));
#17928=CARTESIAN_POINT('Ctrl Pts',(17.8510376144926,11.6674132861792,0.));
#17929=CARTESIAN_POINT('Ctrl Pts',(17.8510376144926,11.6674132861792,21.));
#17930=CARTESIAN_POINT('Ctrl Pts',(17.8754988158862,11.7124987772363,0.));
#17931=CARTESIAN_POINT('Ctrl Pts',(17.8754988158862,11.7124987772363,21.));
#17932=CARTESIAN_POINT('Ctrl Pts',(17.8997675418752,11.7577728408871,0.));
#17933=CARTESIAN_POINT('Ctrl Pts',(17.8997675418752,11.7577728408871,21.));
#17934=CARTESIAN_POINT('Ctrl Pts',(17.9238442458356,11.8032337607271,0.));
#17935=CARTESIAN_POINT('Ctrl Pts',(17.9238442458356,11.8032337607271,21.));
#17936=CARTESIAN_POINT('Ctrl Pts',(17.9477293432951,11.8488798430201,0.));
#17937=CARTESIAN_POINT('Ctrl Pts',(17.9477293432951,11.8488798430201,21.));
#17938=CARTESIAN_POINT('Ctrl Pts',(17.9714232133203,11.8947093631895,0.));
#17939=CARTESIAN_POINT('Ctrl Pts',(17.9714232133203,11.8947093631895,21.));
#17940=CARTESIAN_POINT('Ctrl Pts',(17.9949261997754,11.9407205019619,0.));
#17941=CARTESIAN_POINT('Ctrl Pts',(17.9949261997754,11.9407205019619,21.));
#17942=CARTESIAN_POINT('Ctrl Pts',(18.0182386160553,11.986911314246,0.));
#17943=CARTESIAN_POINT('Ctrl Pts',(18.0182386160553,11.986911314246,21.));
#17944=CARTESIAN_POINT('Ctrl Pts',(18.0413607600052,12.0332798395991,0.));
#17945=CARTESIAN_POINT('Ctrl Pts',(18.0413607600052,12.0332798395991,21.));
#17946=CARTESIAN_POINT('Ctrl Pts',(18.0642929289333,12.0798241915081,0.));
#17947=CARTESIAN_POINT('Ctrl Pts',(18.0642929289333,12.0798241915081,21.));
#17948=CARTESIAN_POINT('Ctrl Pts',(18.0870354350128,12.1265426519718,0.));
#17949=CARTESIAN_POINT('Ctrl Pts',(18.0870354350128,12.1265426519718,21.));
#17950=CARTESIAN_POINT('Ctrl Pts',(18.109588624154,12.1734337668195,0.));
#17951=CARTESIAN_POINT('Ctrl Pts',(18.109588624154,12.1734337668195,21.));
#17952=CARTESIAN_POINT('Ctrl Pts',(18.1319528884305,12.2204964278426,0.));
#17953=CARTESIAN_POINT('Ctrl Pts',(18.1319528884305,12.2204964278426,21.));
#17954=CARTESIAN_POINT('Ctrl Pts',(18.1541286139166,12.2677298318549,0.));
#17955=CARTESIAN_POINT('Ctrl Pts',(18.1541286139166,12.2677298318549,21.));
#17956=CARTESIAN_POINT('Ctrl Pts',(18.1717186310224,12.3056527265146,0.));
#17957=CARTESIAN_POINT('Ctrl Pts',(18.1717186310224,12.3056527265146,21.));
#17958=CARTESIAN_POINT('Ctrl Pts',(18.1848265584754,12.3341713636489,0.));
#17959=CARTESIAN_POINT('Ctrl Pts',(18.1848265584754,12.3341713636489,21.));
#17960=CARTESIAN_POINT('Ctrl Pts',(18.1935275957711,12.3532177620787,0.));
#17961=CARTESIAN_POINT('Ctrl Pts',(18.1935275957711,12.3532177620787,21.));
#17962=CARTESIAN_POINT('Ctrl Pts',(18.1978687191668,12.3627494547115,0.));
#17963=CARTESIAN_POINT('Ctrl Pts',(18.1978687191668,12.3627494547115,21.));
#17964=CARTESIAN_POINT('Ctrl Pts',(16.1689656784104,9.57984538049455,0.));
#17965=CARTESIAN_POINT('Ctrl Pts',(16.1770747160769,9.58464985151482,0.));
#17966=CARTESIAN_POINT('Ctrl Pts',(16.1931534965272,9.59446643316596,0.));
#17967=CARTESIAN_POINT('Ctrl Pts',(16.2168537871666,9.60981421781524,0.));
#17968=CARTESIAN_POINT('Ctrl Pts',(16.2476599387841,9.63146315443273,0.));
#17969=CARTESIAN_POINT('Ctrl Pts',(16.2850845948324,9.66014786078746,0.));
#17970=CARTESIAN_POINT('Ctrl Pts',(16.3217321000366,9.69000797146315,0.));
#17971=CARTESIAN_POINT('Ctrl Pts',(16.3579039682519,9.72060002001012,0.));
#17972=CARTESIAN_POINT('Ctrl Pts',(16.3938231282759,9.75159288382684,0.));
#17973=CARTESIAN_POINT('Ctrl Pts',(16.4295725710378,9.78285689698057,0.));
#17974=CARTESIAN_POINT('Ctrl Pts',(16.4651416449558,9.81439757053278,0.));
#17975=CARTESIAN_POINT('Ctrl Pts',(16.5004633692332,9.84630229363521,0.));
#17976=CARTESIAN_POINT('Ctrl Pts',(16.5354535643506,9.8786843754698,0.));
#17977=CARTESIAN_POINT('Ctrl Pts',(16.5700527532381,9.91162317616648,0.));
#17978=CARTESIAN_POINT('Ctrl Pts',(16.6042559779574,9.9451214271291,0.));
#17979=CARTESIAN_POINT('Ctrl Pts',(16.6380914029057,9.97913546489641,0.));
#17980=CARTESIAN_POINT('Ctrl Pts',(16.6716062376277,10.0135950379525,0.));
#17981=CARTESIAN_POINT('Ctrl Pts',(16.7048506904207,10.0484259314257,0.));
#17982=CARTESIAN_POINT('Ctrl Pts',(16.7378607357337,10.0835742491038,0.));
#17983=CARTESIAN_POINT('Ctrl Pts',(16.7706479198888,10.1190207721353,0.));
#17984=CARTESIAN_POINT('Ctrl Pts',(16.8032089941901,10.1547673397274,0.));
#17985=CARTESIAN_POINT('Ctrl Pts',(16.8355319435838,10.1908283166713,0.));
#17986=CARTESIAN_POINT('Ctrl Pts',(16.8676029947679,10.2272206796636,0.));
#17987=CARTESIAN_POINT('Ctrl Pts',(16.8994142530447,10.2639532144219,0.));
#17988=CARTESIAN_POINT('Ctrl Pts',(16.9309675442426,10.3010210756062,0.));
#17989=CARTESIAN_POINT('Ctrl Pts',(16.9622702798438,10.3384116178624,0.));
#17990=CARTESIAN_POINT('Ctrl Pts',(16.9933329788855,10.3761078860454,0.));
#17991=CARTESIAN_POINT('Ctrl Pts',(17.0241663361802,10.4140927470882,0.));
#17992=CARTESIAN_POINT('Ctrl Pts',(17.0547779975888,10.452353435089,0.));
#17993=CARTESIAN_POINT('Ctrl Pts',(17.0851711712016,10.4908835057575,0.));
#17994=CARTESIAN_POINT('Ctrl Pts',(17.1153464189932,10.5296803023445,0.));
#17995=CARTESIAN_POINT('Ctrl Pts',(17.1453027387554,10.5687434234512,0.));
#17996=CARTESIAN_POINT('Ctrl Pts',(17.1750388395657,10.6080729180997,0.));
#17997=CARTESIAN_POINT('Ctrl Pts',(17.2045545572011,10.6476672831754,0.));
#17998=CARTESIAN_POINT('Ctrl Pts',(17.2338514174708,10.6875226650217,0.));
#17999=CARTESIAN_POINT('Ctrl Pts',(17.2629318816279,10.7276339231608,0.));
#18000=CARTESIAN_POINT('Ctrl Pts',(17.2917988998581,10.7679952591482,0.));
#18001=CARTESIAN_POINT('Ctrl Pts',(17.3204553814537,10.8086009632423,0.));
#18002=CARTESIAN_POINT('Ctrl Pts',(17.3489036079991,10.8494462423128,0.));
#18003=CARTESIAN_POINT('Ctrl Pts',(17.377145012528,10.8905275295837,0.));
#18004=CARTESIAN_POINT('Ctrl Pts',(17.4051805054129,10.9318420203801,0.));
#18005=CARTESIAN_POINT('Ctrl Pts',(17.4330106728622,10.9733873885115,0.));
#18006=CARTESIAN_POINT('Ctrl Pts',(17.460636011184,11.0151614525642,0.));
#18007=CARTESIAN_POINT('Ctrl Pts',(17.4880571878157,11.0571618040371,0.));
#18008=CARTESIAN_POINT('Ctrl Pts',(17.5152751467292,11.0993856581394,0.));
#18009=CARTESIAN_POINT('Ctrl Pts',(17.5422909714139,11.1418300507683,0.));
#18010=CARTESIAN_POINT('Ctrl Pts',(17.5691058058227,11.1844919535058,0.));
#18011=CARTESIAN_POINT('Ctrl Pts',(17.5957207597803,11.2273684103051,0.));
#18012=CARTESIAN_POINT('Ctrl Pts',(17.6221368072528,11.2704566868205,0.));
#18013=CARTESIAN_POINT('Ctrl Pts',(17.6483547422688,11.3137543310722,0.));
#18014=CARTESIAN_POINT('Ctrl Pts',(17.674375235974,11.3572590796967,0.));
#18015=CARTESIAN_POINT('Ctrl Pts',(17.700198872213,11.4009687970126,0.));
#18016=CARTESIAN_POINT('Ctrl Pts',(17.725826190457,11.4448814046804,0.));
#18017=CARTESIAN_POINT('Ctrl Pts',(17.7512577332768,11.4889948016216,0.));
#18018=CARTESIAN_POINT('Ctrl Pts',(17.7764940721306,11.5333068279911,0.));
#18019=CARTESIAN_POINT('Ctrl Pts',(17.8015357852426,11.5778153222435,0.));
#18020=CARTESIAN_POINT('Ctrl Pts',(17.8263834470057,11.6225181583564,0.));
#18021=CARTESIAN_POINT('Ctrl Pts',(17.8510376144926,11.6674132861792,0.));
#18022=CARTESIAN_POINT('Ctrl Pts',(17.8754988158862,11.7124987772363,0.));
#18023=CARTESIAN_POINT('Ctrl Pts',(17.8997675418752,11.7577728408871,0.));
#18024=CARTESIAN_POINT('Ctrl Pts',(17.9238442458356,11.8032337607271,0.));
#18025=CARTESIAN_POINT('Ctrl Pts',(17.9477293432951,11.8488798430201,0.));
#18026=CARTESIAN_POINT('Ctrl Pts',(17.9714232133203,11.8947093631895,0.));
#18027=CARTESIAN_POINT('Ctrl Pts',(17.9949261997754,11.9407205019619,0.));
#18028=CARTESIAN_POINT('Ctrl Pts',(18.0182386160553,11.986911314246,0.));
#18029=CARTESIAN_POINT('Ctrl Pts',(18.0413607600052,12.0332798395991,0.));
#18030=CARTESIAN_POINT('Ctrl Pts',(18.0642929289333,12.0798241915081,0.));
#18031=CARTESIAN_POINT('Ctrl Pts',(18.0870354350128,12.1265426519718,0.));
#18032=CARTESIAN_POINT('Ctrl Pts',(18.109588624154,12.1734337668195,0.));
#18033=CARTESIAN_POINT('Ctrl Pts',(18.1364257412858,12.2299089600472,0.));
#18034=CARTESIAN_POINT('Ctrl Pts',(18.1585543320743,12.2771850498068,0.));
#18035=CARTESIAN_POINT('Ctrl Pts',(18.1761067306718,12.3151419520839,0.));
#18036=CARTESIAN_POINT('Ctrl Pts',(18.1891864723772,12.3436860694314,0.));
#18037=CARTESIAN_POINT('Ctrl Pts',(18.1978687191668,12.3627494547115,0.));
#18038=CARTESIAN_POINT('Ctrl Pts',(16.1689656784104,9.57984538049455,13.));
#18039=CARTESIAN_POINT('Ctrl Pts',(16.1826331205334,9.58794311444298,13.));
#18040=CARTESIAN_POINT('Ctrl Pts',(16.1960605405031,9.59639855902712,13.));
#18041=CARTESIAN_POINT('Ctrl Pts',(16.209264165571,9.60518801711085,13.));
#18042=CARTESIAN_POINT('Ctrl Pts',(16.224739801703,9.6154899193841,13.));
#18043=CARTESIAN_POINT('Ctrl Pts',(16.2399084848584,9.62624998107167,13.));
#18044=CARTESIAN_POINT('Ctrl Pts',(16.254836637175,9.63737105568732,13.));
#18045=CARTESIAN_POINT('Ctrl Pts',(16.2758412618972,9.65301893989003,13.));
#18046=CARTESIAN_POINT('Ctrl Pts',(16.296373798599,9.66937567449949,13.));
#18047=CARTESIAN_POINT('Ctrl Pts',(16.3166650331518,9.68610238201322,13.));
#18048=CARTESIAN_POINT('Ctrl Pts',(16.3301619042985,9.69722828051063,13.));
#18049=CARTESIAN_POINT('Ctrl Pts',(16.3435531467518,9.70851618070807,13.));
#18050=CARTESIAN_POINT('Ctrl Pts',(16.3568892752788,9.7198910779208,13.));
#18051=CARTESIAN_POINT('Ctrl Pts',(16.3709277366574,9.73186502184932,13.));
#18052=CARTESIAN_POINT('Ctrl Pts',(16.3849056240572,9.74393463776872,13.));
#18053=CARTESIAN_POINT('Ctrl Pts',(16.3988451548219,9.75606525513648,13.));
#18054=CARTESIAN_POINT('Ctrl Pts',(16.414325766791,9.76953696975778,13.));
#18055=CARTESIAN_POINT('Ctrl Pts',(16.4297583183324,9.78308498747417,13.));
#18056=CARTESIAN_POINT('Ctrl Pts',(16.4451338763398,9.79671869019648,13.));
#18057=CARTESIAN_POINT('Ctrl Pts',(16.4683132763075,9.8172721587789,13.));
#18058=CARTESIAN_POINT('Ctrl Pts',(16.4913594464712,9.83802550134249,13.));
#18059=CARTESIAN_POINT('Ctrl Pts',(16.5141788054336,9.8591036086492,13.));
#18060=CARTESIAN_POINT('Ctrl Pts',(16.5307565708362,9.87441639279171,13.));
#18061=CARTESIAN_POINT('Ctrl Pts',(16.5472127770975,9.88990330206224,13.));
#18062=CARTESIAN_POINT('Ctrl Pts',(16.5635345032205,9.90558047214324,13.));
#18063=CARTESIAN_POINT('Ctrl Pts',(16.5834864158081,9.92474447016174,13.));
#18064=CARTESIAN_POINT('Ctrl Pts',(16.6032381063718,9.94419173110009,13.));
#18065=CARTESIAN_POINT('Ctrl Pts',(16.6228156007807,9.96388214930655,13.));
#18066=CARTESIAN_POINT('Ctrl Pts',(16.6439625439398,9.9851510689085,13.));
#18067=CARTESIAN_POINT('Ctrl Pts',(16.6649096998191,10.006698815053,13.));
#18068=CARTESIAN_POINT('Ctrl Pts',(16.6857083247995,10.0284493480904,13.));
#18069=CARTESIAN_POINT('Ctrl Pts',(16.7049095176705,10.0485293380076,13.));
#18070=CARTESIAN_POINT('Ctrl Pts',(16.7239855768682,10.0687801145851,13.));
#18071=CARTESIAN_POINT('Ctrl Pts',(16.7429517500628,10.0891775910162,13.));
#18072=CARTESIAN_POINT('Ctrl Pts',(16.7687182701337,10.1168886100216,13.));
#18073=CARTESIAN_POINT('Ctrl Pts',(16.7942808297111,10.1448719871919,13.));
#18074=CARTESIAN_POINT('Ctrl Pts',(16.8196194580035,10.1731502199822,13.));
#18075=CARTESIAN_POINT('Ctrl Pts',(16.8440706870575,10.200438103889,13.));
#18076=CARTESIAN_POINT('Ctrl Pts',(16.8683088890845,10.22800693093,13.));
#18077=CARTESIAN_POINT('Ctrl Pts',(16.8923226175348,10.2558682820695,13.));
#18078=CARTESIAN_POINT('Ctrl Pts',(16.9249459403077,10.2937187080453,13.));
#18079=CARTESIAN_POINT('Ctrl Pts',(16.957156835636,10.3321063567987,13.));
#18080=CARTESIAN_POINT('Ctrl Pts',(16.9889999235631,10.3709578724441,13.));
#18081=CARTESIAN_POINT('Ctrl Pts',(17.0169893056038,10.4051075100907,13.));
#18082=CARTESIAN_POINT('Ctrl Pts',(17.0446984863548,10.4396099589581,13.));
#18083=CARTESIAN_POINT('Ctrl Pts',(17.0721430002005,10.4744368762492,13.));
#18084=CARTESIAN_POINT('Ctrl Pts',(17.112602877038,10.5257802081858,13.));
#18085=CARTESIAN_POINT('Ctrl Pts',(17.1524822680213,10.5778361036166,13.));
#18086=CARTESIAN_POINT('Ctrl Pts',(17.1917748564439,10.6305946314109,13.));
#18087=CARTESIAN_POINT('Ctrl Pts',(17.2413624862159,10.6971764079904,13.));
#18088=CARTESIAN_POINT('Ctrl Pts',(17.2900185097256,10.7648729796203,13.));
#18089=CARTESIAN_POINT('Ctrl Pts',(17.3377983049414,10.8335716332062,13.));
#18090=CARTESIAN_POINT('Ctrl Pts',(17.4025197210759,10.9266292557124,13.));
#18091=CARTESIAN_POINT('Ctrl Pts',(17.465629946413,11.0215303642373,13.));
#18092=CARTESIAN_POINT('Ctrl Pts',(17.5271690583425,11.1181400554142,13.));
#18093=CARTESIAN_POINT('Ctrl Pts',(17.5820327884924,11.2042701255502,13.));
#18094=CARTESIAN_POINT('Ctrl Pts',(17.6356526662298,11.2917512652669,13.));
#18095=CARTESIAN_POINT('Ctrl Pts',(17.6880597469793,11.3804891386312,13.));
#18096=CARTESIAN_POINT('Ctrl Pts',(17.7623349917745,11.5062551071316,13.));
#18097=CARTESIAN_POINT('Ctrl Pts',(17.8341701535693,11.6345494475267,13.));
#18098=CARTESIAN_POINT('Ctrl Pts',(17.9036238122721,11.7651542351076,13.));
#18099=CARTESIAN_POINT('Ctrl Pts',(17.9575737615817,11.8666049261321,13.));
#18100=CARTESIAN_POINT('Ctrl Pts',(18.0100864746848,11.9694546915729,13.));
#18101=CARTESIAN_POINT('Ctrl Pts',(18.0611784501166,12.0736101882024,13.));
#18102=CARTESIAN_POINT('Ctrl Pts',(18.105376864951,12.1637125537578,13.));
#18103=CARTESIAN_POINT('Ctrl Pts',(18.148512095574,12.2547877896022,13.));
#18104=CARTESIAN_POINT('Ctrl Pts',(18.1905949538311,12.3468112455713,13.));
#18105=CARTESIAN_POINT('Ctrl Pts',(18.193023049118,12.3521208117218,13.));
#18106=CARTESIAN_POINT('Ctrl Pts',(18.1954476374996,12.3574335481621,13.));
#18107=CARTESIAN_POINT('Ctrl Pts',(18.1978687191668,12.3627494547115,13.));
#18108=CARTESIAN_POINT('Ctrl Pts',(20.698113262342,7.45574324794401,0.));
#18109=CARTESIAN_POINT('Ctrl Pts',(20.698113262342,7.45574324794401,21.));
#18110=CARTESIAN_POINT('Ctrl Pts',(20.6878503127065,7.45783379370107,0.));
#18111=CARTESIAN_POINT('Ctrl Pts',(20.6878503127065,7.45783379370107,21.));
#18112=CARTESIAN_POINT('Ctrl Pts',(20.6673271112931,7.46198969876653,0.));
#18113=CARTESIAN_POINT('Ctrl Pts',(20.6673271112931,7.46198969876653,21.));
#18114=CARTESIAN_POINT('Ctrl Pts',(20.6365504027501,7.46814799701905,0.));
#18115=CARTESIAN_POINT('Ctrl Pts',(20.6365504027501,7.46814799701905,21.));
#18116=CARTESIAN_POINT('Ctrl Pts',(20.5955309838521,7.47620789245428,0.));
#18117=CARTESIAN_POINT('Ctrl Pts',(20.5955309838521,7.47620789245428,21.));
#18118=CARTESIAN_POINT('Ctrl Pts',(20.5442837929044,7.48603045196744,0.));
#18119=CARTESIAN_POINT('Ctrl Pts',(20.5442837929044,7.48603045196744,21.));
#18120=CARTESIAN_POINT('Ctrl Pts',(20.4930639156161,7.49560012018405,0.));
#18121=CARTESIAN_POINT('Ctrl Pts',(20.4930639156161,7.49560012018405,21.));
#18122=CARTESIAN_POINT('Ctrl Pts',(20.4418717748497,7.50491611266253,0.));
#18123=CARTESIAN_POINT('Ctrl Pts',(20.4418717748497,7.50491611266253,21.));
#18124=CARTESIAN_POINT('Ctrl Pts',(20.3907080367098,7.51397746081993,0.));
#18125=CARTESIAN_POINT('Ctrl Pts',(20.3907080367098,7.51397746081993,21.));
#18126=CARTESIAN_POINT('Ctrl Pts',(20.3395736743243,7.52278303006887,0.));
#18127=CARTESIAN_POINT('Ctrl Pts',(20.3395736743243,7.52278303006887,21.));
#18128=CARTESIAN_POINT('Ctrl Pts',(20.2884698940944,7.53133155804008,0.));
#18129=CARTESIAN_POINT('Ctrl Pts',(20.2884698940944,7.53133155804008,21.));
#18130=CARTESIAN_POINT('Ctrl Pts',(20.2373980474879,7.53962169534167,0.));
#18131=CARTESIAN_POINT('Ctrl Pts',(20.2373980474879,7.53962169534167,21.));
#18132=CARTESIAN_POINT('Ctrl Pts',(20.1863595454674,7.54765204869254,0.));
#18133=CARTESIAN_POINT('Ctrl Pts',(20.1863595454674,7.54765204869254,21.));
#18134=CARTESIAN_POINT('Ctrl Pts',(20.1353557774357,7.55542122125494,0.));
#18135=CARTESIAN_POINT('Ctrl Pts',(20.1353557774357,7.55542122125494,21.));
#18136=CARTESIAN_POINT('Ctrl Pts',(20.0843880130978,7.5629278654946,0.));
#18137=CARTESIAN_POINT('Ctrl Pts',(20.0843880130978,7.5629278654946,21.));
#18138=CARTESIAN_POINT('Ctrl Pts',(20.0334574248556,7.57017066105973,0.));
#18139=CARTESIAN_POINT('Ctrl Pts',(20.0334574248556,7.57017066105973,21.));
#18140=CARTESIAN_POINT('Ctrl Pts',(19.9825651387294,7.57714827622806,0.));
#18141=CARTESIAN_POINT('Ctrl Pts',(19.9825651387294,7.57714827622806,21.));
#18142=CARTESIAN_POINT('Ctrl Pts',(19.931712276832,7.58385933533351,0.));
#18143=CARTESIAN_POINT('Ctrl Pts',(19.931712276832,7.58385933533351,21.));
#18144=CARTESIAN_POINT('Ctrl Pts',(19.8808999994024,7.59030238888852,0.));
#18145=CARTESIAN_POINT('Ctrl Pts',(19.8808999994024,7.59030238888852,21.));
#18146=CARTESIAN_POINT('Ctrl Pts',(19.830129556152,7.59647587605448,0.));
#18147=CARTESIAN_POINT('Ctrl Pts',(19.830129556152,7.59647587605448,21.));
#18148=CARTESIAN_POINT('Ctrl Pts',(19.7794022782484,7.60237814110186,0.));
#18149=CARTESIAN_POINT('Ctrl Pts',(19.7794022782484,7.60237814110186,21.));
#18150=CARTESIAN_POINT('Ctrl Pts',(19.7287195480601,7.60800746969261,0.));
#18151=CARTESIAN_POINT('Ctrl Pts',(19.7287195480601,7.60800746969261,21.));
#18152=CARTESIAN_POINT('Ctrl Pts',(19.6780827744426,7.61336212350879,0.));
#18153=CARTESIAN_POINT('Ctrl Pts',(19.6780827744426,7.61336212350879,21.));
#18154=CARTESIAN_POINT('Ctrl Pts',(19.6274933688524,7.6184403707059,0.));
#18155=CARTESIAN_POINT('Ctrl Pts',(19.6274933688524,7.6184403707059,21.));
#18156=CARTESIAN_POINT('Ctrl Pts',(19.5769527121826,7.62324053735219,0.));
#18157=CARTESIAN_POINT('Ctrl Pts',(19.5769527121826,7.62324053735219,21.));
#18158=CARTESIAN_POINT('Ctrl Pts',(19.5264621687521,7.62776096538883,0.));
#18159=CARTESIAN_POINT('Ctrl Pts',(19.5264621687521,7.62776096538883,21.));
#18160=CARTESIAN_POINT('Ctrl Pts',(19.4760231231881,7.63199992715365,0.));
#18161=CARTESIAN_POINT('Ctrl Pts',(19.4760231231881,7.63199992715365,21.));
#18162=CARTESIAN_POINT('Ctrl Pts',(19.4256370121006,7.63595554930654,0.));
#18163=CARTESIAN_POINT('Ctrl Pts',(19.4256370121006,7.63595554930654,21.));
#18164=CARTESIAN_POINT('Ctrl Pts',(19.3753053524647,7.6396257482276,0.));
#18165=CARTESIAN_POINT('Ctrl Pts',(19.3753053524647,7.6396257482276,21.));
#18166=CARTESIAN_POINT('Ctrl Pts',(19.3250297839295,7.64300812875339,0.));
#18167=CARTESIAN_POINT('Ctrl Pts',(19.3250297839295,7.64300812875339,21.));
#18168=CARTESIAN_POINT('Ctrl Pts',(19.2748120456486,7.64610005549613,0.));
#18169=CARTESIAN_POINT('Ctrl Pts',(19.2748120456486,7.64610005549613,21.));
#18170=CARTESIAN_POINT('Ctrl Pts',(19.224653915265,7.64889882291923,0.));
#18171=CARTESIAN_POINT('Ctrl Pts',(19.224653915265,7.64889882291923,21.));
#18172=CARTESIAN_POINT('Ctrl Pts',(19.1745571539291,7.65140181220525,0.));
#18173=CARTESIAN_POINT('Ctrl Pts',(19.1745571539291,7.65140181220525,21.));
#18174=CARTESIAN_POINT('Ctrl Pts',(19.1245234597312,7.65360662280609,0.));
#18175=CARTESIAN_POINT('Ctrl Pts',(19.1245234597312,7.65360662280609,21.));
#18176=CARTESIAN_POINT('Ctrl Pts',(19.0745543888799,7.65551129907201,0.));
#18177=CARTESIAN_POINT('Ctrl Pts',(19.0745543888799,7.65551129907201,21.));
#18178=CARTESIAN_POINT('Ctrl Pts',(19.0246514144531,7.65711415727855,0.));
#18179=CARTESIAN_POINT('Ctrl Pts',(19.0246514144531,7.65711415727855,21.));
#18180=CARTESIAN_POINT('Ctrl Pts',(18.974816073814,7.65841335587266,0.));
#18181=CARTESIAN_POINT('Ctrl Pts',(18.974816073814,7.65841335587266,21.));
#18182=CARTESIAN_POINT('Ctrl Pts',(18.9250501008887,7.65940650980099,0.));
#18183=CARTESIAN_POINT('Ctrl Pts',(18.9250501008887,7.65940650980099,21.));
#18184=CARTESIAN_POINT('Ctrl Pts',(18.8753555389435,7.66009036321663,0.));
#18185=CARTESIAN_POINT('Ctrl Pts',(18.8753555389435,7.66009036321663,21.));
#18186=CARTESIAN_POINT('Ctrl Pts',(18.8257349246207,7.66046025294775,0.));
#18187=CARTESIAN_POINT('Ctrl Pts',(18.8257349246207,7.66046025294775,21.));
#18188=CARTESIAN_POINT('Ctrl Pts',(18.7761911671591,7.6605104692254,0.));
#18189=CARTESIAN_POINT('Ctrl Pts',(18.7761911671591,7.6605104692254,21.));
#18190=CARTESIAN_POINT('Ctrl Pts',(18.7267272235231,7.66023521705904,0.));
#18191=CARTESIAN_POINT('Ctrl Pts',(18.7267272235231,7.66023521705904,21.));
#18192=CARTESIAN_POINT('Ctrl Pts',(18.6773458057584,7.65962948375621,0.));
#18193=CARTESIAN_POINT('Ctrl Pts',(18.6773458057584,7.65962948375621,21.));
#18194=CARTESIAN_POINT('Ctrl Pts',(18.6280491346907,7.65868976978872,0.));
#18195=CARTESIAN_POINT('Ctrl Pts',(18.6280491346907,7.65868976978872,21.));
#18196=CARTESIAN_POINT('Ctrl Pts',(18.5788385228928,7.65741532450727,0.));
#18197=CARTESIAN_POINT('Ctrl Pts',(18.5788385228928,7.65741532450727,21.));
#18198=CARTESIAN_POINT('Ctrl Pts',(18.5297146894905,7.65580722110437,0.));
#18199=CARTESIAN_POINT('Ctrl Pts',(18.5297146894905,7.65580722110437,21.));
#18200=CARTESIAN_POINT('Ctrl Pts',(18.4806785483052,7.65386603444743,0.));
#18201=CARTESIAN_POINT('Ctrl Pts',(18.4806785483052,7.65386603444743,21.));
#18202=CARTESIAN_POINT('Ctrl Pts',(18.4317319183719,7.65158974829126,0.));
#18203=CARTESIAN_POINT('Ctrl Pts',(18.4317319183719,7.65158974829126,21.));
#18204=CARTESIAN_POINT('Ctrl Pts',(18.3828781275628,7.6489719793775,0.));
#18205=CARTESIAN_POINT('Ctrl Pts',(18.3828781275628,7.6489719793775,21.));
#18206=CARTESIAN_POINT('Ctrl Pts',(18.3341230095852,7.64599903846601,0.));
#18207=CARTESIAN_POINT('Ctrl Pts',(18.3341230095852,7.64599903846601,21.));
#18208=CARTESIAN_POINT('Ctrl Pts',(18.2854741391282,7.6426522027076,0.));
#18209=CARTESIAN_POINT('Ctrl Pts',(18.2854741391282,7.6426522027076,21.));
#18210=CARTESIAN_POINT('Ctrl Pts',(18.2369390502576,7.63891299603826,0.));
#18211=CARTESIAN_POINT('Ctrl Pts',(18.2369390502576,7.63891299603826,21.));
#18212=CARTESIAN_POINT('Ctrl Pts',(18.1885236169197,7.63476798969016,0.));
#18213=CARTESIAN_POINT('Ctrl Pts',(18.1885236169197,7.63476798969016,21.));
#18214=CARTESIAN_POINT('Ctrl Pts',(18.1402306858819,7.63021285851761,0.));
#18215=CARTESIAN_POINT('Ctrl Pts',(18.1402306858819,7.63021285851761,21.));
#18216=CARTESIAN_POINT('Ctrl Pts',(18.0920577897363,7.62525915358073,0.));
#18217=CARTESIAN_POINT('Ctrl Pts',(18.0920577897363,7.62525915358073,21.));
#18218=CARTESIAN_POINT('Ctrl Pts',(18.0439992897906,7.61992799636654,0.));
#18219=CARTESIAN_POINT('Ctrl Pts',(18.0439992897906,7.61992799636654,21.));
#18220=CARTESIAN_POINT('Ctrl Pts',(17.9960506269561,7.61423755067037,0.));
#18221=CARTESIAN_POINT('Ctrl Pts',(17.9960506269561,7.61423755067037,21.));
#18222=CARTESIAN_POINT('Ctrl Pts',(17.9482122228183,7.60819152580111,0.));
#18223=CARTESIAN_POINT('Ctrl Pts',(17.9482122228183,7.60819152580111,21.));
#18224=CARTESIAN_POINT('Ctrl Pts',(17.900492838997,7.60176928403058,0.));
#18225=CARTESIAN_POINT('Ctrl Pts',(17.900492838997,7.60176928403058,21.));
#18226=CARTESIAN_POINT('Ctrl Pts',(17.8529149331931,7.59491004201955,0.));
#18227=CARTESIAN_POINT('Ctrl Pts',(17.8529149331931,7.59491004201955,21.));
#18228=CARTESIAN_POINT('Ctrl Pts',(17.8055090348024,7.58752955799499,0.));
#18229=CARTESIAN_POINT('Ctrl Pts',(17.8055090348024,7.58752955799499,21.));
#18230=CARTESIAN_POINT('Ctrl Pts',(17.7583042294209,7.57954834582803,0.));
#18231=CARTESIAN_POINT('Ctrl Pts',(17.7583042294209,7.57954834582803,21.));
#18232=CARTESIAN_POINT('Ctrl Pts',(17.7113192869136,7.57091795530423,0.));
#18233=CARTESIAN_POINT('Ctrl Pts',(17.7113192869136,7.57091795530423,21.));
#18234=CARTESIAN_POINT('Ctrl Pts',(17.6645549117314,7.56164400295863,0.));
#18235=CARTESIAN_POINT('Ctrl Pts',(17.6645549117314,7.56164400295863,21.));
#18236=CARTESIAN_POINT('Ctrl Pts',(17.6179818599248,7.55182125346563,0.));
#18237=CARTESIAN_POINT('Ctrl Pts',(17.6179818599248,7.55182125346563,21.));
#18238=CARTESIAN_POINT('Ctrl Pts',(17.5715579419204,7.54158441095317,0.));
#18239=CARTESIAN_POINT('Ctrl Pts',(17.5715579419204,7.54158441095317,21.));
#18240=CARTESIAN_POINT('Ctrl Pts',(17.5252518287336,7.53103903007863,0.));
#18241=CARTESIAN_POINT('Ctrl Pts',(17.5252518287336,7.53103903007863,21.));
#18242=CARTESIAN_POINT('Ctrl Pts',(17.4790653226646,7.52019696747328,0.));
#18243=CARTESIAN_POINT('Ctrl Pts',(17.4790653226646,7.52019696747328,21.));
#18244=CARTESIAN_POINT('Ctrl Pts',(17.4330545448126,7.50891486634214,0.));
#18245=CARTESIAN_POINT('Ctrl Pts',(17.4330545448126,7.50891486634214,21.));
#18246=CARTESIAN_POINT('Ctrl Pts',(17.3873563447297,7.49681774451751,0.));
#18247=CARTESIAN_POINT('Ctrl Pts',(17.3873563447297,7.49681774451751,21.));
#18248=CARTESIAN_POINT('Ctrl Pts',(17.3421522689127,7.48340100912745,0.));
#18249=CARTESIAN_POINT('Ctrl Pts',(17.3421522689127,7.48340100912745,21.));
#18250=CARTESIAN_POINT('Ctrl Pts',(17.3065305096784,7.47120323460919,0.));
#18251=CARTESIAN_POINT('Ctrl Pts',(17.3065305096784,7.47120323460919,21.));
#18252=CARTESIAN_POINT('Ctrl Pts',(17.2801832097582,7.4610504981825,0.));
#18253=CARTESIAN_POINT('Ctrl Pts',(17.2801832097582,7.4610504981825,21.));
#18254=CARTESIAN_POINT('Ctrl Pts',(17.2627905583523,7.45381253347183,0.));
#18255=CARTESIAN_POINT('Ctrl Pts',(17.2627905583523,7.45381253347183,21.));
#18256=CARTESIAN_POINT('Ctrl Pts',(17.2541372868972,7.45007618140238,0.));
#18257=CARTESIAN_POINT('Ctrl Pts',(17.2541372868972,7.45007618140238,21.));
#18258=CARTESIAN_POINT('',(20.698113262342,7.45574324794407,0.));
#18259=CARTESIAN_POINT('Ctrl Pts',(17.2541372868972,7.45007618140238,0.));
#18260=CARTESIAN_POINT('Ctrl Pts',(17.2627905583523,7.45381253347183,0.));
#18261=CARTESIAN_POINT('Ctrl Pts',(17.2801832097582,7.4610504981825,0.));
#18262=CARTESIAN_POINT('Ctrl Pts',(17.3065305096784,7.47120323460919,0.));
#18263=CARTESIAN_POINT('Ctrl Pts',(17.3421522689127,7.48340100912745,0.));
#18264=CARTESIAN_POINT('Ctrl Pts',(17.3873563447297,7.49681774451751,0.));
#18265=CARTESIAN_POINT('Ctrl Pts',(17.4330545448126,7.50891486634214,0.));
#18266=CARTESIAN_POINT('Ctrl Pts',(17.4790653226646,7.52019696747328,0.));
#18267=CARTESIAN_POINT('Ctrl Pts',(17.5252518287336,7.53103903007863,0.));
#18268=CARTESIAN_POINT('Ctrl Pts',(17.5715579419204,7.54158441095317,0.));
#18269=CARTESIAN_POINT('Ctrl Pts',(17.6179818599248,7.55182125346563,0.));
#18270=CARTESIAN_POINT('Ctrl Pts',(17.6645549117314,7.56164400295863,0.));
#18271=CARTESIAN_POINT('Ctrl Pts',(17.7113192869136,7.57091795530423,0.));
#18272=CARTESIAN_POINT('Ctrl Pts',(17.7583042294209,7.57954834582803,0.));
#18273=CARTESIAN_POINT('Ctrl Pts',(17.8055090348024,7.58752955799499,0.));
#18274=CARTESIAN_POINT('Ctrl Pts',(17.8529149331931,7.59491004201955,0.));
#18275=CARTESIAN_POINT('Ctrl Pts',(17.900492838997,7.60176928403058,0.));
#18276=CARTESIAN_POINT('Ctrl Pts',(17.9482122228183,7.60819152580111,0.));
#18277=CARTESIAN_POINT('Ctrl Pts',(17.9960506269561,7.61423755067037,0.));
#18278=CARTESIAN_POINT('Ctrl Pts',(18.0439992897906,7.61992799636654,0.));
#18279=CARTESIAN_POINT('Ctrl Pts',(18.0920577897363,7.62525915358073,0.));
#18280=CARTESIAN_POINT('Ctrl Pts',(18.1402306858819,7.63021285851761,0.));
#18281=CARTESIAN_POINT('Ctrl Pts',(18.1885236169197,7.63476798969016,0.));
#18282=CARTESIAN_POINT('Ctrl Pts',(18.2369390502576,7.63891299603826,0.));
#18283=CARTESIAN_POINT('Ctrl Pts',(18.2854741391282,7.6426522027076,0.));
#18284=CARTESIAN_POINT('Ctrl Pts',(18.3341230095852,7.64599903846601,0.));
#18285=CARTESIAN_POINT('Ctrl Pts',(18.3828781275628,7.6489719793775,0.));
#18286=CARTESIAN_POINT('Ctrl Pts',(18.4317319183719,7.65158974829126,0.));
#18287=CARTESIAN_POINT('Ctrl Pts',(18.4806785483052,7.65386603444743,0.));
#18288=CARTESIAN_POINT('Ctrl Pts',(18.5297146894905,7.65580722110437,0.));
#18289=CARTESIAN_POINT('Ctrl Pts',(18.5788385228928,7.65741532450727,0.));
#18290=CARTESIAN_POINT('Ctrl Pts',(18.6280491346907,7.65868976978872,0.));
#18291=CARTESIAN_POINT('Ctrl Pts',(18.6773458057584,7.65962948375621,0.));
#18292=CARTESIAN_POINT('Ctrl Pts',(18.7267272235231,7.66023521705904,0.));
#18293=CARTESIAN_POINT('Ctrl Pts',(18.7761911671591,7.6605104692254,0.));
#18294=CARTESIAN_POINT('Ctrl Pts',(18.8257349246207,7.66046025294775,0.));
#18295=CARTESIAN_POINT('Ctrl Pts',(18.8753555389435,7.66009036321663,0.));
#18296=CARTESIAN_POINT('Ctrl Pts',(18.9250501008887,7.65940650980099,0.));
#18297=CARTESIAN_POINT('Ctrl Pts',(18.974816073814,7.65841335587266,0.));
#18298=CARTESIAN_POINT('Ctrl Pts',(19.0246514144531,7.65711415727855,0.));
#18299=CARTESIAN_POINT('Ctrl Pts',(19.0745543888799,7.65551129907201,0.));
#18300=CARTESIAN_POINT('Ctrl Pts',(19.1245234597312,7.65360662280609,0.));
#18301=CARTESIAN_POINT('Ctrl Pts',(19.1745571539291,7.65140181220525,0.));
#18302=CARTESIAN_POINT('Ctrl Pts',(19.224653915265,7.64889882291923,0.));
#18303=CARTESIAN_POINT('Ctrl Pts',(19.2748120456486,7.64610005549613,0.));
#18304=CARTESIAN_POINT('Ctrl Pts',(19.3250297839295,7.64300812875339,0.));
#18305=CARTESIAN_POINT('Ctrl Pts',(19.3753053524647,7.6396257482276,0.));
#18306=CARTESIAN_POINT('Ctrl Pts',(19.4256370121006,7.63595554930654,0.));
#18307=CARTESIAN_POINT('Ctrl Pts',(19.4760231231881,7.63199992715365,0.));
#18308=CARTESIAN_POINT('Ctrl Pts',(19.5264621687521,7.62776096538883,0.));
#18309=CARTESIAN_POINT('Ctrl Pts',(19.5769527121826,7.62324053735219,0.));
#18310=CARTESIAN_POINT('Ctrl Pts',(19.6274933688524,7.6184403707059,0.));
#18311=CARTESIAN_POINT('Ctrl Pts',(19.6780827744426,7.61336212350879,0.));
#18312=CARTESIAN_POINT('Ctrl Pts',(19.7287195480601,7.60800746969261,0.));
#18313=CARTESIAN_POINT('Ctrl Pts',(19.7794022782484,7.60237814110186,0.));
#18314=CARTESIAN_POINT('Ctrl Pts',(19.830129556152,7.59647587605448,0.));
#18315=CARTESIAN_POINT('Ctrl Pts',(19.8808999994024,7.59030238888852,0.));
#18316=CARTESIAN_POINT('Ctrl Pts',(19.931712276832,7.58385933533351,0.));
#18317=CARTESIAN_POINT('Ctrl Pts',(19.9825651387294,7.57714827622806,0.));
#18318=CARTESIAN_POINT('Ctrl Pts',(20.0334574248556,7.57017066105973,0.));
#18319=CARTESIAN_POINT('Ctrl Pts',(20.0843880130978,7.5629278654946,0.));
#18320=CARTESIAN_POINT('Ctrl Pts',(20.1353557774357,7.55542122125494,0.));
#18321=CARTESIAN_POINT('Ctrl Pts',(20.1863595454674,7.54765204869254,0.));
#18322=CARTESIAN_POINT('Ctrl Pts',(20.2373980474879,7.53962169534167,0.));
#18323=CARTESIAN_POINT('Ctrl Pts',(20.2884698940944,7.53133155804008,0.));
#18324=CARTESIAN_POINT('Ctrl Pts',(20.3395736743243,7.52278303006887,0.));
#18325=CARTESIAN_POINT('Ctrl Pts',(20.3907080367098,7.51397746081993,0.));
#18326=CARTESIAN_POINT('Ctrl Pts',(20.4418717748497,7.50491611266253,0.));
#18327=CARTESIAN_POINT('Ctrl Pts',(20.4930639156161,7.49560012018405,0.));
#18328=CARTESIAN_POINT('Ctrl Pts',(20.5545277683621,7.48411651832412,0.));
#18329=CARTESIAN_POINT('Ctrl Pts',(20.6057817877246,7.47423073598682,0.));
#18330=CARTESIAN_POINT('Ctrl Pts',(20.6468066077586,7.46612041736313,0.));
#18331=CARTESIAN_POINT('Ctrl Pts',(20.6775873630604,7.45992433946823,0.));
#18332=CARTESIAN_POINT('Ctrl Pts',(20.698113262342,7.45574324794401,0.));
#18333=CARTESIAN_POINT('',(20.698113262342,7.45574324794407,13.));
#18334=CARTESIAN_POINT('Ctrl Pts',(20.698113262342,7.45574324794401,13.));
#18335=CARTESIAN_POINT('Ctrl Pts',(20.5970733923829,7.47632490126386,13.));
#18336=CARTESIAN_POINT('Ctrl Pts',(20.4961877829119,7.49544541992866,13.));
#18337=CARTESIAN_POINT('Ctrl Pts',(20.3954689812661,7.51308219876085,13.));
#18338=CARTESIAN_POINT('Ctrl Pts',(20.2285735541666,7.54230710699806,13.));
#18339=CARTESIAN_POINT('Ctrl Pts',(20.0621477284121,7.56745095724697,13.));
#18340=CARTESIAN_POINT('Ctrl Pts',(19.8963869092994,7.58830059943194,13.));
#18341=CARTESIAN_POINT('Ctrl Pts',(19.7689734227607,7.6043268571332,13.));
#18342=CARTESIAN_POINT('Ctrl Pts',(19.6419503907988,7.61781485456745,13.));
#18343=CARTESIAN_POINT('Ctrl Pts',(19.5154161608668,7.62864367960643,13.));
#18344=CARTESIAN_POINT('Ctrl Pts',(19.3792051088178,7.64030064904313,13.));
#18345=CARTESIAN_POINT('Ctrl Pts',(19.2435576419436,7.64888186449425,13.));
#18346=CARTESIAN_POINT('Ctrl Pts',(19.1086228815965,7.65417053749926,13.));
#18347=CARTESIAN_POINT('Ctrl Pts',(19.0339193340502,7.65709849049128,13.));
#18348=CARTESIAN_POINT('Ctrl Pts',(18.9594327293866,7.65902218177988,13.));
#18349=CARTESIAN_POINT('Ctrl Pts',(18.8851905383007,7.65990168002227,13.));
#18350=CARTESIAN_POINT('Ctrl Pts',(18.8136478507039,7.66074919902834,13.));
#18351=CARTESIAN_POINT('Ctrl Pts',(18.7423342826456,7.66062065570543,13.));
#18352=CARTESIAN_POINT('Ctrl Pts',(18.6712863103749,7.65944821272316,13.));
#18353=CARTESIAN_POINT('Ctrl Pts',(18.6098790735343,7.65843486242485,13.));
#18354=CARTESIAN_POINT('Ctrl Pts',(18.5486692004459,7.65664478986642,13.));
#18355=CARTESIAN_POINT('Ctrl Pts',(18.487665986183,7.65407864074932,13.));
#18356=CARTESIAN_POINT('Ctrl Pts',(18.4438867394649,7.65223703163625,13.));
#18357=CARTESIAN_POINT('Ctrl Pts',(18.4002130340387,7.64999840204417,13.));
#18358=CARTESIAN_POINT('Ctrl Pts',(18.3566609397295,7.64732656570801,13.));
#18359=CARTESIAN_POINT('Ctrl Pts',(18.3138180368763,7.64469823688926,13.));
#18360=CARTESIAN_POINT('Ctrl Pts',(18.2710948581547,7.64164464446501,13.));
#18361=CARTESIAN_POINT('Ctrl Pts',(18.2285117414039,7.63811742049252,13.));
#18362=CARTESIAN_POINT('Ctrl Pts',(18.1915896774841,7.63505911008904,13.));
#18363=CARTESIAN_POINT('Ctrl Pts',(18.1547737067871,7.63164238139629,13.));
#18364=CARTESIAN_POINT('Ctrl Pts',(18.1180614606597,7.62788266168324,13.));
#18365=CARTESIAN_POINT('Ctrl Pts',(18.0848085888946,7.62447721825009,13.));
#18366=CARTESIAN_POINT('Ctrl Pts',(18.0516390300359,7.62079564904865,13.));
#18367=CARTESIAN_POINT('Ctrl Pts',(18.0185473589474,7.61686093613286,13.));
#18368=CARTESIAN_POINT('Ctrl Pts',(17.9906726831367,7.61354654180559,13.));
#18369=CARTESIAN_POINT('Ctrl Pts',(17.9628527178424,7.61005417567813,13.));
#18370=CARTESIAN_POINT('Ctrl Pts',(17.935095231726,7.60636550506403,13.));
#18371=CARTESIAN_POINT('Ctrl Pts',(17.8949271289847,7.60102759731604,13.));
#18372=CARTESIAN_POINT('Ctrl Pts',(17.8548900766178,7.59527782595327,13.));
#18373=CARTESIAN_POINT('Ctrl Pts',(17.8150590775895,7.58891067819837,13.));
#18374=CARTESIAN_POINT('Ctrl Pts',(17.7909916428746,7.58506340053399,13.));
#18375=CARTESIAN_POINT('Ctrl Pts',(17.7670005714583,7.58098742033575,13.));
#18376=CARTESIAN_POINT('Ctrl Pts',(17.7430955910393,7.57665817615414,13.));
#18377=CARTESIAN_POINT('Ctrl Pts',(17.7210484741769,7.57266539512171,13.));
#18378=CARTESIAN_POINT('Ctrl Pts',(17.6990750115351,7.56845593261444,13.));
#18379=CARTESIAN_POINT('Ctrl Pts',(17.6771683090889,7.56405390347121,13.));
#18380=CARTESIAN_POINT('Ctrl Pts',(17.6470334199542,7.55799846630422,13.));
#18381=CARTESIAN_POINT('Ctrl Pts',(17.6170224065569,7.55158552706227,13.));
#18382=CARTESIAN_POINT('Ctrl Pts',(17.5870909090696,7.54495919888595,13.));
#18383=CARTESIAN_POINT('Ctrl Pts',(17.5681018330441,7.54075533806796,13.));
#18384=CARTESIAN_POINT('Ctrl Pts',(17.5491442492123,7.53646718588454,13.));
#18385=CARTESIAN_POINT('Ctrl Pts',(17.5302169634342,7.53210330805877,13.));
#18386=CARTESIAN_POINT('Ctrl Pts',(17.5132306054349,7.52818693083054,13.));
#18387=CARTESIAN_POINT('Ctrl Pts',(17.4962684162077,7.52421025223973,13.));
#18388=CARTESIAN_POINT('Ctrl Pts',(17.4793429836255,7.52014106533042,13.));
#18389=CARTESIAN_POINT('Ctrl Pts',(17.461550983085,7.51586353946286,13.));
#18390=CARTESIAN_POINT('Ctrl Pts',(17.4437995540587,7.51148394212765,13.));
#18391=CARTESIAN_POINT('Ctrl Pts',(17.4261238144457,7.50690601564176,13.));
#18392=CARTESIAN_POINT('Ctrl Pts',(17.3967644500333,7.4993020898714,13.));
#18393=CARTESIAN_POINT('Ctrl Pts',(17.3676168189686,7.49114308216385,13.));
#18394=CARTESIAN_POINT('Ctrl Pts',(17.3388922515559,7.48183975624005,13.));
#18395=CARTESIAN_POINT('Ctrl Pts',(17.3230525028126,7.47670957123173,13.));
#18396=CARTESIAN_POINT('Ctrl Pts',(17.3073418195136,7.47123011547027,13.));
#18397=CARTESIAN_POINT('Ctrl Pts',(17.2917860606183,7.46532888199725,13.));
#18398=CARTESIAN_POINT('Ctrl Pts',(17.2791322530438,7.46052853292248,13.));
#18399=CARTESIAN_POINT('Ctrl Pts',(17.266580931693,7.45544915949809,13.));
#18400=CARTESIAN_POINT('Ctrl Pts',(17.2541372868972,7.45007618140238,13.));
#18401=CARTESIAN_POINT('',(20.698113262342,7.45574324794407,0.));
#18402=CARTESIAN_POINT('Origin',(5.38923623413286E-12,1.75106900012182E-12,
0.));
#18403=CARTESIAN_POINT('',(21.1275013067528,6.1342227326009,0.));
#18404=CARTESIAN_POINT('Origin',(5.38923623413286E-12,1.75106900012182E-12,
0.));
#18405=CARTESIAN_POINT('',(21.1275013067528,6.1342227326009,13.));
#18406=CARTESIAN_POINT('Origin',(5.38923623413286E-12,1.75106900012182E-12,
13.));
#18407=CARTESIAN_POINT('',(21.1275013067528,6.1342227326009,0.));
#18408=CARTESIAN_POINT('Ctrl Pts',(18.337935196262,4.1144891981253,0.));
#18409=CARTESIAN_POINT('Ctrl Pts',(18.337935196262,4.1144891981253,21.));
#18410=CARTESIAN_POINT('Ctrl Pts',(18.3471320125699,4.11655269114951,0.));
#18411=CARTESIAN_POINT('Ctrl Pts',(18.3471320125699,4.11655269114951,21.));
#18412=CARTESIAN_POINT('Ctrl Pts',(18.3654573320481,4.1209201986886,0.));
#18413=CARTESIAN_POINT('Ctrl Pts',(18.3654573320481,4.1209201986886,21.));
#18414=CARTESIAN_POINT('Ctrl Pts',(18.3927403741815,4.12819301671078,0.));
#18415=CARTESIAN_POINT('Ctrl Pts',(18.3927403741815,4.12819301671078,21.));
#18416=CARTESIAN_POINT('Ctrl Pts',(18.4287286547442,4.13926275457062,0.));
#18417=CARTESIAN_POINT('Ctrl Pts',(18.4287286547442,4.13926275457062,21.));
#18418=CARTESIAN_POINT('Ctrl Pts',(18.4731856794913,4.15497867673974,0.));
#18419=CARTESIAN_POINT('Ctrl Pts',(18.4731856794913,4.15497867673974,21.));
#18420=CARTESIAN_POINT('Ctrl Pts',(18.5172668097744,4.17205262766561,0.));
#18421=CARTESIAN_POINT('Ctrl Pts',(18.5172668097744,4.17205262766561,21.));
#18422=CARTESIAN_POINT('Ctrl Pts',(18.5611217636409,4.1899696727862,0.));
#18423=CARTESIAN_POINT('Ctrl Pts',(18.5611217636409,4.1899696727862,21.));
#18424=CARTESIAN_POINT('Ctrl Pts',(18.6048602364653,4.20834600700665,0.));
#18425=CARTESIAN_POINT('Ctrl Pts',(18.6048602364653,4.20834600700665,21.));
#18426=CARTESIAN_POINT('Ctrl Pts',(18.6485210883348,4.22703266508919,0.));
#18427=CARTESIAN_POINT('Ctrl Pts',(18.6485210883348,4.22703266508919,21.));
#18428=CARTESIAN_POINT('Ctrl Pts',(18.6920958920047,4.24603817988452,0.));
#18429=CARTESIAN_POINT('Ctrl Pts',(18.6920958920047,4.24603817988452,21.));
#18430=CARTESIAN_POINT('Ctrl Pts',(18.735547949685,4.26546636161933,0.));
#18431=CARTESIAN_POINT('Ctrl Pts',(18.735547949685,4.26546636161933,21.));
#18432=CARTESIAN_POINT('Ctrl Pts',(18.778832216358,4.28545098663153,0.));
#18433=CARTESIAN_POINT('Ctrl Pts',(18.778832216358,4.28545098663153,21.));
#18434=CARTESIAN_POINT('Ctrl Pts',(18.8219166495975,4.30608591031526,0.));
#18435=CARTESIAN_POINT('Ctrl Pts',(18.8219166495975,4.30608591031526,21.));
#18436=CARTESIAN_POINT('Ctrl Pts',(18.8647973781745,4.32737526247704,0.));
#18437=CARTESIAN_POINT('Ctrl Pts',(18.8647973781745,4.32737526247704,21.));
#18438=CARTESIAN_POINT('Ctrl Pts',(18.9074876952706,4.34926881342021,0.));
#18439=CARTESIAN_POINT('Ctrl Pts',(18.9074876952706,4.34926881342021,21.));
#18440=CARTESIAN_POINT('Ctrl Pts',(18.9500107909187,4.37168516143122,0.));
#18441=CARTESIAN_POINT('Ctrl Pts',(18.9500107909187,4.37168516143122,21.));
#18442=CARTESIAN_POINT('Ctrl Pts',(18.9923914823906,4.39453820875555,0.));
#18443=CARTESIAN_POINT('Ctrl Pts',(18.9923914823906,4.39453820875555,21.));
#18444=CARTESIAN_POINT('Ctrl Pts',(19.034647328575,4.41776558033332,0.));
#18445=CARTESIAN_POINT('Ctrl Pts',(19.034647328575,4.41776558033332,21.));
#18446=CARTESIAN_POINT('Ctrl Pts',(19.0767833717249,4.44134542994081,0.));
#18447=CARTESIAN_POINT('Ctrl Pts',(19.0767833717249,4.44134542994081,21.));
#18448=CARTESIAN_POINT('Ctrl Pts',(19.1187970904932,4.46528051067021,0.));
#18449=CARTESIAN_POINT('Ctrl Pts',(19.1187970904932,4.46528051067021,21.));
#18450=CARTESIAN_POINT('Ctrl Pts',(19.1606814968494,4.48958819710577,0.));
#18451=CARTESIAN_POINT('Ctrl Pts',(19.1606814968494,4.48958819710577,21.));
#18452=CARTESIAN_POINT('Ctrl Pts',(19.2024287376926,4.51428889122954,0.));
#18453=CARTESIAN_POINT('Ctrl Pts',(19.2024287376926,4.51428889122954,21.));
#18454=CARTESIAN_POINT('Ctrl Pts',(19.2440340196551,4.53939338835151,0.));
#18455=CARTESIAN_POINT('Ctrl Pts',(19.2440340196551,4.53939338835151,21.));
#18456=CARTESIAN_POINT('Ctrl Pts',(19.2854975819105,4.56489651606741,0.));
#18457=CARTESIAN_POINT('Ctrl Pts',(19.2854975819105,4.56489651606741,21.));
#18458=CARTESIAN_POINT('Ctrl Pts',(19.3268225655679,4.59078395765677,0.));
#18459=CARTESIAN_POINT('Ctrl Pts',(19.3268225655679,4.59078395765677,21.));
#18460=CARTESIAN_POINT('Ctrl Pts',(19.3680137353983,4.61703633725712,0.));
#18461=CARTESIAN_POINT('Ctrl Pts',(19.3680137353983,4.61703633725712,21.));
#18462=CARTESIAN_POINT('Ctrl Pts',(19.4090759683639,4.64363405547472,0.));
#18463=CARTESIAN_POINT('Ctrl Pts',(19.4090759683639,4.64363405547472,21.));
#18464=CARTESIAN_POINT('Ctrl Pts',(19.4500125912299,4.67056260851453,0.));
#18465=CARTESIAN_POINT('Ctrl Pts',(19.4500125912299,4.67056260851453,21.));
#18466=CARTESIAN_POINT('Ctrl Pts',(19.4908246636763,4.69781487613784,0.));
#18467=CARTESIAN_POINT('Ctrl Pts',(19.4908246636763,4.69781487613784,21.));
#18468=CARTESIAN_POINT('Ctrl Pts',(19.531511899192,4.72538815796615,0.));
#18469=CARTESIAN_POINT('Ctrl Pts',(19.531511899192,4.72538815796615,21.));
#18470=CARTESIAN_POINT('Ctrl Pts',(19.5720732205813,4.75328238194611,0.));
#18471=CARTESIAN_POINT('Ctrl Pts',(19.5720732205813,4.75328238194611,21.));
#18472=CARTESIAN_POINT('Ctrl Pts',(19.6125074152527,4.7814979936173,0.));
#18473=CARTESIAN_POINT('Ctrl Pts',(19.6125074152527,4.7814979936173,21.));
#18474=CARTESIAN_POINT('Ctrl Pts',(19.6528138625329,4.81003361418061,0.));
#18475=CARTESIAN_POINT('Ctrl Pts',(19.6528138625329,4.81003361418061,21.));
#18476=CARTESIAN_POINT('Ctrl Pts',(19.6929928227072,4.83888510708974,0.));
#18477=CARTESIAN_POINT('Ctrl Pts',(19.6929928227072,4.83888510708974,21.));
#18478=CARTESIAN_POINT('Ctrl Pts',(19.7330450480715,4.86804682289087,0.));
#18479=CARTESIAN_POINT('Ctrl Pts',(19.7330450480715,4.86804682289087,21.));
#18480=CARTESIAN_POINT('Ctrl Pts',(19.772971552601,4.89751233527804,0.));
#18481=CARTESIAN_POINT('Ctrl Pts',(19.772971552601,4.89751233527804,21.));
#18482=CARTESIAN_POINT('Ctrl Pts',(19.8127733387903,4.92727531494346,0.));
#18483=CARTESIAN_POINT('Ctrl Pts',(19.8127733387903,4.92727531494346,21.));
#18484=CARTESIAN_POINT('Ctrl Pts',(19.8524510953961,4.95733049830096,0.));
#18485=CARTESIAN_POINT('Ctrl Pts',(19.8524510953961,4.95733049830096,21.));
#18486=CARTESIAN_POINT('Ctrl Pts',(19.8920050831202,4.98767405031333,0.));
#18487=CARTESIAN_POINT('Ctrl Pts',(19.8920050831202,4.98767405031333,21.));
#18488=CARTESIAN_POINT('Ctrl Pts',(19.931435301086,5.01830302225557,0.));
#18489=CARTESIAN_POINT('Ctrl Pts',(19.931435301086,5.01830302225557,21.));
#18490=CARTESIAN_POINT('Ctrl Pts',(19.9707415879783,5.04921502064063,0.));
#18491=CARTESIAN_POINT('Ctrl Pts',(19.9707415879783,5.04921502064063,21.));
#18492=CARTESIAN_POINT('Ctrl Pts',(20.0099237417205,5.08040781745336,0.));
#18493=CARTESIAN_POINT('Ctrl Pts',(20.0099237417205,5.08040781745336,21.));
#18494=CARTESIAN_POINT('Ctrl Pts',(20.0489816528155,5.11187891582334,0.));
#18495=CARTESIAN_POINT('Ctrl Pts',(20.0489816528155,5.11187891582334,21.));
#18496=CARTESIAN_POINT('Ctrl Pts',(20.087915358486,5.14362537555398,0.));
#18497=CARTESIAN_POINT('Ctrl Pts',(20.087915358486,5.14362537555398,21.));
#18498=CARTESIAN_POINT('Ctrl Pts',(20.1267249732337,5.17564404279922,0.));
#18499=CARTESIAN_POINT('Ctrl Pts',(20.1267249732337,5.17564404279922,21.));
#18500=CARTESIAN_POINT('Ctrl Pts',(20.1654106491899,5.20793168386163,0.));
#18501=CARTESIAN_POINT('Ctrl Pts',(20.1654106491899,5.20793168386163,21.));
#18502=CARTESIAN_POINT('Ctrl Pts',(20.2039725283917,5.2404851444189,0.));
#18503=CARTESIAN_POINT('Ctrl Pts',(20.2039725283917,5.2404851444189,21.));
#18504=CARTESIAN_POINT('Ctrl Pts',(20.2424106921768,5.2733015229815,0.));
#18505=CARTESIAN_POINT('Ctrl Pts',(20.2424106921768,5.2733015229815,21.));
#18506=CARTESIAN_POINT('Ctrl Pts',(20.2807251380077,5.30637824220997,0.));
#18507=CARTESIAN_POINT('Ctrl Pts',(20.2807251380077,5.30637824220997,21.));
#18508=CARTESIAN_POINT('Ctrl Pts',(20.3189158047642,5.33971294212214,0.));
#18509=CARTESIAN_POINT('Ctrl Pts',(20.3189158047642,5.33971294212214,21.));
#18510=CARTESIAN_POINT('Ctrl Pts',(20.3569825877537,5.37330341114649,0.));
#18511=CARTESIAN_POINT('Ctrl Pts',(20.3569825877537,5.37330341114649,21.));
#18512=CARTESIAN_POINT('Ctrl Pts',(20.3949253578015,5.40714750595875,0.));
#18513=CARTESIAN_POINT('Ctrl Pts',(20.3949253578015,5.40714750595875,21.));
#18514=CARTESIAN_POINT('Ctrl Pts',(20.4327439816542,5.44124306065111,0.));
#18515=CARTESIAN_POINT('Ctrl Pts',(20.4327439816542,5.44124306065111,21.));
#18516=CARTESIAN_POINT('Ctrl Pts',(20.4704383353718,5.47558784449851,0.));
#18517=CARTESIAN_POINT('Ctrl Pts',(20.4704383353718,5.47558784449851,21.));
#18518=CARTESIAN_POINT('Ctrl Pts',(20.5080083009242,5.51017962306782,0.));
#18519=CARTESIAN_POINT('Ctrl Pts',(20.5080083009242,5.51017962306782,21.));
#18520=CARTESIAN_POINT('Ctrl Pts',(20.5454537676144,5.5450161968946,0.));
#18521=CARTESIAN_POINT('Ctrl Pts',(20.5454537676144,5.5450161968946,21.));
#18522=CARTESIAN_POINT('Ctrl Pts',(20.5827746317185,5.58009544402475,0.));
#18523=CARTESIAN_POINT('Ctrl Pts',(20.5827746317185,5.58009544402475,21.));
#18524=CARTESIAN_POINT('Ctrl Pts',(20.6199707996366,5.61541536715149,0.));
#18525=CARTESIAN_POINT('Ctrl Pts',(20.6199707996366,5.61541536715149,21.));
#18526=CARTESIAN_POINT('Ctrl Pts',(20.6570421847033,5.65097411164335,0.));
#18527=CARTESIAN_POINT('Ctrl Pts',(20.6570421847033,5.65097411164335,21.));
#18528=CARTESIAN_POINT('Ctrl Pts',(20.6939886877061,5.68676990500163,0.));
#18529=CARTESIAN_POINT('Ctrl Pts',(20.6939886877061,5.68676990500163,21.));
#18530=CARTESIAN_POINT('Ctrl Pts',(20.7308101804425,5.72280100798241,0.));
#18531=CARTESIAN_POINT('Ctrl Pts',(20.7308101804425,5.72280100798241,21.));
#18532=CARTESIAN_POINT('Ctrl Pts',(20.7675064905026,5.75906566327796,0.));
#18533=CARTESIAN_POINT('Ctrl Pts',(20.7675064905026,5.75906566327796,21.));
#18534=CARTESIAN_POINT('Ctrl Pts',(20.8040773827343,5.79556203439644,0.));
#18535=CARTESIAN_POINT('Ctrl Pts',(20.8040773827343,5.79556203439644,21.));
#18536=CARTESIAN_POINT('Ctrl Pts',(20.8405225541277,5.83228817460178,0.));
#18537=CARTESIAN_POINT('Ctrl Pts',(20.8405225541277,5.83228817460178,21.));
#18538=CARTESIAN_POINT('Ctrl Pts',(20.8768416821402,5.86924212736287,0.));
#18539=CARTESIAN_POINT('Ctrl Pts',(20.8768416821402,5.86924212736287,21.));
#18540=CARTESIAN_POINT('Ctrl Pts',(20.9130344665641,5.90642200662599,0.));
#18541=CARTESIAN_POINT('Ctrl Pts',(20.9130344665641,5.90642200662599,21.));
#18542=CARTESIAN_POINT('Ctrl Pts',(20.9491006734021,5.94382608200804,0.));
#18543=CARTESIAN_POINT('Ctrl Pts',(20.9491006734021,5.94382608200804,21.));
#18544=CARTESIAN_POINT('Ctrl Pts',(20.9850401822713,5.98145286361836,0.));
#18545=CARTESIAN_POINT('Ctrl Pts',(20.9850401822713,5.98145286361836,21.));
#18546=CARTESIAN_POINT('Ctrl Pts',(21.0208530236003,6.01930117633044,0.));
#18547=CARTESIAN_POINT('Ctrl Pts',(21.0208530236003,6.01930117633044,21.));
#18548=CARTESIAN_POINT('Ctrl Pts',(21.0565393163693,6.05737013696532,0.));
#18549=CARTESIAN_POINT('Ctrl Pts',(21.0565393163693,6.05737013696532,21.));
#18550=CARTESIAN_POINT('Ctrl Pts',(21.0849872356853,6.08800133883114,0.));
#18551=CARTESIAN_POINT('Ctrl Pts',(21.0849872356853,6.08800133883114,21.));
#18552=CARTESIAN_POINT('Ctrl Pts',(21.1062663590356,6.11107360216958,0.));
#18553=CARTESIAN_POINT('Ctrl Pts',(21.1062663590356,6.11107360216958,21.));
#18554=CARTESIAN_POINT('Ctrl Pts',(21.1204271980506,6.12649903511517,0.));
#18555=CARTESIAN_POINT('Ctrl Pts',(21.1204271980506,6.12649903511517,21.));
#18556=CARTESIAN_POINT('Ctrl Pts',(21.1275013067528,6.1342227326009,0.));
#18557=CARTESIAN_POINT('Ctrl Pts',(21.1275013067528,6.1342227326009,21.));
#18558=CARTESIAN_POINT('Ctrl Pts',(18.337935196262,4.1144891981253,0.));
#18559=CARTESIAN_POINT('Ctrl Pts',(18.3471320125699,4.11655269114951,0.));
#18560=CARTESIAN_POINT('Ctrl Pts',(18.3654573320481,4.1209201986886,0.));
#18561=CARTESIAN_POINT('Ctrl Pts',(18.3927403741815,4.12819301671078,0.));
#18562=CARTESIAN_POINT('Ctrl Pts',(18.4287286547442,4.13926275457062,0.));
#18563=CARTESIAN_POINT('Ctrl Pts',(18.4731856794913,4.15497867673974,0.));
#18564=CARTESIAN_POINT('Ctrl Pts',(18.5172668097744,4.17205262766561,0.));
#18565=CARTESIAN_POINT('Ctrl Pts',(18.5611217636409,4.1899696727862,0.));
#18566=CARTESIAN_POINT('Ctrl Pts',(18.6048602364653,4.20834600700665,0.));
#18567=CARTESIAN_POINT('Ctrl Pts',(18.6485210883348,4.22703266508919,0.));
#18568=CARTESIAN_POINT('Ctrl Pts',(18.6920958920047,4.24603817988452,0.));
#18569=CARTESIAN_POINT('Ctrl Pts',(18.735547949685,4.26546636161933,0.));
#18570=CARTESIAN_POINT('Ctrl Pts',(18.778832216358,4.28545098663153,0.));
#18571=CARTESIAN_POINT('Ctrl Pts',(18.8219166495975,4.30608591031526,0.));
#18572=CARTESIAN_POINT('Ctrl Pts',(18.8647973781745,4.32737526247704,0.));
#18573=CARTESIAN_POINT('Ctrl Pts',(18.9074876952706,4.34926881342021,0.));
#18574=CARTESIAN_POINT('Ctrl Pts',(18.9500107909187,4.37168516143122,0.));
#18575=CARTESIAN_POINT('Ctrl Pts',(18.9923914823906,4.39453820875555,0.));
#18576=CARTESIAN_POINT('Ctrl Pts',(19.034647328575,4.41776558033332,0.));
#18577=CARTESIAN_POINT('Ctrl Pts',(19.0767833717249,4.44134542994081,0.));
#18578=CARTESIAN_POINT('Ctrl Pts',(19.1187970904932,4.46528051067021,0.));
#18579=CARTESIAN_POINT('Ctrl Pts',(19.1606814968494,4.48958819710577,0.));
#18580=CARTESIAN_POINT('Ctrl Pts',(19.2024287376926,4.51428889122954,0.));
#18581=CARTESIAN_POINT('Ctrl Pts',(19.2440340196551,4.53939338835151,0.));
#18582=CARTESIAN_POINT('Ctrl Pts',(19.2854975819105,4.56489651606741,0.));
#18583=CARTESIAN_POINT('Ctrl Pts',(19.3268225655679,4.59078395765677,0.));
#18584=CARTESIAN_POINT('Ctrl Pts',(19.3680137353983,4.61703633725712,0.));
#18585=CARTESIAN_POINT('Ctrl Pts',(19.4090759683639,4.64363405547472,0.));
#18586=CARTESIAN_POINT('Ctrl Pts',(19.4500125912299,4.67056260851453,0.));
#18587=CARTESIAN_POINT('Ctrl Pts',(19.4908246636763,4.69781487613784,0.));
#18588=CARTESIAN_POINT('Ctrl Pts',(19.531511899192,4.72538815796615,0.));
#18589=CARTESIAN_POINT('Ctrl Pts',(19.5720732205813,4.75328238194611,0.));
#18590=CARTESIAN_POINT('Ctrl Pts',(19.6125074152527,4.7814979936173,0.));
#18591=CARTESIAN_POINT('Ctrl Pts',(19.6528138625329,4.81003361418061,0.));
#18592=CARTESIAN_POINT('Ctrl Pts',(19.6929928227072,4.83888510708974,0.));
#18593=CARTESIAN_POINT('Ctrl Pts',(19.7330450480715,4.86804682289087,0.));
#18594=CARTESIAN_POINT('Ctrl Pts',(19.772971552601,4.89751233527804,0.));
#18595=CARTESIAN_POINT('Ctrl Pts',(19.8127733387903,4.92727531494346,0.));
#18596=CARTESIAN_POINT('Ctrl Pts',(19.8524510953961,4.95733049830096,0.));
#18597=CARTESIAN_POINT('Ctrl Pts',(19.8920050831202,4.98767405031333,0.));
#18598=CARTESIAN_POINT('Ctrl Pts',(19.931435301086,5.01830302225557,0.));
#18599=CARTESIAN_POINT('Ctrl Pts',(19.9707415879783,5.04921502064063,0.));
#18600=CARTESIAN_POINT('Ctrl Pts',(20.0099237417205,5.08040781745336,0.));
#18601=CARTESIAN_POINT('Ctrl Pts',(20.0489816528155,5.11187891582334,0.));
#18602=CARTESIAN_POINT('Ctrl Pts',(20.087915358486,5.14362537555398,0.));
#18603=CARTESIAN_POINT('Ctrl Pts',(20.1267249732337,5.17564404279922,0.));
#18604=CARTESIAN_POINT('Ctrl Pts',(20.1654106491899,5.20793168386163,0.));
#18605=CARTESIAN_POINT('Ctrl Pts',(20.2039725283917,5.2404851444189,0.));
#18606=CARTESIAN_POINT('Ctrl Pts',(20.2424106921768,5.2733015229815,0.));
#18607=CARTESIAN_POINT('Ctrl Pts',(20.2807251380077,5.30637824220997,0.));
#18608=CARTESIAN_POINT('Ctrl Pts',(20.3189158047642,5.33971294212214,0.));
#18609=CARTESIAN_POINT('Ctrl Pts',(20.3569825877537,5.37330341114649,0.));
#18610=CARTESIAN_POINT('Ctrl Pts',(20.3949253578015,5.40714750595875,0.));
#18611=CARTESIAN_POINT('Ctrl Pts',(20.4327439816542,5.44124306065111,0.));
#18612=CARTESIAN_POINT('Ctrl Pts',(20.4704383353718,5.47558784449851,0.));
#18613=CARTESIAN_POINT('Ctrl Pts',(20.5080083009242,5.51017962306782,0.));
#18614=CARTESIAN_POINT('Ctrl Pts',(20.5454537676144,5.5450161968946,0.));
#18615=CARTESIAN_POINT('Ctrl Pts',(20.5827746317185,5.58009544402475,0.));
#18616=CARTESIAN_POINT('Ctrl Pts',(20.6199707996366,5.61541536715149,0.));
#18617=CARTESIAN_POINT('Ctrl Pts',(20.6570421847033,5.65097411164335,0.));
#18618=CARTESIAN_POINT('Ctrl Pts',(20.6939886877061,5.68676990500163,0.));
#18619=CARTESIAN_POINT('Ctrl Pts',(20.7308101804425,5.72280100798241,0.));
#18620=CARTESIAN_POINT('Ctrl Pts',(20.7675064905026,5.75906566327796,0.));
#18621=CARTESIAN_POINT('Ctrl Pts',(20.8040773827343,5.79556203439644,0.));
#18622=CARTESIAN_POINT('Ctrl Pts',(20.8405225541277,5.83228817460178,0.));
#18623=CARTESIAN_POINT('Ctrl Pts',(20.8768416821402,5.86924212736287,0.));
#18624=CARTESIAN_POINT('Ctrl Pts',(20.9130344665641,5.90642200662599,0.));
#18625=CARTESIAN_POINT('Ctrl Pts',(20.9491006734021,5.94382608200804,0.));
#18626=CARTESIAN_POINT('Ctrl Pts',(20.9850401822713,5.98145286361836,0.));
#18627=CARTESIAN_POINT('Ctrl Pts',(21.0280155918661,6.02687083887286,0.));
#18628=CARTESIAN_POINT('Ctrl Pts',(21.0636702474951,6.06499496148844,0.));
#18629=CARTESIAN_POINT('Ctrl Pts',(21.0920928984154,6.09567013127871,0.));
#18630=CARTESIAN_POINT('Ctrl Pts',(21.1133530893457,6.11877533761502,0.));
#18631=CARTESIAN_POINT('Ctrl Pts',(21.1275013067528,6.1342227326009,0.));
#18632=CARTESIAN_POINT('Ctrl Pts',(18.337935196262,4.1144891981253,13.));
#18633=CARTESIAN_POINT('Ctrl Pts',(18.3534360435722,4.11796712888124,13.));
#18634=CARTESIAN_POINT('Ctrl Pts',(18.3688191549147,4.12185943359325,13.));
#18635=CARTESIAN_POINT('Ctrl Pts',(18.3840926405051,4.12613856044905,13.));
#18636=CARTESIAN_POINT('Ctrl Pts',(18.4019943079695,4.13115401717352,13.));
#18637=CARTESIAN_POINT('Ctrl Pts',(18.4197456248504,4.13670006308074,13.));
#18638=CARTESIAN_POINT('Ctrl Pts',(18.4373797424396,4.14266378080247,13.));
#18639=CARTESIAN_POINT('Ctrl Pts',(18.462191789787,4.15105501703698,13.));
#18640=CARTESIAN_POINT('Ctrl Pts',(18.4867739015687,4.16026629329012,13.));
#18641=CARTESIAN_POINT('Ctrl Pts',(18.5112408492841,4.16990400114915,13.));
#18642=CARTESIAN_POINT('Ctrl Pts',(18.5275152282521,4.17631459685994,13.));
#18643=CARTESIAN_POINT('Ctrl Pts',(18.5437392096415,4.18291190640452,13.));
#18644=CARTESIAN_POINT('Ctrl Pts',(18.5599376581282,4.18960898616729,13.));
#18645=CARTESIAN_POINT('Ctrl Pts',(18.5769891804621,4.19665876042442,13.));
#18646=CARTESIAN_POINT('Ctrl Pts',(18.59401265779,4.20381824254071,13.));
#18647=CARTESIAN_POINT('Ctrl Pts',(18.6110185062743,4.21104759333406,13.));
#18648=CARTESIAN_POINT('Ctrl Pts',(18.6299044319261,4.21907618312892,13.));
#18649=CARTESIAN_POINT('Ctrl Pts',(18.648768228348,4.22719219296854,13.));
#18650=CARTESIAN_POINT('Ctrl Pts',(18.6676042988209,4.23540730606195,13.));
#18651=CARTESIAN_POINT('Ctrl Pts',(18.6960005892894,4.24779198778028,13.));
#18652=CARTESIAN_POINT('Ctrl Pts',(18.7243319351414,4.26040793122445,13.));
#18653=CARTESIAN_POINT('Ctrl Pts',(18.7525479285473,4.27340283280954,13.));
#18654=CARTESIAN_POINT('Ctrl Pts',(18.7730462308896,4.28284334471236,13.));
#18655=CARTESIAN_POINT('Ctrl Pts',(18.793482731242,4.29248702329332,13.));
#18656=CARTESIAN_POINT('Ctrl Pts',(18.8138501272064,4.30235320730602,13.));
#18657=CARTESIAN_POINT('Ctrl Pts',(18.8387475247408,4.31441377243381,13.));
#18658=CARTESIAN_POINT('Ctrl Pts',(18.8635420328707,4.32680560861507,13.));
#18659=CARTESIAN_POINT('Ctrl Pts',(18.8882460103409,4.33948253067256,13.));
#18660=CARTESIAN_POINT('Ctrl Pts',(18.9149304060407,4.35317571043872,13.));
#18661=CARTESIAN_POINT('Ctrl Pts',(18.9415109548862,4.3671958076699,13.));
#18662=CARTESIAN_POINT('Ctrl Pts',(18.9680129070487,4.38145466526891,13.));
#18663=CARTESIAN_POINT('Ctrl Pts',(18.9924793847863,4.39461837562023,13.));
#18664=CARTESIAN_POINT('Ctrl Pts',(19.0168796293089,4.40798318216942,13.));
#18665=CARTESIAN_POINT('Ctrl Pts',(19.0412206987801,4.42152146521284,13.));
#18666=CARTESIAN_POINT('Ctrl Pts',(19.074289291449,4.43991391785044,13.));
#18667=CARTESIAN_POINT('Ctrl Pts',(19.1072480694626,4.45862842575511,13.));
#18668=CARTESIAN_POINT('Ctrl Pts',(19.1400849915655,4.47769255659232,13.));
#18669=CARTESIAN_POINT('Ctrl Pts',(19.1717719121569,4.49608903108798,13.));
#18670=CARTESIAN_POINT('Ctrl Pts',(19.2033430482091,4.51481852735374,13.));
#18671=CARTESIAN_POINT('Ctrl Pts',(19.2347910921211,4.53389559671967,13.));
#18672=CARTESIAN_POINT('Ctrl Pts',(19.2775141409376,4.55981232998548,13.));
#18673=CARTESIAN_POINT('Ctrl Pts',(19.3200109589111,4.5863674395711,13.));
#18674=CARTESIAN_POINT('Ctrl Pts',(19.3623013140095,4.61347737153013,13.));
#18675=CARTESIAN_POINT('Ctrl Pts',(19.3994736167756,4.63730641236946,13.));
#18676=CARTESIAN_POINT('Ctrl Pts',(19.4364884569407,4.66155758358413,13.));
#18677=CARTESIAN_POINT('Ctrl Pts',(19.4733518501762,4.68619912918312,13.));
#18678=CARTESIAN_POINT('Ctrl Pts',(19.5276974416099,4.7225267499439,13.));
#18679=CARTESIAN_POINT('Ctrl Pts',(19.5817111524207,4.75971143884683,13.));
#18680=CARTESIAN_POINT('Ctrl Pts',(19.635383906176,4.79774570279521,13.));
#18681=CARTESIAN_POINT('Ctrl Pts',(19.7031194451446,4.84574531502973,13.));
#18682=CARTESIAN_POINT('Ctrl Pts',(19.7703134645214,4.89509304253072,13.));
#18683=CARTESIAN_POINT('Ctrl Pts',(19.8369838016228,4.94566457604163,13.));
#18684=CARTESIAN_POINT('Ctrl Pts',(19.927293913377,5.01416761714691,13.));
#18685=CARTESIAN_POINT('Ctrl Pts',(20.0166413601247,5.08492180299973,13.));
#18686=CARTESIAN_POINT('Ctrl Pts',(20.1050225702956,5.15778644827742,13.));
#18687=CARTESIAN_POINT('Ctrl Pts',(20.1838167339246,5.22274718791513,13.));
#18688=CARTESIAN_POINT('Ctrl Pts',(20.2618454270691,5.28937724262181,13.));
#18689=CARTESIAN_POINT('Ctrl Pts',(20.3391090337862,5.35757729693952,13.));
#18690=CARTESIAN_POINT('Ctrl Pts',(20.4486128110626,5.45423552809844,13.));
#18691=CARTESIAN_POINT('Ctrl Pts',(20.55657724138,5.55405241094525,13.));
#18692=CARTESIAN_POINT('Ctrl Pts',(20.6629906951036,5.65680258457791,13.));
#18693=CARTESIAN_POINT('Ctrl Pts',(20.7456501415197,5.73661648192293,13.));
#18694=CARTESIAN_POINT('Ctrl Pts',(20.8273750326667,5.81820510886241,13.));
#18695=CARTESIAN_POINT('Ctrl Pts',(20.9081522149365,5.90147459235682,13.));
#18696=CARTESIAN_POINT('Ctrl Pts',(20.9780305832912,5.97350898965602,13.));
#18697=CARTESIAN_POINT('Ctrl Pts',(21.0471984365026,6.04679718413474,13.));
#18698=CARTESIAN_POINT('Ctrl Pts',(21.11565843993,6.12131239104349,13.));
#18699=CARTESIAN_POINT('Ctrl Pts',(21.1196084177252,6.12561173953841,13.));
#18700=CARTESIAN_POINT('Ctrl Pts',(21.1235560399575,6.12991518680116,13.));
#18701=CARTESIAN_POINT('Ctrl Pts',(21.1275013067528,6.1342227326009,13.));
#18702=CARTESIAN_POINT('Origin',(0.,0.,0.));
#18703=CARTESIAN_POINT('Origin',(0.,0.,0.));
#18704=CARTESIAN_POINT('Origin',(0.,0.,0.));
#18705=CARTESIAN_POINT('Origin',(0.,0.,0.));
#18706=CARTESIAN_POINT('Origin',(0.,0.,0.));
#18707=CARTESIAN_POINT('Origin',(0.,0.,0.));
#18708=CARTESIAN_POINT('Origin',(0.,0.,0.));
#18709=CARTESIAN_POINT('Origin',(0.,0.,0.));
#18710=CARTESIAN_POINT('Origin',(0.,0.,0.));
#18711=CARTESIAN_POINT('Origin',(0.,0.,0.));
#18712=CARTESIAN_POINT('Origin',(0.,0.,0.));
#18713=CARTESIAN_POINT('Origin',(0.,0.,0.));
#18714=CARTESIAN_POINT('Origin',(0.,0.,0.));
#18715=CARTESIAN_POINT('Origin',(0.,0.,0.));
#18716=CARTESIAN_POINT('Origin',(0.,0.,0.));
#18717=CARTESIAN_POINT('Origin',(0.,0.,0.));
#18718=CARTESIAN_POINT('Origin',(0.,0.,0.));
#18719=CARTESIAN_POINT('Origin',(0.,0.,0.));
#18720=CARTESIAN_POINT('',(17.4952923049513,2.59023998199238,0.));
#18721=CARTESIAN_POINT('Origin',(0.,0.,0.));
#18722=CARTESIAN_POINT('',(18.5778175999297,1.74105979901401,0.));
#18723=CARTESIAN_POINT('Origin',(18.4845093299966,2.73669706567396,0.));
#18724=CARTESIAN_POINT('',(18.7118598491961,1.75362185428836,0.));
#18725=CARTESIAN_POINT('',(17.5988843254813,1.64931697933718,0.));
#18726=CARTESIAN_POINT('',(21.9890268624765,0.694764450219646,0.));
#18727=CARTESIAN_POINT('Ctrl Pts',(18.7118598491961,1.75362185428836,0.));
#18728=CARTESIAN_POINT('Ctrl Pts',(18.7212441956871,1.75450132833464,0.));
#18729=CARTESIAN_POINT('Ctrl Pts',(18.7400222442427,1.75601041697575,0.));
#18730=CARTESIAN_POINT('Ctrl Pts',(18.7682173836138,1.75752447968136,0.));
#18731=CARTESIAN_POINT('Ctrl Pts',(18.8058650094752,1.7581175236483,0.));
#18732=CARTESIAN_POINT('Ctrl Pts',(18.8530026395886,1.75690876962597,0.));
#18733=CARTESIAN_POINT('Ctrl Pts',(18.9002024267872,1.75429229572775,0.));
#18734=CARTESIAN_POINT('Ctrl Pts',(18.947447637865,1.75080409924533,0.));
#18735=CARTESIAN_POINT('Ctrl Pts',(18.9947239970259,1.74684309825012,0.));
#18736=CARTESIAN_POINT('Ctrl Pts',(19.0420224296189,1.74256297552949,0.));
#18737=CARTESIAN_POINT('Ctrl Pts',(19.0893375576541,1.7379530116984,0.));
#18738=CARTESIAN_POINT('Ctrl Pts',(19.1366665585833,1.73290313712353,0.));
#18739=CARTESIAN_POINT('Ctrl Pts',(19.1840079312107,1.72727220327098,0.));
#18740=CARTESIAN_POINT('Ctrl Pts',(19.2313602042899,1.72096104670234,0.));
#18741=CARTESIAN_POINT('Ctrl Pts',(19.2787209722437,1.71396454346262,0.));
#18742=CARTESIAN_POINT('Ctrl Pts',(19.3260873558094,1.70633457265124,0.));
#18743=CARTESIAN_POINT('Ctrl Pts',(19.3734562555057,1.69815571801252,0.));
#18744=CARTESIAN_POINT('Ctrl Pts',(19.4208246682917,1.68951753233571,0.));
#18745=CARTESIAN_POINT('Ctrl Pts',(19.4681900187091,1.68048476382294,0.));
#18746=CARTESIAN_POINT('Ctrl Pts',(19.5155503513712,1.67107974760949,0.));
#18747=CARTESIAN_POINT('Ctrl Pts',(19.5629041190868,1.66129908621006,0.));
#18748=CARTESIAN_POINT('Ctrl Pts',(19.6102500448855,1.65112409599283,0.));
#18749=CARTESIAN_POINT('Ctrl Pts',(19.6575869645839,1.64053294677821,0.));
#18750=CARTESIAN_POINT('Ctrl Pts',(19.7049136553525,1.62951389038422,0.));
#18751=CARTESIAN_POINT('Ctrl Pts',(19.7522287462982,1.61807191996834,0.));
#18752=CARTESIAN_POINT('Ctrl Pts',(19.7995308006834,1.60622162219699,0.));
#18753=CARTESIAN_POINT('Ctrl Pts',(19.8468183626037,1.59398289700559,0.));
#18754=CARTESIAN_POINT('Ctrl Pts',(19.8940900137801,1.58137589158952,0.));
#18755=CARTESIAN_POINT('Ctrl Pts',(19.9413444362352,1.56841542790452,0.));
#18756=CARTESIAN_POINT('Ctrl Pts',(19.9885804375096,1.55510860515913,0.));
#18757=CARTESIAN_POINT('Ctrl Pts',(20.0357969106526,1.54145790302918,0.));
#18758=CARTESIAN_POINT('Ctrl Pts',(20.0829928089241,1.52746305716964,0.));
#18759=CARTESIAN_POINT('Ctrl Pts',(20.1301671167606,1.51312326913583,0.));
#18760=CARTESIAN_POINT('Ctrl Pts',(20.1773188177942,1.49843965844502,0.));
#18761=CARTESIAN_POINT('Ctrl Pts',(20.224446881308,1.48341623961914,0.));
#18762=CARTESIAN_POINT('Ctrl Pts',(20.2715502770004,1.46805861808021,0.));
#18763=CARTESIAN_POINT('Ctrl Pts',(20.3186279833818,1.45237321894404,0.));
#18764=CARTESIAN_POINT('Ctrl Pts',(20.3656789980171,1.43636637152782,0.));
#18765=CARTESIAN_POINT('Ctrl Pts',(20.4127023494155,1.4200432946371,0.));
#18766=CARTESIAN_POINT('Ctrl Pts',(20.4596971004275,1.40340771617024,0.));
#18767=CARTESIAN_POINT('Ctrl Pts',(20.5066623390132,1.38646244026049,0.));
#18768=CARTESIAN_POINT('Ctrl Pts',(20.5535971721246,1.36920969340018,0.));
#18769=CARTESIAN_POINT('Ctrl Pts',(20.6005007190809,1.35165153211253,0.));
#18770=CARTESIAN_POINT('Ctrl Pts',(20.6473721041685,1.3337902972259,0.));
#18771=CARTESIAN_POINT('Ctrl Pts',(20.694210454218,1.31562879653596,0.));
#18772=CARTESIAN_POINT('Ctrl Pts',(20.7410149035348,1.2971700649115,0.));
#18773=CARTESIAN_POINT('Ctrl Pts',(20.7877845975367,1.27841722479262,0.));
#18774=CARTESIAN_POINT('Ctrl Pts',(20.83451869657,1.25937332001005,0.));
#18775=CARTESIAN_POINT('Ctrl Pts',(20.881216381382,1.24004113517905,0.));
#18776=CARTESIAN_POINT('Ctrl Pts',(20.9278768531175,1.22042312071096,0.));
#18777=CARTESIAN_POINT('Ctrl Pts',(20.9744993243732,1.20052150219503,0.));
#18778=CARTESIAN_POINT('Ctrl Pts',(21.0210830121673,1.18033835060894,0.));
#18779=CARTESIAN_POINT('Ctrl Pts',(21.0676271313238,1.15987566445807,0.));
#18780=CARTESIAN_POINT('Ctrl Pts',(21.1141308858087,1.13913546246555,0.));
#18781=CARTESIAN_POINT('Ctrl Pts',(21.1605934684164,1.11811982787746,0.));
#18782=CARTESIAN_POINT('Ctrl Pts',(21.2070140764156,1.09683084929266,0.));
#18783=CARTESIAN_POINT('Ctrl Pts',(21.2533919248553,1.07527058431887,0.));
#18784=CARTESIAN_POINT('Ctrl Pts',(21.2997262593683,1.05344101900192,0.));
#18785=CARTESIAN_POINT('Ctrl Pts',(21.3460163737343,1.03134402396953,0.));
#18786=CARTESIAN_POINT('Ctrl Pts',(21.3922616124166,1.00898133629988,0.));
#18787=CARTESIAN_POINT('Ctrl Pts',(21.4384613333266,0.986354611081135,0.));
#18788=CARTESIAN_POINT('Ctrl Pts',(21.4846148770804,0.963465462815772,0.));
#18789=CARTESIAN_POINT('Ctrl Pts',(21.5307215366685,0.94031550952515,0.));
#18790=CARTESIAN_POINT('Ctrl Pts',(21.5767805209408,0.916906425150854,0.));
#18791=CARTESIAN_POINT('Ctrl Pts',(21.6227909401433,0.893239967513673,0.));
#18792=CARTESIAN_POINT('Ctrl Pts',(21.6687518829182,0.869317897714099,0.));
#18793=CARTESIAN_POINT('Ctrl Pts',(21.7146624809285,0.845141916726558,0.));
#18794=CARTESIAN_POINT('Ctrl Pts',(21.7605219769118,0.820713597934077,0.));
#18795=CARTESIAN_POINT('Ctrl Pts',(21.8063297959755,0.796034321106413,0.));
#18796=CARTESIAN_POINT('Ctrl Pts',(21.8612367655148,0.766119391688713,0.));
#18797=CARTESIAN_POINT('Ctrl Pts',(21.9069273598709,0.740879090965099,0.));
#18798=CARTESIAN_POINT('Ctrl Pts',(21.9434380560096,0.720488353007148,0.));
#18799=CARTESIAN_POINT('Ctrl Pts',(21.970797600548,0.705083756261759,0.));
#18800=CARTESIAN_POINT('Ctrl Pts',(21.9890268624765,0.694764450219581,0.));
#18801=CARTESIAN_POINT('',(21.9890268624765,-0.694764450219581,0.));
#18802=CARTESIAN_POINT('Origin',(5.6665783176868E-12,0.,0.));
#18803=CARTESIAN_POINT('',(18.7118598491961,-1.75362185428836,0.));
#18804=CARTESIAN_POINT('Ctrl Pts',(18.7118598491961,-1.75362185428836,0.));
#18805=CARTESIAN_POINT('Ctrl Pts',(18.7212441956871,-1.75450132833464,0.));
#18806=CARTESIAN_POINT('Ctrl Pts',(18.7400222442427,-1.75601041697575,0.));
#18807=CARTESIAN_POINT('Ctrl Pts',(18.7682173836138,-1.75752447968136,0.));
#18808=CARTESIAN_POINT('Ctrl Pts',(18.8058650094752,-1.7581175236483,0.));
#18809=CARTESIAN_POINT('Ctrl Pts',(18.8530026395886,-1.75690876962597,0.));
#18810=CARTESIAN_POINT('Ctrl Pts',(18.9002024267872,-1.75429229572775,0.));
#18811=CARTESIAN_POINT('Ctrl Pts',(18.947447637865,-1.75080409924533,0.));
#18812=CARTESIAN_POINT('Ctrl Pts',(18.9947239970259,-1.74684309825012,0.));
#18813=CARTESIAN_POINT('Ctrl Pts',(19.0420224296189,-1.74256297552949,0.));
#18814=CARTESIAN_POINT('Ctrl Pts',(19.0893375576541,-1.7379530116984,0.));
#18815=CARTESIAN_POINT('Ctrl Pts',(19.1366665585833,-1.73290313712353,0.));
#18816=CARTESIAN_POINT('Ctrl Pts',(19.1840079312107,-1.72727220327098,0.));
#18817=CARTESIAN_POINT('Ctrl Pts',(19.2313602042899,-1.72096104670234,0.));
#18818=CARTESIAN_POINT('Ctrl Pts',(19.2787209722437,-1.71396454346262,0.));
#18819=CARTESIAN_POINT('Ctrl Pts',(19.3260873558094,-1.70633457265124,0.));
#18820=CARTESIAN_POINT('Ctrl Pts',(19.3734562555057,-1.69815571801252,0.));
#18821=CARTESIAN_POINT('Ctrl Pts',(19.4208246682917,-1.68951753233571,0.));
#18822=CARTESIAN_POINT('Ctrl Pts',(19.4681900187091,-1.68048476382294,0.));
#18823=CARTESIAN_POINT('Ctrl Pts',(19.5155503513712,-1.67107974760949,0.));
#18824=CARTESIAN_POINT('Ctrl Pts',(19.5629041190868,-1.66129908621006,0.));
#18825=CARTESIAN_POINT('Ctrl Pts',(19.6102500448855,-1.65112409599283,0.));
#18826=CARTESIAN_POINT('Ctrl Pts',(19.6575869645839,-1.64053294677821,0.));
#18827=CARTESIAN_POINT('Ctrl Pts',(19.7049136553525,-1.62951389038422,0.));
#18828=CARTESIAN_POINT('Ctrl Pts',(19.7522287462982,-1.61807191996834,0.));
#18829=CARTESIAN_POINT('Ctrl Pts',(19.7995308006834,-1.60622162219699,0.));
#18830=CARTESIAN_POINT('Ctrl Pts',(19.8468183626037,-1.59398289700559,0.));
#18831=CARTESIAN_POINT('Ctrl Pts',(19.8940900137801,-1.58137589158952,0.));
#18832=CARTESIAN_POINT('Ctrl Pts',(19.9413444362352,-1.56841542790452,0.));
#18833=CARTESIAN_POINT('Ctrl Pts',(19.9885804375096,-1.55510860515913,0.));
#18834=CARTESIAN_POINT('Ctrl Pts',(20.0357969106526,-1.54145790302918,0.));
#18835=CARTESIAN_POINT('Ctrl Pts',(20.0829928089241,-1.52746305716964,0.));
#18836=CARTESIAN_POINT('Ctrl Pts',(20.1301671167606,-1.51312326913583,0.));
#18837=CARTESIAN_POINT('Ctrl Pts',(20.1773188177942,-1.49843965844502,0.));
#18838=CARTESIAN_POINT('Ctrl Pts',(20.224446881308,-1.48341623961914,0.));
#18839=CARTESIAN_POINT('Ctrl Pts',(20.2715502770004,-1.46805861808021,0.));
#18840=CARTESIAN_POINT('Ctrl Pts',(20.3186279833818,-1.45237321894404,0.));
#18841=CARTESIAN_POINT('Ctrl Pts',(20.3656789980171,-1.43636637152782,0.));
#18842=CARTESIAN_POINT('Ctrl Pts',(20.4127023494155,-1.4200432946371,0.));
#18843=CARTESIAN_POINT('Ctrl Pts',(20.4596971004275,-1.40340771617024,0.));
#18844=CARTESIAN_POINT('Ctrl Pts',(20.5066623390132,-1.38646244026049,0.));
#18845=CARTESIAN_POINT('Ctrl Pts',(20.5535971721246,-1.36920969340018,0.));
#18846=CARTESIAN_POINT('Ctrl Pts',(20.6005007190809,-1.35165153211253,0.));
#18847=CARTESIAN_POINT('Ctrl Pts',(20.6473721041685,-1.3337902972259,0.));
#18848=CARTESIAN_POINT('Ctrl Pts',(20.694210454218,-1.31562879653596,0.));
#18849=CARTESIAN_POINT('Ctrl Pts',(20.7410149035348,-1.2971700649115,0.));
#18850=CARTESIAN_POINT('Ctrl Pts',(20.7877845975367,-1.27841722479262,0.));
#18851=CARTESIAN_POINT('Ctrl Pts',(20.83451869657,-1.25937332001005,0.));
#18852=CARTESIAN_POINT('Ctrl Pts',(20.881216381382,-1.24004113517905,0.));
#18853=CARTESIAN_POINT('Ctrl Pts',(20.9278768531175,-1.22042312071096,0.));
#18854=CARTESIAN_POINT('Ctrl Pts',(20.9744993243732,-1.20052150219503,0.));
#18855=CARTESIAN_POINT('Ctrl Pts',(21.0210830121673,-1.18033835060894,0.));
#18856=CARTESIAN_POINT('Ctrl Pts',(21.0676271313238,-1.15987566445807,0.));
#18857=CARTESIAN_POINT('Ctrl Pts',(21.1141308858087,-1.13913546246555,0.));
#18858=CARTESIAN_POINT('Ctrl Pts',(21.1605934684164,-1.11811982787746,0.));
#18859=CARTESIAN_POINT('Ctrl Pts',(21.2070140764156,-1.09683084929266,0.));
#18860=CARTESIAN_POINT('Ctrl Pts',(21.2533919248553,-1.07527058431887,0.));
#18861=CARTESIAN_POINT('Ctrl Pts',(21.2997262593683,-1.05344101900192,0.));
#18862=CARTESIAN_POINT('Ctrl Pts',(21.3460163737343,-1.03134402396953,0.));
#18863=CARTESIAN_POINT('Ctrl Pts',(21.3922616124166,-1.00898133629988,0.));
#18864=CARTESIAN_POINT('Ctrl Pts',(21.4384613333266,-0.986354611081135,
0.));
#18865=CARTESIAN_POINT('Ctrl Pts',(21.4846148770804,-0.963465462815772,
0.));
#18866=CARTESIAN_POINT('Ctrl Pts',(21.5307215366685,-0.94031550952515,0.));
#18867=CARTESIAN_POINT('Ctrl Pts',(21.5767805209408,-0.916906425150854,
0.));
#18868=CARTESIAN_POINT('Ctrl Pts',(21.6227909401433,-0.893239967513673,
0.));
#18869=CARTESIAN_POINT('Ctrl Pts',(21.6687518829182,-0.869317897714099,
0.));
#18870=CARTESIAN_POINT('Ctrl Pts',(21.7146624809285,-0.845141916726558,
0.));
#18871=CARTESIAN_POINT('Ctrl Pts',(21.7605219769118,-0.820713597934077,
0.));
#18872=CARTESIAN_POINT('Ctrl Pts',(21.8063297959755,-0.796034321106413,
0.));
#18873=CARTESIAN_POINT('Ctrl Pts',(21.8612367655148,-0.766119391688713,
0.));
#18874=CARTESIAN_POINT('Ctrl Pts',(21.9069273598709,-0.740879090965099,
0.));
#18875=CARTESIAN_POINT('Ctrl Pts',(21.9434380560096,-0.720488353007148,
0.));
#18876=CARTESIAN_POINT('Ctrl Pts',(21.970797600548,-0.705083756261759,0.));
#18877=CARTESIAN_POINT('Ctrl Pts',(21.9890268624765,-0.694764450219581,
0.));
#18878=CARTESIAN_POINT('',(18.5778175999297,-1.74105979901401,0.));
#18879=CARTESIAN_POINT('',(17.5988843254813,-1.64931697933718,0.));
#18880=CARTESIAN_POINT('',(17.4952923049513,-2.59023998199238,0.));
#18881=CARTESIAN_POINT('Origin',(18.4845093299966,-2.73669706567396,0.));
#18882=CARTESIAN_POINT('Origin',(0.,0.,0.));
#18883=CARTESIAN_POINT('Origin',(0.,0.,0.));
#18884=CARTESIAN_POINT('Origin',(0.,0.,13.));
#18885=CARTESIAN_POINT('',(17.4952923049513,-2.59023998199238,13.));
#18886=CARTESIAN_POINT('Origin',(0.,0.,13.));
#18887=CARTESIAN_POINT('',(18.5778175999297,-1.74105979901401,13.));
#18888=CARTESIAN_POINT('Origin',(18.4845093299966,-2.73669706567396,13.));
#18889=CARTESIAN_POINT('',(18.7118598491961,-1.75362185428836,13.));
#18890=CARTESIAN_POINT('',(8.79944216274063,-0.824658489668591,13.));
#18891=CARTESIAN_POINT('',(21.9890268624765,-0.694764450219581,13.));
#18892=CARTESIAN_POINT('Ctrl Pts',(18.7118598491961,-1.75362185428836,13.));
#18893=CARTESIAN_POINT('Ctrl Pts',(18.7276767707323,-1.75510417082436,13.));
#18894=CARTESIAN_POINT('Ctrl Pts',(18.7435097673037,-1.75615601189521,13.));
#18895=CARTESIAN_POINT('Ctrl Pts',(18.7593580382054,-1.75680608702586,13.));
#18896=CARTESIAN_POINT('Ctrl Pts',(18.7779333970632,-1.75756802370092,13.));
#18897=CARTESIAN_POINT('Ctrl Pts',(18.7965297250933,-1.7577788791907,13.));
#18898=CARTESIAN_POINT('Ctrl Pts',(18.8151436576621,-1.75755628860662,13.));
#18899=CARTESIAN_POINT('Ctrl Pts',(18.8413343515946,-1.75724309300229,13.));
#18900=CARTESIAN_POINT('Ctrl Pts',(18.8675597701108,-1.75607893899569,13.));
#18901=CARTESIAN_POINT('Ctrl Pts',(18.8938074357046,-1.75447363677736,13.));
#18902=CARTESIAN_POINT('Ctrl Pts',(18.9112662728887,-1.75340585762722,13.));
#18903=CARTESIAN_POINT('Ctrl Pts',(18.9287348768749,-1.75214492936053,13.));
#18904=CARTESIAN_POINT('Ctrl Pts',(18.9462100283206,-1.75078122387692,13.));
#18905=CARTESIAN_POINT('Ctrl Pts',(18.9646054898042,-1.74934570031211,13.));
#18906=CARTESIAN_POINT('Ctrl Pts',(18.9830081804949,-1.74779717198946,13.));
#18907=CARTESIAN_POINT('Ctrl Pts',(19.0014156957677,-1.74617674699393,13.));
#18908=CARTESIAN_POINT('Ctrl Pts',(19.0218582491152,-1.74437717633347,13.));
#18909=CARTESIAN_POINT('Ctrl Pts',(19.0423067705939,-1.74248762596164,13.));
#18910=CARTESIAN_POINT('Ctrl Pts',(19.0627595477178,-1.74049525500507,13.));
#18911=CARTESIAN_POINT('Ctrl Pts',(19.093593101927,-1.73749165908643,13.));
#18912=CARTESIAN_POINT('Ctrl Pts',(19.1244363539391,-1.73424805120627,13.));
#18913=CARTESIAN_POINT('Ctrl Pts',(19.1552870037612,-1.73060838685053,13.));
#18914=CARTESIAN_POINT('Ctrl Pts',(19.1776993263911,-1.72796425026749,13.));
#18915=CARTESIAN_POINT('Ctrl Pts',(19.2001156537922,-1.72510779282615,13.));
#18916=CARTESIAN_POINT('Ctrl Pts',(19.2225350169744,-1.72201836571372,13.));
#18917=CARTESIAN_POINT('Ctrl Pts',(19.2499407687317,-1.71824180561129,13.));
#18918=CARTESIAN_POINT('Ctrl Pts',(19.2773510352358,-1.71411839344011,13.));
#18919=CARTESIAN_POINT('Ctrl Pts',(19.3047632983466,-1.70969587297614,13.));
#18920=CARTESIAN_POINT('Ctrl Pts',(19.3343730920125,-1.70491881688659,13.));
#18921=CARTESIAN_POINT('Ctrl Pts',(19.3639851445034,-1.69979875336899,13.));
#18922=CARTESIAN_POINT('Ctrl Pts',(19.393596228118,-1.69442732753702,13.));
#18923=CARTESIAN_POINT('Ctrl Pts',(19.420933041416,-1.68946845244065,13.));
#18924=CARTESIAN_POINT('Ctrl Pts',(19.4482690053259,-1.68429785630576,13.));
#18925=CARTESIAN_POINT('Ctrl Pts',(19.4756022976024,-1.67894398812401,13.));
#18926=CARTESIAN_POINT('Ctrl Pts',(19.5127359785892,-1.67167048330449,13.));
#18927=CARTESIAN_POINT('Ctrl Pts',(19.5498647401833,-1.66405675112972,13.));
#18928=CARTESIAN_POINT('Ctrl Pts',(19.5869856493472,-1.65607285223917,13.));
#18929=CARTESIAN_POINT('Ctrl Pts',(19.6228065249488,-1.64836856224694,13.));
#18930=CARTESIAN_POINT('Ctrl Pts',(19.6586201922964,-1.6403117703391,13.));
#18931=CARTESIAN_POINT('Ctrl Pts',(19.6944241980566,-1.63188637920554,13.));
#18932=CARTESIAN_POINT('Ctrl Pts',(19.743064943113,-1.62044024927043,13.));
#18933=CARTESIAN_POINT('Ctrl Pts',(19.7916877989836,-1.60831707819959,13.));
#18934=CARTESIAN_POINT('Ctrl Pts',(19.8402857465336,-1.59560243915671,13.));
#18935=CARTESIAN_POINT('Ctrl Pts',(19.8830022859205,-1.58442654785171,13.));
#18936=CARTESIAN_POINT('Ctrl Pts',(19.9256995149344,-1.57280052808225,13.));
#18937=CARTESIAN_POINT('Ctrl Pts',(19.9683733416779,-1.56075644053511,13.));
#18938=CARTESIAN_POINT('Ctrl Pts',(20.0312849226334,-1.54300053143161,13.));
#18939=CARTESIAN_POINT('Ctrl Pts',(20.0941457149814,-1.52432694533669,13.));
#18940=CARTESIAN_POINT('Ctrl Pts',(20.1569447710271,-1.50474000383683,13.));
#18941=CARTESIAN_POINT('Ctrl Pts',(20.23619779263,-1.48002109250969,13.));
#18942=CARTESIAN_POINT('Ctrl Pts',(20.3153523890243,-1.45385270861794,13.));
#18943=CARTESIAN_POINT('Ctrl Pts',(20.3943871108328,-1.4263585893238,13.));
#18944=CARTESIAN_POINT('Ctrl Pts',(20.50144573481,-1.38911568504398,13.));
#18945=CARTESIAN_POINT('Ctrl Pts',(20.6082844519443,-1.34943433504336,13.));
#18946=CARTESIAN_POINT('Ctrl Pts',(20.7148563913151,-1.30744723533842,13.));
#18947=CARTESIAN_POINT('Ctrl Pts',(20.8098680660179,-1.27001463645326,13.));
#18948=CARTESIAN_POINT('Ctrl Pts',(20.9046675817562,-1.23075788122755,13.));
#18949=CARTESIAN_POINT('Ctrl Pts',(20.9992246136264,-1.18977154295355,13.));
#18950=CARTESIAN_POINT('Ctrl Pts',(21.1332379306991,-1.13168263049381,13.));
#18951=CARTESIAN_POINT('Ctrl Pts',(21.2667633188666,-1.07011397738899,13.));
#18952=CARTESIAN_POINT('Ctrl Pts',(21.39972007734,-1.00527632083917,13.));
#18953=CARTESIAN_POINT('Ctrl Pts',(21.5029977296385,-0.954911969106397,
13.));
#18954=CARTESIAN_POINT('Ctrl Pts',(21.6059349886872,-0.902570955902035,
13.));
#18955=CARTESIAN_POINT('Ctrl Pts',(21.7084903363009,-0.848338495094938,
13.));
#18956=CARTESIAN_POINT('Ctrl Pts',(21.7972084616082,-0.801423318406783,
13.));
#18957=CARTESIAN_POINT('Ctrl Pts',(21.8856382915295,-0.75309614865077,13.));
#18958=CARTESIAN_POINT('Ctrl Pts',(21.9737740840291,-0.70338328327774,13.));
#18959=CARTESIAN_POINT('Ctrl Pts',(21.9788593171835,-0.700514964924581,
13.));
#18960=CARTESIAN_POINT('Ctrl Pts',(21.9839435766499,-0.697642020485719,
13.));
#18961=CARTESIAN_POINT('Ctrl Pts',(21.9890268624765,-0.694764450219581,
13.));
#18962=CARTESIAN_POINT('',(21.9890268624765,0.694764450219646,13.));
#18963=CARTESIAN_POINT('Origin',(5.6665783176868E-12,0.,13.));
#18964=CARTESIAN_POINT('',(18.7118598491961,1.75362185428836,13.));
#18965=CARTESIAN_POINT('Ctrl Pts',(21.9890268624765,0.694764450219581,13.));
#18966=CARTESIAN_POINT('Ctrl Pts',(21.899292315352,0.745561803242415,13.));
#18967=CARTESIAN_POINT('Ctrl Pts',(21.8092529632231,0.794921865484829,13.));
#18968=CARTESIAN_POINT('Ctrl Pts',(21.7189137539334,0.842819260803599,13.));
#18969=CARTESIAN_POINT('Ctrl Pts',(21.569217762881,0.922187323878742,13.));
#18970=CARTESIAN_POINT('Ctrl Pts',(21.4187072729658,0.997528955316443,13.));
#18971=CARTESIAN_POINT('Ctrl Pts',(21.2675022586751,1.06858105378595,13.));
#18972=CARTESIAN_POINT('Ctrl Pts',(21.151277217989,1.12319586318354,13.));
#18973=CARTESIAN_POINT('Ctrl Pts',(21.0346391561147,1.17527598651107,13.));
#18974=CARTESIAN_POINT('Ctrl Pts',(20.9176442431357,1.2246760384665,13.));
#18975=CARTESIAN_POINT('Ctrl Pts',(20.7917020384811,1.27785400402849,13.));
#18976=CARTESIAN_POINT('Ctrl Pts',(20.6653453749438,1.327932596435,13.));
#18977=CARTESIAN_POINT('Ctrl Pts',(20.5386490840353,1.37465955658916,13.));
#18978=CARTESIAN_POINT('Ctrl Pts',(20.4685065762054,1.40052887087594,13.));
#18979=CARTESIAN_POINT('Ctrl Pts',(20.3982600593864,1.42537603650614,13.));
#18980=CARTESIAN_POINT('Ctrl Pts',(20.3279233202978,1.4491545876062,13.));
#18981=CARTESIAN_POINT('Ctrl Pts',(20.2601440775423,1.47206853283981,13.));
#18982=CARTESIAN_POINT('Ctrl Pts',(20.1922811205662,1.49398338576682,13.));
#18983=CARTESIAN_POINT('Ctrl Pts',(20.1243481774567,1.51482335746684,13.));
#18984=CARTESIAN_POINT('Ctrl Pts',(20.0656332822855,1.53283548380392,13.));
#18985=CARTESIAN_POINT('Ctrl Pts',(20.0068660708186,1.55004791462172,13.));
#18986=CARTESIAN_POINT('Ctrl Pts',(19.948055582729,1.56645839168308,13.));
#18987=CARTESIAN_POINT('Ctrl Pts',(19.9058499563011,1.57823544857983,13.));
#18988=CARTESIAN_POINT('Ctrl Pts',(19.8636220195312,1.58960230250921,13.));
#18989=CARTESIAN_POINT('Ctrl Pts',(19.8213758735606,1.6005195724384,13.));
#18990=CARTESIAN_POINT('Ctrl Pts',(19.779817653503,1.61125906821305,13.));
#18991=CARTESIAN_POINT('Ctrl Pts',(19.7382418841798,1.62155711747599,13.));
#18992=CARTESIAN_POINT('Ctrl Pts',(19.6966529615092,1.63136143484286,13.));
#18993=CARTESIAN_POINT('Ctrl Pts',(19.6605929222238,1.63986235399904,13.));
#18994=CARTESIAN_POINT('Ctrl Pts',(19.6245230262468,1.64798961249865,13.));
#18995=CARTESIAN_POINT('Ctrl Pts',(19.5884457881434,1.65575861450053,13.));
#18996=CARTESIAN_POINT('Ctrl Pts',(19.5557680877664,1.66279554784111,13.));
#18997=CARTESIAN_POINT('Ctrl Pts',(19.5230842951169,1.66954412486476,13.));
#18998=CARTESIAN_POINT('Ctrl Pts',(19.4903963524289,1.67602787926304,13.));
#18999=CARTESIAN_POINT('Ctrl Pts',(19.4628617562097,1.68148945147165,13.));
#19000=CARTESIAN_POINT('Ctrl Pts',(19.4353241964729,1.68676485596096,13.));
#19001=CARTESIAN_POINT('Ctrl Pts',(19.4077853965428,1.69183425666145,13.));
#19002=CARTESIAN_POINT('Ctrl Pts',(19.3679337567804,1.6991702310336,13.));
#19003=CARTESIAN_POINT('Ctrl Pts',(19.3280794804744,1.70607400304418,13.));
#19004=CARTESIAN_POINT('Ctrl Pts',(19.2882303927414,1.71232694124141,13.));
#19005=CARTESIAN_POINT('Ctrl Pts',(19.2641520279257,1.71610520909267,13.));
#19006=CARTESIAN_POINT('Ctrl Pts',(19.2400756159532,1.71964237035168,13.));
#19007=CARTESIAN_POINT('Ctrl Pts',(19.2160028185096,1.72291205966735,13.));
#19008=CARTESIAN_POINT('Ctrl Pts',(19.1938009271707,1.72592763303679,13.));
#19009=CARTESIAN_POINT('Ctrl Pts',(19.1716021269002,1.72871436967202,13.));
#19010=CARTESIAN_POINT('Ctrl Pts',(19.1494073129856,1.7312973345182,13.));
#19011=CARTESIAN_POINT('Ctrl Pts',(19.1188760971263,1.73485046443309,13.));
#19012=CARTESIAN_POINT('Ctrl Pts',(19.0883522198778,1.73802530995667,13.));
#19013=CARTESIAN_POINT('Ctrl Pts',(19.0578380259466,1.74097263877354,13.));
#19014=CARTESIAN_POINT('Ctrl Pts',(19.0384792770224,1.74284247674769,13.));
#19015=CARTESIAN_POINT('Ctrl Pts',(19.0191244314898,1.74462241724651,13.));
#19016=CARTESIAN_POINT('Ctrl Pts',(18.9997750006083,1.74632097576622,13.));
#19017=CARTESIAN_POINT('Ctrl Pts',(18.9824097870281,1.74784535297679,13.));
#19018=CARTESIAN_POINT('Ctrl Pts',(18.9650489251703,1.74930491162225,13.));
#19019=CARTESIAN_POINT('Ctrl Pts',(18.9476944343168,1.75066513120051,13.));
#19020=CARTESIAN_POINT('Ctrl Pts',(18.9294514080686,1.75209499288178,13.));
#19021=CARTESIAN_POINT('Ctrl Pts',(18.9112154258052,1.75341524154102,13.));
#19022=CARTESIAN_POINT('Ctrl Pts',(18.8929901413736,1.75452347865357,13.));
#19023=CARTESIAN_POINT('Ctrl Pts',(18.8627179842696,1.75636425804473,13.));
#19024=CARTESIAN_POINT('Ctrl Pts',(18.8324756677938,1.75761169393965,13.));
#19025=CARTESIAN_POINT('Ctrl Pts',(18.8022820949853,1.75764008468142,13.));
#19026=CARTESIAN_POINT('Ctrl Pts',(18.78563228436,1.75765574034685,13.));
#19027=CARTESIAN_POINT('Ctrl Pts',(18.7689972916683,1.75729933637005,13.));
#19028=CARTESIAN_POINT('Ctrl Pts',(18.7523793043596,1.75649392367776,13.));
#19029=CARTESIAN_POINT('Ctrl Pts',(18.7388614288031,1.75583876199398,13.));
#19030=CARTESIAN_POINT('Ctrl Pts',(18.7253548001715,1.75488656240096,13.));
#19031=CARTESIAN_POINT('Ctrl Pts',(18.7118598491961,1.75362185428836,13.));
#19032=CARTESIAN_POINT('',(18.5778175999297,1.74105979901401,13.));
#19033=CARTESIAN_POINT('',(9.35592992459806,0.876810927144181,13.));
#19034=CARTESIAN_POINT('',(17.4952923049513,2.59023998199238,13.));
#19035=CARTESIAN_POINT('Origin',(18.4845093299966,2.73669706567396,13.));
#19036=CARTESIAN_POINT('Origin',(0.,0.,13.));
#19037=CARTESIAN_POINT('Origin',(0.,0.,13.));
#19038=CARTESIAN_POINT('Origin',(0.,0.,13.));
#19039=CARTESIAN_POINT('Origin',(0.,0.,13.));
#19040=CARTESIAN_POINT('Origin',(0.,0.,13.));
#19041=CARTESIAN_POINT('Origin',(0.,0.,13.));
#19042=CARTESIAN_POINT('Origin',(0.,0.,13.));
#19043=CARTESIAN_POINT('Origin',(0.,0.,13.));
#19044=CARTESIAN_POINT('Origin',(0.,0.,13.));
#19045=CARTESIAN_POINT('Origin',(0.,0.,13.));
#19046=CARTESIAN_POINT('Origin',(0.,0.,13.));
#19047=CARTESIAN_POINT('Origin',(0.,0.,13.));
#19048=CARTESIAN_POINT('Origin',(0.,0.,13.));
#19049=CARTESIAN_POINT('Origin',(0.,0.,13.));
#19050=CARTESIAN_POINT('Origin',(0.,0.,13.));
#19051=CARTESIAN_POINT('Origin',(0.,0.,13.));
#19052=CARTESIAN_POINT('Origin',(0.,0.,13.));
#19053=CARTESIAN_POINT('Origin',(0.,0.,13.));
#19054=CARTESIAN_POINT('Origin',(0.,0.,13.));
#19055=CARTESIAN_POINT('Origin',(0.,0.,0.));
#19056=CARTESIAN_POINT('',(17.4952923049513,2.59023998199238,0.));
#19057=CARTESIAN_POINT('Origin',(0.,0.,0.));
#19058=CARTESIAN_POINT('Origin',(0.,0.,0.));
#19059=CARTESIAN_POINT('Origin',(0.,0.,0.));
#19060=CARTESIAN_POINT('Origin',(0.,0.,0.));
#19061=CARTESIAN_POINT('Origin',(0.,0.,0.));
#19062=CARTESIAN_POINT('Origin',(0.,0.,0.));
#19063=CARTESIAN_POINT('Origin',(0.,0.,0.));
#19064=CARTESIAN_POINT('Origin',(0.,0.,0.));
#19065=CARTESIAN_POINT('Origin',(0.,0.,0.));
#19066=CARTESIAN_POINT('Origin',(0.,0.,0.));
#19067=CARTESIAN_POINT('Origin',(0.,0.,0.));
#19068=CARTESIAN_POINT('Origin',(0.,0.,0.));
#19069=CARTESIAN_POINT('Origin',(0.,0.,0.));
#19070=CARTESIAN_POINT('Origin',(0.,0.,0.));
#19071=CARTESIAN_POINT('Origin',(0.,0.,0.));
#19072=CARTESIAN_POINT('Origin',(0.,0.,0.));
#19073=CARTESIAN_POINT('Origin',(0.,0.,0.));
#19074=CARTESIAN_POINT('Origin',(0.,0.,0.));
#19075=CARTESIAN_POINT('Origin',(18.4845093299966,2.73669706567396,0.));
#19076=CARTESIAN_POINT('',(18.5778175999297,1.74105979901401,0.));
#19077=CARTESIAN_POINT('Origin',(18.7118598491961,1.75362185428836,0.));
#19078=CARTESIAN_POINT('',(18.7118598491961,1.75362185428836,0.));
#19079=CARTESIAN_POINT('Origin',(18.4845093299966,-2.73669706567396,0.));
#19080=CARTESIAN_POINT('',(18.5778175999297,-1.74105979901401,0.));
#19081=CARTESIAN_POINT('',(17.4952923049513,-2.59023998199238,0.));
#19082=CARTESIAN_POINT('Origin',(17.5988843254813,-1.64931697933718,0.));
#19083=CARTESIAN_POINT('',(18.7118598491961,-1.75362185428836,0.));
#19084=CARTESIAN_POINT('Ctrl Pts',(21.9890268624765,0.694764450219581,0.));
#19085=CARTESIAN_POINT('Ctrl Pts',(21.9890268624765,0.694764450219581,21.));
#19086=CARTESIAN_POINT('Ctrl Pts',(21.9799122315157,0.699924103234223,0.));
#19087=CARTESIAN_POINT('Ctrl Pts',(21.9799122315157,0.699924103234223,21.));
#19088=CARTESIAN_POINT('Ctrl Pts',(21.9616777523685,0.710218621843556,0.));
#19089=CARTESIAN_POINT('Ctrl Pts',(21.9616777523685,0.710218621843556,21.));
#19090=CARTESIAN_POINT('Ctrl Pts',(21.9343103819749,0.725586037496636,0.));
#19091=CARTESIAN_POINT('Ctrl Pts',(21.9343103819749,0.725586037496636,21.));
#19092=CARTESIAN_POINT('Ctrl Pts',(21.8977892409997,0.745927151109822,0.));
#19093=CARTESIAN_POINT('Ctrl Pts',(21.8977892409997,0.745927151109822,21.));
#19094=CARTESIAN_POINT('Ctrl Pts',(21.8520856039249,0.77110521325833,0.));
#19095=CARTESIAN_POINT('Ctrl Pts',(21.8520856039249,0.77110521325833,21.));
#19096=CARTESIAN_POINT('Ctrl Pts',(21.8063297959755,0.796034321106413,0.));
#19097=CARTESIAN_POINT('Ctrl Pts',(21.8063297959755,0.796034321106413,21.));
#19098=CARTESIAN_POINT('Ctrl Pts',(21.7605219769118,0.820713597934077,0.));
#19099=CARTESIAN_POINT('Ctrl Pts',(21.7605219769118,0.820713597934077,21.));
#19100=CARTESIAN_POINT('Ctrl Pts',(21.7146624809285,0.845141916726558,0.));
#19101=CARTESIAN_POINT('Ctrl Pts',(21.7146624809285,0.845141916726558,21.));
#19102=CARTESIAN_POINT('Ctrl Pts',(21.6687518829182,0.869317897714099,0.));
#19103=CARTESIAN_POINT('Ctrl Pts',(21.6687518829182,0.869317897714099,21.));
#19104=CARTESIAN_POINT('Ctrl Pts',(21.6227909401433,0.893239967513673,0.));
#19105=CARTESIAN_POINT('Ctrl Pts',(21.6227909401433,0.893239967513673,21.));
#19106=CARTESIAN_POINT('Ctrl Pts',(21.5767805209408,0.916906425150854,0.));
#19107=CARTESIAN_POINT('Ctrl Pts',(21.5767805209408,0.916906425150854,21.));
#19108=CARTESIAN_POINT('Ctrl Pts',(21.5307215366685,0.94031550952515,0.));
#19109=CARTESIAN_POINT('Ctrl Pts',(21.5307215366685,0.94031550952515,21.));
#19110=CARTESIAN_POINT('Ctrl Pts',(21.4846148770804,0.963465462815772,0.));
#19111=CARTESIAN_POINT('Ctrl Pts',(21.4846148770804,0.963465462815772,21.));
#19112=CARTESIAN_POINT('Ctrl Pts',(21.4384613333266,0.986354611081135,0.));
#19113=CARTESIAN_POINT('Ctrl Pts',(21.4384613333266,0.986354611081135,21.));
#19114=CARTESIAN_POINT('Ctrl Pts',(21.3922616124166,1.00898133629988,0.));
#19115=CARTESIAN_POINT('Ctrl Pts',(21.3922616124166,1.00898133629988,21.));
#19116=CARTESIAN_POINT('Ctrl Pts',(21.3460163737343,1.03134402396953,0.));
#19117=CARTESIAN_POINT('Ctrl Pts',(21.3460163737343,1.03134402396953,21.));
#19118=CARTESIAN_POINT('Ctrl Pts',(21.2997262593683,1.05344101900192,0.));
#19119=CARTESIAN_POINT('Ctrl Pts',(21.2997262593683,1.05344101900192,21.));
#19120=CARTESIAN_POINT('Ctrl Pts',(21.2533919248553,1.07527058431887,0.));
#19121=CARTESIAN_POINT('Ctrl Pts',(21.2533919248553,1.07527058431887,21.));
#19122=CARTESIAN_POINT('Ctrl Pts',(21.2070140764156,1.09683084929266,0.));
#19123=CARTESIAN_POINT('Ctrl Pts',(21.2070140764156,1.09683084929266,21.));
#19124=CARTESIAN_POINT('Ctrl Pts',(21.1605934684164,1.11811982787746,0.));
#19125=CARTESIAN_POINT('Ctrl Pts',(21.1605934684164,1.11811982787746,21.));
#19126=CARTESIAN_POINT('Ctrl Pts',(21.1141308858087,1.13913546246555,0.));
#19127=CARTESIAN_POINT('Ctrl Pts',(21.1141308858087,1.13913546246555,21.));
#19128=CARTESIAN_POINT('Ctrl Pts',(21.0676271313238,1.15987566445807,0.));
#19129=CARTESIAN_POINT('Ctrl Pts',(21.0676271313238,1.15987566445807,21.));
#19130=CARTESIAN_POINT('Ctrl Pts',(21.0210830121673,1.18033835060894,0.));
#19131=CARTESIAN_POINT('Ctrl Pts',(21.0210830121673,1.18033835060894,21.));
#19132=CARTESIAN_POINT('Ctrl Pts',(20.9744993243732,1.20052150219503,0.));
#19133=CARTESIAN_POINT('Ctrl Pts',(20.9744993243732,1.20052150219503,21.));
#19134=CARTESIAN_POINT('Ctrl Pts',(20.9278768531175,1.22042312071096,0.));
#19135=CARTESIAN_POINT('Ctrl Pts',(20.9278768531175,1.22042312071096,21.));
#19136=CARTESIAN_POINT('Ctrl Pts',(20.881216381382,1.24004113517905,0.));
#19137=CARTESIAN_POINT('Ctrl Pts',(20.881216381382,1.24004113517905,21.));
#19138=CARTESIAN_POINT('Ctrl Pts',(20.83451869657,1.25937332001005,0.));
#19139=CARTESIAN_POINT('Ctrl Pts',(20.83451869657,1.25937332001005,21.));
#19140=CARTESIAN_POINT('Ctrl Pts',(20.7877845975367,1.27841722479262,0.));
#19141=CARTESIAN_POINT('Ctrl Pts',(20.7877845975367,1.27841722479262,21.));
#19142=CARTESIAN_POINT('Ctrl Pts',(20.7410149035348,1.2971700649115,0.));
#19143=CARTESIAN_POINT('Ctrl Pts',(20.7410149035348,1.2971700649115,21.));
#19144=CARTESIAN_POINT('Ctrl Pts',(20.694210454218,1.31562879653596,0.));
#19145=CARTESIAN_POINT('Ctrl Pts',(20.694210454218,1.31562879653596,21.));
#19146=CARTESIAN_POINT('Ctrl Pts',(20.6473721041685,1.3337902972259,0.));
#19147=CARTESIAN_POINT('Ctrl Pts',(20.6473721041685,1.3337902972259,21.));
#19148=CARTESIAN_POINT('Ctrl Pts',(20.6005007190809,1.35165153211253,0.));
#19149=CARTESIAN_POINT('Ctrl Pts',(20.6005007190809,1.35165153211253,21.));
#19150=CARTESIAN_POINT('Ctrl Pts',(20.5535971721246,1.36920969340018,0.));
#19151=CARTESIAN_POINT('Ctrl Pts',(20.5535971721246,1.36920969340018,21.));
#19152=CARTESIAN_POINT('Ctrl Pts',(20.5066623390132,1.38646244026049,0.));
#19153=CARTESIAN_POINT('Ctrl Pts',(20.5066623390132,1.38646244026049,21.));
#19154=CARTESIAN_POINT('Ctrl Pts',(20.4596971004275,1.40340771617024,0.));
#19155=CARTESIAN_POINT('Ctrl Pts',(20.4596971004275,1.40340771617024,21.));
#19156=CARTESIAN_POINT('Ctrl Pts',(20.4127023494155,1.4200432946371,0.));
#19157=CARTESIAN_POINT('Ctrl Pts',(20.4127023494155,1.4200432946371,21.));
#19158=CARTESIAN_POINT('Ctrl Pts',(20.3656789980171,1.43636637152782,0.));
#19159=CARTESIAN_POINT('Ctrl Pts',(20.3656789980171,1.43636637152782,21.));
#19160=CARTESIAN_POINT('Ctrl Pts',(20.3186279833818,1.45237321894404,0.));
#19161=CARTESIAN_POINT('Ctrl Pts',(20.3186279833818,1.45237321894404,21.));
#19162=CARTESIAN_POINT('Ctrl Pts',(20.2715502770004,1.46805861808021,0.));
#19163=CARTESIAN_POINT('Ctrl Pts',(20.2715502770004,1.46805861808021,21.));
#19164=CARTESIAN_POINT('Ctrl Pts',(20.224446881308,1.48341623961914,0.));
#19165=CARTESIAN_POINT('Ctrl Pts',(20.224446881308,1.48341623961914,21.));
#19166=CARTESIAN_POINT('Ctrl Pts',(20.1773188177942,1.49843965844502,0.));
#19167=CARTESIAN_POINT('Ctrl Pts',(20.1773188177942,1.49843965844502,21.));
#19168=CARTESIAN_POINT('Ctrl Pts',(20.1301671167606,1.51312326913583,0.));
#19169=CARTESIAN_POINT('Ctrl Pts',(20.1301671167606,1.51312326913583,21.));
#19170=CARTESIAN_POINT('Ctrl Pts',(20.0829928089241,1.52746305716964,0.));
#19171=CARTESIAN_POINT('Ctrl Pts',(20.0829928089241,1.52746305716964,21.));
#19172=CARTESIAN_POINT('Ctrl Pts',(20.0357969106526,1.54145790302918,0.));
#19173=CARTESIAN_POINT('Ctrl Pts',(20.0357969106526,1.54145790302918,21.));
#19174=CARTESIAN_POINT('Ctrl Pts',(19.9885804375096,1.55510860515913,0.));
#19175=CARTESIAN_POINT('Ctrl Pts',(19.9885804375096,1.55510860515913,21.));
#19176=CARTESIAN_POINT('Ctrl Pts',(19.9413444362352,1.56841542790452,0.));
#19177=CARTESIAN_POINT('Ctrl Pts',(19.9413444362352,1.56841542790452,21.));
#19178=CARTESIAN_POINT('Ctrl Pts',(19.8940900137801,1.58137589158952,0.));
#19179=CARTESIAN_POINT('Ctrl Pts',(19.8940900137801,1.58137589158952,21.));
#19180=CARTESIAN_POINT('Ctrl Pts',(19.8468183626037,1.59398289700559,0.));
#19181=CARTESIAN_POINT('Ctrl Pts',(19.8468183626037,1.59398289700559,21.));
#19182=CARTESIAN_POINT('Ctrl Pts',(19.7995308006834,1.60622162219699,0.));
#19183=CARTESIAN_POINT('Ctrl Pts',(19.7995308006834,1.60622162219699,21.));
#19184=CARTESIAN_POINT('Ctrl Pts',(19.7522287462982,1.61807191996834,0.));
#19185=CARTESIAN_POINT('Ctrl Pts',(19.7522287462982,1.61807191996834,21.));
#19186=CARTESIAN_POINT('Ctrl Pts',(19.7049136553525,1.62951389038422,0.));
#19187=CARTESIAN_POINT('Ctrl Pts',(19.7049136553525,1.62951389038422,21.));
#19188=CARTESIAN_POINT('Ctrl Pts',(19.6575869645839,1.64053294677821,0.));
#19189=CARTESIAN_POINT('Ctrl Pts',(19.6575869645839,1.64053294677821,21.));
#19190=CARTESIAN_POINT('Ctrl Pts',(19.6102500448855,1.65112409599283,0.));
#19191=CARTESIAN_POINT('Ctrl Pts',(19.6102500448855,1.65112409599283,21.));
#19192=CARTESIAN_POINT('Ctrl Pts',(19.5629041190868,1.66129908621006,0.));
#19193=CARTESIAN_POINT('Ctrl Pts',(19.5629041190868,1.66129908621006,21.));
#19194=CARTESIAN_POINT('Ctrl Pts',(19.5155503513712,1.67107974760949,0.));
#19195=CARTESIAN_POINT('Ctrl Pts',(19.5155503513712,1.67107974760949,21.));
#19196=CARTESIAN_POINT('Ctrl Pts',(19.4681900187091,1.68048476382294,0.));
#19197=CARTESIAN_POINT('Ctrl Pts',(19.4681900187091,1.68048476382294,21.));
#19198=CARTESIAN_POINT('Ctrl Pts',(19.4208246682917,1.68951753233571,0.));
#19199=CARTESIAN_POINT('Ctrl Pts',(19.4208246682917,1.68951753233571,21.));
#19200=CARTESIAN_POINT('Ctrl Pts',(19.3734562555057,1.69815571801252,0.));
#19201=CARTESIAN_POINT('Ctrl Pts',(19.3734562555057,1.69815571801252,21.));
#19202=CARTESIAN_POINT('Ctrl Pts',(19.3260873558094,1.70633457265124,0.));
#19203=CARTESIAN_POINT('Ctrl Pts',(19.3260873558094,1.70633457265124,21.));
#19204=CARTESIAN_POINT('Ctrl Pts',(19.2787209722437,1.71396454346262,0.));
#19205=CARTESIAN_POINT('Ctrl Pts',(19.2787209722437,1.71396454346262,21.));
#19206=CARTESIAN_POINT('Ctrl Pts',(19.2313602042899,1.72096104670234,0.));
#19207=CARTESIAN_POINT('Ctrl Pts',(19.2313602042899,1.72096104670234,21.));
#19208=CARTESIAN_POINT('Ctrl Pts',(19.1840079312107,1.72727220327098,0.));
#19209=CARTESIAN_POINT('Ctrl Pts',(19.1840079312107,1.72727220327098,21.));
#19210=CARTESIAN_POINT('Ctrl Pts',(19.1366665585833,1.73290313712353,0.));
#19211=CARTESIAN_POINT('Ctrl Pts',(19.1366665585833,1.73290313712353,21.));
#19212=CARTESIAN_POINT('Ctrl Pts',(19.0893375576541,1.7379530116984,0.));
#19213=CARTESIAN_POINT('Ctrl Pts',(19.0893375576541,1.7379530116984,21.));
#19214=CARTESIAN_POINT('Ctrl Pts',(19.0420224296189,1.74256297552949,0.));
#19215=CARTESIAN_POINT('Ctrl Pts',(19.0420224296189,1.74256297552949,21.));
#19216=CARTESIAN_POINT('Ctrl Pts',(18.9947239970259,1.74684309825012,0.));
#19217=CARTESIAN_POINT('Ctrl Pts',(18.9947239970259,1.74684309825012,21.));
#19218=CARTESIAN_POINT('Ctrl Pts',(18.947447637865,1.75080409924533,0.));
#19219=CARTESIAN_POINT('Ctrl Pts',(18.947447637865,1.75080409924533,21.));
#19220=CARTESIAN_POINT('Ctrl Pts',(18.9002024267872,1.75429229572775,0.));
#19221=CARTESIAN_POINT('Ctrl Pts',(18.9002024267872,1.75429229572775,21.));
#19222=CARTESIAN_POINT('Ctrl Pts',(18.8530026395886,1.75690876962597,0.));
#19223=CARTESIAN_POINT('Ctrl Pts',(18.8530026395886,1.75690876962597,21.));
#19224=CARTESIAN_POINT('Ctrl Pts',(18.8058650094752,1.7581175236483,0.));
#19225=CARTESIAN_POINT('Ctrl Pts',(18.8058650094752,1.7581175236483,21.));
#19226=CARTESIAN_POINT('Ctrl Pts',(18.7682173836138,1.75752447968136,0.));
#19227=CARTESIAN_POINT('Ctrl Pts',(18.7682173836138,1.75752447968136,21.));
#19228=CARTESIAN_POINT('Ctrl Pts',(18.7400222442427,1.75601041697575,0.));
#19229=CARTESIAN_POINT('Ctrl Pts',(18.7400222442427,1.75601041697575,21.));
#19230=CARTESIAN_POINT('Ctrl Pts',(18.7212441956871,1.75450132833464,0.));
#19231=CARTESIAN_POINT('Ctrl Pts',(18.7212441956871,1.75450132833464,21.));
#19232=CARTESIAN_POINT('Ctrl Pts',(18.7118598491961,1.75362185428836,0.));
#19233=CARTESIAN_POINT('Ctrl Pts',(18.7118598491961,1.75362185428836,21.));
#19234=CARTESIAN_POINT('',(21.9890268624765,0.694764450219646,0.));
#19235=CARTESIAN_POINT('Origin',(5.6665783176868E-12,0.,0.));
#19236=CARTESIAN_POINT('',(21.9890268624765,-0.694764450219581,0.));
#19237=CARTESIAN_POINT('Ctrl Pts',(18.7118598491961,-1.75362185428836,0.));
#19238=CARTESIAN_POINT('Ctrl Pts',(18.7118598491961,-1.75362185428836,21.));
#19239=CARTESIAN_POINT('Ctrl Pts',(18.7212441956871,-1.75450132833464,0.));
#19240=CARTESIAN_POINT('Ctrl Pts',(18.7212441956871,-1.75450132833464,21.));
#19241=CARTESIAN_POINT('Ctrl Pts',(18.7400222442427,-1.75601041697575,0.));
#19242=CARTESIAN_POINT('Ctrl Pts',(18.7400222442427,-1.75601041697575,21.));
#19243=CARTESIAN_POINT('Ctrl Pts',(18.7682173836138,-1.75752447968136,0.));
#19244=CARTESIAN_POINT('Ctrl Pts',(18.7682173836138,-1.75752447968136,21.));
#19245=CARTESIAN_POINT('Ctrl Pts',(18.8058650094752,-1.7581175236483,0.));
#19246=CARTESIAN_POINT('Ctrl Pts',(18.8058650094752,-1.7581175236483,21.));
#19247=CARTESIAN_POINT('Ctrl Pts',(18.8530026395886,-1.75690876962597,0.));
#19248=CARTESIAN_POINT('Ctrl Pts',(18.8530026395886,-1.75690876962597,21.));
#19249=CARTESIAN_POINT('Ctrl Pts',(18.9002024267872,-1.75429229572775,0.));
#19250=CARTESIAN_POINT('Ctrl Pts',(18.9002024267872,-1.75429229572775,21.));
#19251=CARTESIAN_POINT('Ctrl Pts',(18.947447637865,-1.75080409924533,0.));
#19252=CARTESIAN_POINT('Ctrl Pts',(18.947447637865,-1.75080409924533,21.));
#19253=CARTESIAN_POINT('Ctrl Pts',(18.9947239970259,-1.74684309825012,0.));
#19254=CARTESIAN_POINT('Ctrl Pts',(18.9947239970259,-1.74684309825012,21.));
#19255=CARTESIAN_POINT('Ctrl Pts',(19.0420224296189,-1.74256297552949,0.));
#19256=CARTESIAN_POINT('Ctrl Pts',(19.0420224296189,-1.74256297552949,21.));
#19257=CARTESIAN_POINT('Ctrl Pts',(19.0893375576541,-1.7379530116984,0.));
#19258=CARTESIAN_POINT('Ctrl Pts',(19.0893375576541,-1.7379530116984,21.));
#19259=CARTESIAN_POINT('Ctrl Pts',(19.1366665585833,-1.73290313712353,0.));
#19260=CARTESIAN_POINT('Ctrl Pts',(19.1366665585833,-1.73290313712353,21.));
#19261=CARTESIAN_POINT('Ctrl Pts',(19.1840079312107,-1.72727220327098,0.));
#19262=CARTESIAN_POINT('Ctrl Pts',(19.1840079312107,-1.72727220327098,21.));
#19263=CARTESIAN_POINT('Ctrl Pts',(19.2313602042899,-1.72096104670234,0.));
#19264=CARTESIAN_POINT('Ctrl Pts',(19.2313602042899,-1.72096104670234,21.));
#19265=CARTESIAN_POINT('Ctrl Pts',(19.2787209722437,-1.71396454346262,0.));
#19266=CARTESIAN_POINT('Ctrl Pts',(19.2787209722437,-1.71396454346262,21.));
#19267=CARTESIAN_POINT('Ctrl Pts',(19.3260873558094,-1.70633457265124,0.));
#19268=CARTESIAN_POINT('Ctrl Pts',(19.3260873558094,-1.70633457265124,21.));
#19269=CARTESIAN_POINT('Ctrl Pts',(19.3734562555057,-1.69815571801252,0.));
#19270=CARTESIAN_POINT('Ctrl Pts',(19.3734562555057,-1.69815571801252,21.));
#19271=CARTESIAN_POINT('Ctrl Pts',(19.4208246682917,-1.68951753233571,0.));
#19272=CARTESIAN_POINT('Ctrl Pts',(19.4208246682917,-1.68951753233571,21.));
#19273=CARTESIAN_POINT('Ctrl Pts',(19.4681900187091,-1.68048476382294,0.));
#19274=CARTESIAN_POINT('Ctrl Pts',(19.4681900187091,-1.68048476382294,21.));
#19275=CARTESIAN_POINT('Ctrl Pts',(19.5155503513712,-1.67107974760949,0.));
#19276=CARTESIAN_POINT('Ctrl Pts',(19.5155503513712,-1.67107974760949,21.));
#19277=CARTESIAN_POINT('Ctrl Pts',(19.5629041190868,-1.66129908621006,0.));
#19278=CARTESIAN_POINT('Ctrl Pts',(19.5629041190868,-1.66129908621006,21.));
#19279=CARTESIAN_POINT('Ctrl Pts',(19.6102500448855,-1.65112409599283,0.));
#19280=CARTESIAN_POINT('Ctrl Pts',(19.6102500448855,-1.65112409599283,21.));
#19281=CARTESIAN_POINT('Ctrl Pts',(19.6575869645839,-1.64053294677821,0.));
#19282=CARTESIAN_POINT('Ctrl Pts',(19.6575869645839,-1.64053294677821,21.));
#19283=CARTESIAN_POINT('Ctrl Pts',(19.7049136553525,-1.62951389038422,0.));
#19284=CARTESIAN_POINT('Ctrl Pts',(19.7049136553525,-1.62951389038422,21.));
#19285=CARTESIAN_POINT('Ctrl Pts',(19.7522287462982,-1.61807191996834,0.));
#19286=CARTESIAN_POINT('Ctrl Pts',(19.7522287462982,-1.61807191996834,21.));
#19287=CARTESIAN_POINT('Ctrl Pts',(19.7995308006834,-1.60622162219699,0.));
#19288=CARTESIAN_POINT('Ctrl Pts',(19.7995308006834,-1.60622162219699,21.));
#19289=CARTESIAN_POINT('Ctrl Pts',(19.8468183626037,-1.59398289700559,0.));
#19290=CARTESIAN_POINT('Ctrl Pts',(19.8468183626037,-1.59398289700559,21.));
#19291=CARTESIAN_POINT('Ctrl Pts',(19.8940900137801,-1.58137589158952,0.));
#19292=CARTESIAN_POINT('Ctrl Pts',(19.8940900137801,-1.58137589158952,21.));
#19293=CARTESIAN_POINT('Ctrl Pts',(19.9413444362352,-1.56841542790452,0.));
#19294=CARTESIAN_POINT('Ctrl Pts',(19.9413444362352,-1.56841542790452,21.));
#19295=CARTESIAN_POINT('Ctrl Pts',(19.9885804375096,-1.55510860515913,0.));
#19296=CARTESIAN_POINT('Ctrl Pts',(19.9885804375096,-1.55510860515913,21.));
#19297=CARTESIAN_POINT('Ctrl Pts',(20.0357969106526,-1.54145790302918,0.));
#19298=CARTESIAN_POINT('Ctrl Pts',(20.0357969106526,-1.54145790302918,21.));
#19299=CARTESIAN_POINT('Ctrl Pts',(20.0829928089241,-1.52746305716964,0.));
#19300=CARTESIAN_POINT('Ctrl Pts',(20.0829928089241,-1.52746305716964,21.));
#19301=CARTESIAN_POINT('Ctrl Pts',(20.1301671167606,-1.51312326913583,0.));
#19302=CARTESIAN_POINT('Ctrl Pts',(20.1301671167606,-1.51312326913583,21.));
#19303=CARTESIAN_POINT('Ctrl Pts',(20.1773188177942,-1.49843965844502,0.));
#19304=CARTESIAN_POINT('Ctrl Pts',(20.1773188177942,-1.49843965844502,21.));
#19305=CARTESIAN_POINT('Ctrl Pts',(20.224446881308,-1.48341623961914,0.));
#19306=CARTESIAN_POINT('Ctrl Pts',(20.224446881308,-1.48341623961914,21.));
#19307=CARTESIAN_POINT('Ctrl Pts',(20.2715502770004,-1.46805861808021,0.));
#19308=CARTESIAN_POINT('Ctrl Pts',(20.2715502770004,-1.46805861808021,21.));
#19309=CARTESIAN_POINT('Ctrl Pts',(20.3186279833818,-1.45237321894404,0.));
#19310=CARTESIAN_POINT('Ctrl Pts',(20.3186279833818,-1.45237321894404,21.));
#19311=CARTESIAN_POINT('Ctrl Pts',(20.3656789980171,-1.43636637152782,0.));
#19312=CARTESIAN_POINT('Ctrl Pts',(20.3656789980171,-1.43636637152782,21.));
#19313=CARTESIAN_POINT('Ctrl Pts',(20.4127023494155,-1.4200432946371,0.));
#19314=CARTESIAN_POINT('Ctrl Pts',(20.4127023494155,-1.4200432946371,21.));
#19315=CARTESIAN_POINT('Ctrl Pts',(20.4596971004275,-1.40340771617024,0.));
#19316=CARTESIAN_POINT('Ctrl Pts',(20.4596971004275,-1.40340771617024,21.));
#19317=CARTESIAN_POINT('Ctrl Pts',(20.5066623390132,-1.38646244026049,0.));
#19318=CARTESIAN_POINT('Ctrl Pts',(20.5066623390132,-1.38646244026049,21.));
#19319=CARTESIAN_POINT('Ctrl Pts',(20.5535971721246,-1.36920969340018,0.));
#19320=CARTESIAN_POINT('Ctrl Pts',(20.5535971721246,-1.36920969340018,21.));
#19321=CARTESIAN_POINT('Ctrl Pts',(20.6005007190809,-1.35165153211253,0.));
#19322=CARTESIAN_POINT('Ctrl Pts',(20.6005007190809,-1.35165153211253,21.));
#19323=CARTESIAN_POINT('Ctrl Pts',(20.6473721041685,-1.3337902972259,0.));
#19324=CARTESIAN_POINT('Ctrl Pts',(20.6473721041685,-1.3337902972259,21.));
#19325=CARTESIAN_POINT('Ctrl Pts',(20.694210454218,-1.31562879653596,0.));
#19326=CARTESIAN_POINT('Ctrl Pts',(20.694210454218,-1.31562879653596,21.));
#19327=CARTESIAN_POINT('Ctrl Pts',(20.7410149035348,-1.2971700649115,0.));
#19328=CARTESIAN_POINT('Ctrl Pts',(20.7410149035348,-1.2971700649115,21.));
#19329=CARTESIAN_POINT('Ctrl Pts',(20.7877845975367,-1.27841722479262,0.));
#19330=CARTESIAN_POINT('Ctrl Pts',(20.7877845975367,-1.27841722479262,21.));
#19331=CARTESIAN_POINT('Ctrl Pts',(20.83451869657,-1.25937332001005,0.));
#19332=CARTESIAN_POINT('Ctrl Pts',(20.83451869657,-1.25937332001005,21.));
#19333=CARTESIAN_POINT('Ctrl Pts',(20.881216381382,-1.24004113517905,0.));
#19334=CARTESIAN_POINT('Ctrl Pts',(20.881216381382,-1.24004113517905,21.));
#19335=CARTESIAN_POINT('Ctrl Pts',(20.9278768531175,-1.22042312071096,0.));
#19336=CARTESIAN_POINT('Ctrl Pts',(20.9278768531175,-1.22042312071096,21.));
#19337=CARTESIAN_POINT('Ctrl Pts',(20.9744993243732,-1.20052150219503,0.));
#19338=CARTESIAN_POINT('Ctrl Pts',(20.9744993243732,-1.20052150219503,21.));
#19339=CARTESIAN_POINT('Ctrl Pts',(21.0210830121673,-1.18033835060894,0.));
#19340=CARTESIAN_POINT('Ctrl Pts',(21.0210830121673,-1.18033835060894,21.));
#19341=CARTESIAN_POINT('Ctrl Pts',(21.0676271313238,-1.15987566445807,0.));
#19342=CARTESIAN_POINT('Ctrl Pts',(21.0676271313238,-1.15987566445807,21.));
#19343=CARTESIAN_POINT('Ctrl Pts',(21.1141308858087,-1.13913546246555,0.));
#19344=CARTESIAN_POINT('Ctrl Pts',(21.1141308858087,-1.13913546246555,21.));
#19345=CARTESIAN_POINT('Ctrl Pts',(21.1605934684164,-1.11811982787746,0.));
#19346=CARTESIAN_POINT('Ctrl Pts',(21.1605934684164,-1.11811982787746,21.));
#19347=CARTESIAN_POINT('Ctrl Pts',(21.2070140764156,-1.09683084929266,0.));
#19348=CARTESIAN_POINT('Ctrl Pts',(21.2070140764156,-1.09683084929266,21.));
#19349=CARTESIAN_POINT('Ctrl Pts',(21.2533919248553,-1.07527058431887,0.));
#19350=CARTESIAN_POINT('Ctrl Pts',(21.2533919248553,-1.07527058431887,21.));
#19351=CARTESIAN_POINT('Ctrl Pts',(21.2997262593683,-1.05344101900192,0.));
#19352=CARTESIAN_POINT('Ctrl Pts',(21.2997262593683,-1.05344101900192,21.));
#19353=CARTESIAN_POINT('Ctrl Pts',(21.3460163737343,-1.03134402396953,0.));
#19354=CARTESIAN_POINT('Ctrl Pts',(21.3460163737343,-1.03134402396953,21.));
#19355=CARTESIAN_POINT('Ctrl Pts',(21.3922616124166,-1.00898133629988,0.));
#19356=CARTESIAN_POINT('Ctrl Pts',(21.3922616124166,-1.00898133629988,21.));
#19357=CARTESIAN_POINT('Ctrl Pts',(21.4384613333266,-0.986354611081135,
0.));
#19358=CARTESIAN_POINT('Ctrl Pts',(21.4384613333266,-0.986354611081135,
21.));
#19359=CARTESIAN_POINT('Ctrl Pts',(21.4846148770804,-0.963465462815772,
0.));
#19360=CARTESIAN_POINT('Ctrl Pts',(21.4846148770804,-0.963465462815772,
21.));
#19361=CARTESIAN_POINT('Ctrl Pts',(21.5307215366685,-0.94031550952515,0.));
#19362=CARTESIAN_POINT('Ctrl Pts',(21.5307215366685,-0.94031550952515,21.));
#19363=CARTESIAN_POINT('Ctrl Pts',(21.5767805209408,-0.916906425150854,
0.));
#19364=CARTESIAN_POINT('Ctrl Pts',(21.5767805209408,-0.916906425150854,
21.));
#19365=CARTESIAN_POINT('Ctrl Pts',(21.6227909401433,-0.893239967513673,
0.));
#19366=CARTESIAN_POINT('Ctrl Pts',(21.6227909401433,-0.893239967513673,
21.));
#19367=CARTESIAN_POINT('Ctrl Pts',(21.6687518829182,-0.869317897714099,
0.));
#19368=CARTESIAN_POINT('Ctrl Pts',(21.6687518829182,-0.869317897714099,
21.));
#19369=CARTESIAN_POINT('Ctrl Pts',(21.7146624809285,-0.845141916726558,
0.));
#19370=CARTESIAN_POINT('Ctrl Pts',(21.7146624809285,-0.845141916726558,
21.));
#19371=CARTESIAN_POINT('Ctrl Pts',(21.7605219769118,-0.820713597934077,
0.));
#19372=CARTESIAN_POINT('Ctrl Pts',(21.7605219769118,-0.820713597934077,
21.));
#19373=CARTESIAN_POINT('Ctrl Pts',(21.8063297959755,-0.796034321106413,
0.));
#19374=CARTESIAN_POINT('Ctrl Pts',(21.8063297959755,-0.796034321106413,
21.));
#19375=CARTESIAN_POINT('Ctrl Pts',(21.8520856039249,-0.77110521325833,0.));
#19376=CARTESIAN_POINT('Ctrl Pts',(21.8520856039249,-0.77110521325833,21.));
#19377=CARTESIAN_POINT('Ctrl Pts',(21.8977892409997,-0.745927151109822,
0.));
#19378=CARTESIAN_POINT('Ctrl Pts',(21.8977892409997,-0.745927151109822,
21.));
#19379=CARTESIAN_POINT('Ctrl Pts',(21.9343103819749,-0.725586037496636,
0.));
#19380=CARTESIAN_POINT('Ctrl Pts',(21.9343103819749,-0.725586037496636,
21.));
#19381=CARTESIAN_POINT('Ctrl Pts',(21.9616777523685,-0.710218621843556,
0.));
#19382=CARTESIAN_POINT('Ctrl Pts',(21.9616777523685,-0.710218621843556,
21.));
#19383=CARTESIAN_POINT('Ctrl Pts',(21.9799122315157,-0.699924103234223,
0.));
#19384=CARTESIAN_POINT('Ctrl Pts',(21.9799122315157,-0.699924103234223,
21.));
#19385=CARTESIAN_POINT('Ctrl Pts',(21.9890268624765,-0.694764450219581,
0.));
#19386=CARTESIAN_POINT('Ctrl Pts',(21.9890268624765,-0.694764450219581,
21.));
#19387=CARTESIAN_POINT('Origin',(0.,0.,0.));
#19862=UNCERTAINTY_MEASURE_WITH_UNIT(LENGTH_MEASURE(0.01),#19879,
'DISTANCE_ACCURACY_VALUE',
'Maximum model space distance between geometric entities at asserted c
onnectivities');
#19869=UNCERTAINTY_MEASURE_WITH_UNIT(LENGTH_MEASURE(0.01),#19879,
'DISTANCE_ACCURACY_VALUE',
'Maximum model space distance between geometric entities at asserted c
onnectivities');
#19871=(
GEOMETRIC_REPRESENTATION_CONTEXT(3)
GLOBAL_UNCERTAINTY_ASSIGNED_CONTEXT((#19862))
GLOBAL_UNIT_ASSIGNED_CONTEXT((#19879,#19881,#19882))
REPRESENTATION_CONTEXT('','3D')
);
#19878=(
GEOMETRIC_REPRESENTATION_CONTEXT(3)
GLOBAL_UNCERTAINTY_ASSIGNED_CONTEXT((#19869))
GLOBAL_UNIT_ASSIGNED_CONTEXT((#19879,#19881,#19882))
REPRESENTATION_CONTEXT('','3D')
);
#19879=(
LENGTH_UNIT()
NAMED_UNIT(*)
SI_UNIT(.MILLI.,.METRE.)
);
#19881=(
NAMED_UNIT(*)
PLANE_ANGLE_UNIT()
SI_UNIT($,.RADIAN.)
);
#19882=(
NAMED_UNIT(*)
SI_UNIT($,.STERADIAN.)
SOLID_ANGLE_UNIT()
);
#19884=SHAPE_DEFINITION_REPRESENTATION(#19892,#19907);
#19892=PRODUCT_DEFINITION_SHAPE('',$,#19916);
#19907=SHAPE_REPRESENTATION('',(#4911),#19871);
#19914=PRODUCT_DEFINITION_CONTEXT('part definition',#19940,'design');
#19916=PRODUCT_DEFINITION('Gear','Gear',#19924,#19914);
#19924=PRODUCT_DEFINITION_FORMATION('',$,#19943);
#19940=APPLICATION_CONTEXT(
'Core Data for Automotive Mechanical Design Process');
#19941=PRODUCT_CONTEXT('part definition',#19940,'mechanical');
#19943=PRODUCT('Gear','Gear',
'Spur Gear; Module: 2.0; Num Teeth: 20; Pressure Angle: 20.0; Backlash
: 0.00 mm',(#19941));
#19951=PRESENTATION_STYLE_ASSIGNMENT((#19957));
#19957=SURFACE_STYLE_USAGE(.BOTH.,#19963);
#19963=SURFACE_SIDE_STYLE('',(#19969));
#19969=SURFACE_STYLE_FILL_AREA(#19975);
#19975=FILL_AREA_STYLE('Opaque(203,203,203)',(#19981));
#19981=FILL_AREA_STYLE_COLOUR('Opaque(203,203,203)',#19987);
#19987=COLOUR_RGB('Opaque(203,203,203)', 0.09019608, 0.27058824, 0.51372549);
ENDSEC;
END-ISO-10303-21;
